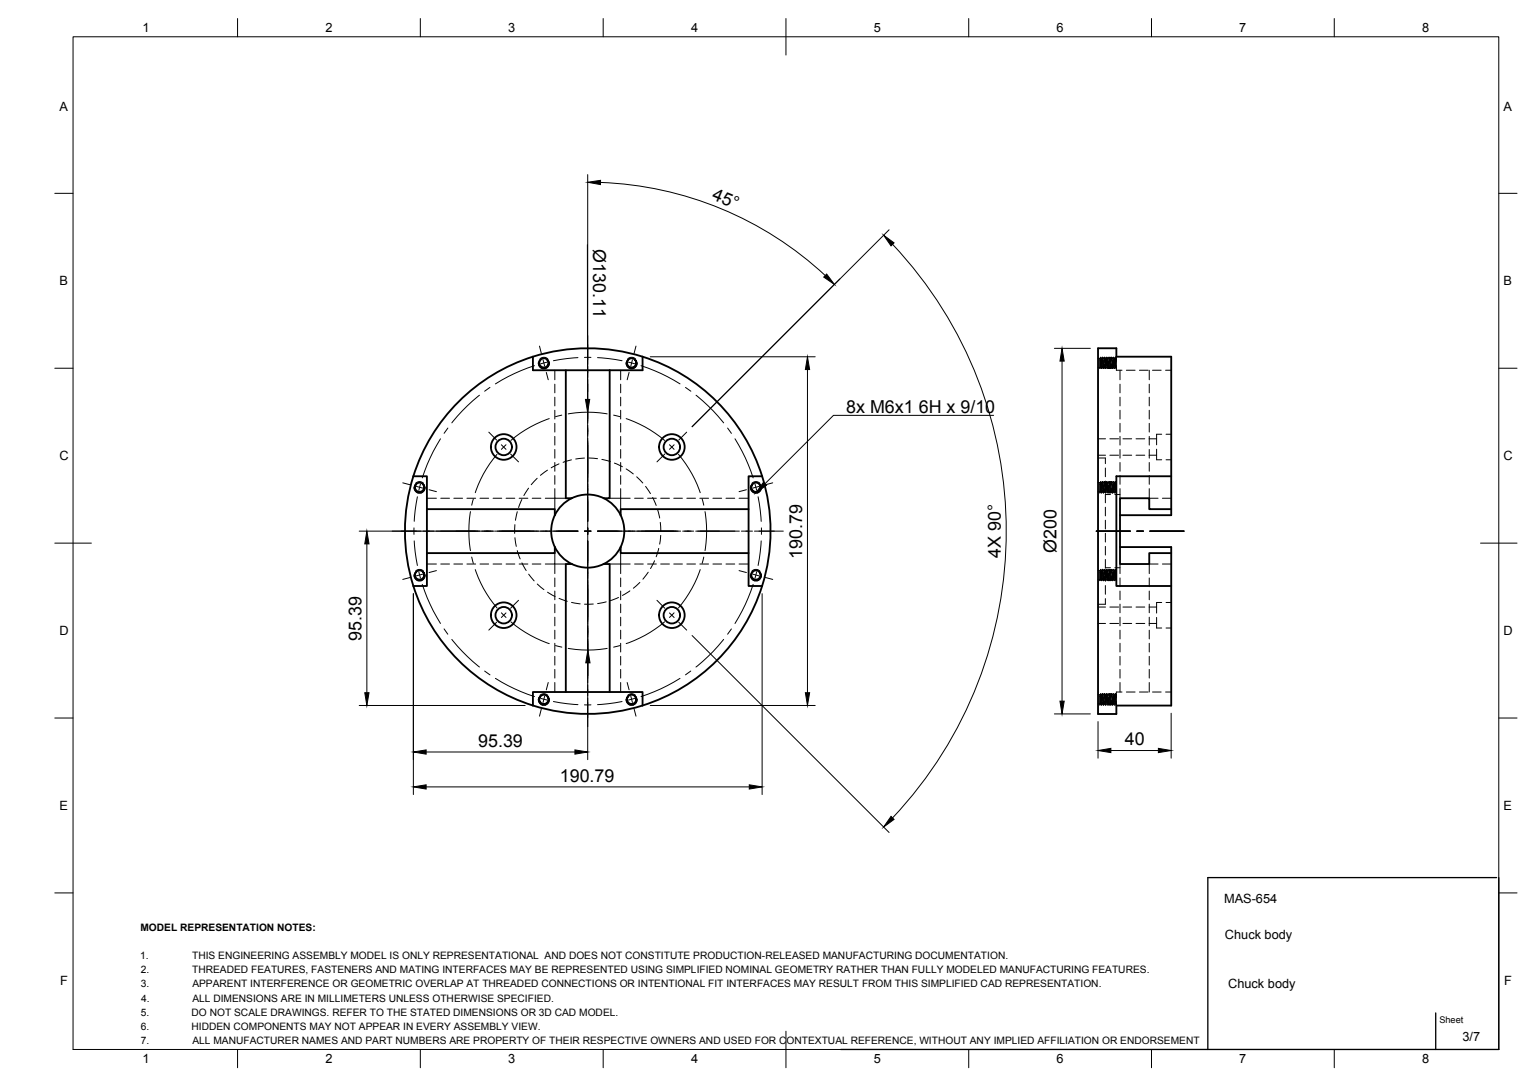
ISO-10303-21;
HEADER;
/* Generated by software containing ST-Developer
 * from STEP Tools, Inc. (www.steptools.com) 
 */

FILE_DESCRIPTION(
/* description */ ('Independent four-jaw lathe chuck,200mm body,40mm bore,36\X2\2013\X0\7
6mm nominal opposed jaw opening. Four shared machined T-jaws and model
ed partial M12x1.75 feed screws, native independent screw/slider links
, removable bolted bronze-bearing cartridges, fully captured ring/wash
er/head thrust stacks and registered bolted backplate. Custom spindle 
interface; no compatibility, speed, grip force or safety rating assign
ed.'),
/* implementation_level */ '2;1');

FILE_NAME(
/* name */ 'Chuck body.step',
/* time_stamp */ '2026-11-09T20:24:54-08:00',
/* author */ (''),
/* organization */ (''),
/* preprocessor_version */ 'ST-DEVELOPER v20.2',
/* originating_system */ 'Autodesk Translation Framework v15.17.0.0',
/* authorisation */ '');

FILE_SCHEMA (('AUTOMOTIVE_DESIGN { 1 0 10303 214 3 1 1 }'));
ENDSEC;

DATA;
#10=MECHANICAL_DESIGN_GEOMETRIC_PRESENTATION_REPRESENTATION('',(#236),#69491);
#214=SHAPE_REPRESENTATION_RELATIONSHIP('SRR','None',#69571,#225);
#225=ADVANCED_BREP_SHAPE_REPRESENTATION('',(#247),#69480);
#236=STYLED_ITEM('',(#69635),#247);
#247=MANIFOLD_SOLID_BREP('Body1',#14731);
#258=B_SPLINE_SURFACE_WITH_KNOTS('',3,3,((#24006,#24007,#24008,#24009,#24010,
#24011,#24012,#24013,#24014,#24015,#24016,#24017,#24018,#24019,#24020,#24021,
#24022,#24023,#24024,#24025,#24026,#24027,#24028,#24029,#24030,#24031,#24032,
#24033,#24034,#24035,#24036,#24037,#24038,#24039,#24040,#24041,#24042,#24043,
#24044,#24045,#24046,#24047,#24048,#24049,#24050,#24051,#24052,#24053,#24054,
#24055,#24056,#24057,#24058,#24059,#24060,#24061,#24062,#24063,#24064,#24065,
#24066,#24067),(#24068,#24069,#24070,#24071,#24072,#24073,#24074,#24075,
#24076,#24077,#24078,#24079,#24080,#24081,#24082,#24083,#24084,#24085,#24086,
#24087,#24088,#24089,#24090,#24091,#24092,#24093,#24094,#24095,#24096,#24097,
#24098,#24099,#24100,#24101,#24102,#24103,#24104,#24105,#24106,#24107,#24108,
#24109,#24110,#24111,#24112,#24113,#24114,#24115,#24116,#24117,#24118,#24119,
#24120,#24121,#24122,#24123,#24124,#24125,#24126,#24127,#24128,#24129),
(#24130,#24131,#24132,#24133,#24134,#24135,#24136,#24137,#24138,#24139,
#24140,#24141,#24142,#24143,#24144,#24145,#24146,#24147,#24148,#24149,#24150,
#24151,#24152,#24153,#24154,#24155,#24156,#24157,#24158,#24159,#24160,#24161,
#24162,#24163,#24164,#24165,#24166,#24167,#24168,#24169,#24170,#24171,#24172,
#24173,#24174,#24175,#24176,#24177,#24178,#24179,#24180,#24181,#24182,#24183,
#24184,#24185,#24186,#24187,#24188,#24189,#24190,#24191),(#24192,#24193,
#24194,#24195,#24196,#24197,#24198,#24199,#24200,#24201,#24202,#24203,#24204,
#24205,#24206,#24207,#24208,#24209,#24210,#24211,#24212,#24213,#24214,#24215,
#24216,#24217,#24218,#24219,#24220,#24221,#24222,#24223,#24224,#24225,#24226,
#24227,#24228,#24229,#24230,#24231,#24232,#24233,#24234,#24235,#24236,#24237,
#24238,#24239,#24240,#24241,#24242,#24243,#24244,#24245,#24246,#24247,#24248,
#24249,#24250,#24251,#24252,#24253)),.UNSPECIFIED.,.F.,.F.,.F.,(4,4),(4,
1,1,1,1,1,1,1,1,1,1,1,1,1,1,1,1,1,1,1,1,1,1,1,1,1,1,1,1,1,1,1,1,1,1,1,1,
1,1,1,1,1,1,1,1,1,1,1,1,1,1,1,1,1,1,1,1,1,1,4),(0.,0.0642013499338865),
(11.8589888623078,12.8516263649797,13.8442638676517,14.8369013703236,15.8295388729956,
16.8221763756675,17.8148138783395,18.8074513810114,19.8000888836834,20.7927263863553,
21.7853638890272,22.7780013916992,23.7706388943711,24.7632763970431,25.755913899715,
26.748551402387,27.7411889050589,28.7338264077309,29.7264639104028,30.7191014130747,
31.7117389157467,32.7043764184186,33.6970139210906,34.6896514237625,35.6822889264345,
36.6749264291064,37.6675639317784,38.6602014344503,39.6528389371222,40.6454764397942,
41.6381139424661,42.6307514451381,43.62338894781,44.616026450482,45.6086639531539,
46.6013014558259,47.5939389584978,48.5865764611697,49.5792139638417,50.5718514665136,
51.5644889691856,52.5571264718575,53.5497639745295,54.5424014772014,55.5350389798734,
56.5276764825453,57.5203139852172,58.5129514878892,59.5055889905611,60.4982264932331,
61.490863995905,62.483501498577,63.4761390012489,64.4687765039209,65.4614140065928,
66.4540515092648,67.4466890119367,68.4393265146086,69.4319640172806,70.4246015199525),
 .UNSPECIFIED.);
#259=B_SPLINE_SURFACE_WITH_KNOTS('',3,3,((#24370,#24371,#24372,#24373,#24374,
#24375,#24376,#24377,#24378,#24379,#24380,#24381,#24382,#24383,#24384,#24385,
#24386,#24387,#24388,#24389,#24390,#24391,#24392,#24393,#24394,#24395,#24396,
#24397,#24398,#24399,#24400,#24401,#24402,#24403,#24404,#24405,#24406,#24407,
#24408,#24409,#24410,#24411,#24412,#24413,#24414,#24415,#24416,#24417,#24418,
#24419,#24420,#24421,#24422,#24423,#24424,#24425,#24426,#24427,#24428,#24429,
#24430,#24431),(#24432,#24433,#24434,#24435,#24436,#24437,#24438,#24439,
#24440,#24441,#24442,#24443,#24444,#24445,#24446,#24447,#24448,#24449,#24450,
#24451,#24452,#24453,#24454,#24455,#24456,#24457,#24458,#24459,#24460,#24461,
#24462,#24463,#24464,#24465,#24466,#24467,#24468,#24469,#24470,#24471,#24472,
#24473,#24474,#24475,#24476,#24477,#24478,#24479,#24480,#24481,#24482,#24483,
#24484,#24485,#24486,#24487,#24488,#24489,#24490,#24491,#24492,#24493),
(#24494,#24495,#24496,#24497,#24498,#24499,#24500,#24501,#24502,#24503,
#24504,#24505,#24506,#24507,#24508,#24509,#24510,#24511,#24512,#24513,#24514,
#24515,#24516,#24517,#24518,#24519,#24520,#24521,#24522,#24523,#24524,#24525,
#24526,#24527,#24528,#24529,#24530,#24531,#24532,#24533,#24534,#24535,#24536,
#24537,#24538,#24539,#24540,#24541,#24542,#24543,#24544,#24545,#24546,#24547,
#24548,#24549,#24550,#24551,#24552,#24553,#24554,#24555),(#24556,#24557,
#24558,#24559,#24560,#24561,#24562,#24563,#24564,#24565,#24566,#24567,#24568,
#24569,#24570,#24571,#24572,#24573,#24574,#24575,#24576,#24577,#24578,#24579,
#24580,#24581,#24582,#24583,#24584,#24585,#24586,#24587,#24588,#24589,#24590,
#24591,#24592,#24593,#24594,#24595,#24596,#24597,#24598,#24599,#24600,#24601,
#24602,#24603,#24604,#24605,#24606,#24607,#24608,#24609,#24610,#24611,#24612,
#24613,#24614,#24615,#24616,#24617)),.UNSPECIFIED.,.F.,.F.,.F.,(4,4),(4,
1,1,1,1,1,1,1,1,1,1,1,1,1,1,1,1,1,1,1,1,1,1,1,1,1,1,1,1,1,1,1,1,1,1,1,1,
1,1,1,1,1,1,1,1,1,1,1,1,1,1,1,1,1,1,1,1,1,1,4),(0.,0.0642013499338865),
(14.3984001269718,15.3910376296438,16.3836751323157,17.3763126349877,18.3689501376596,
19.3615876403316,20.3542251430035,21.3468626456754,22.3395001483474,23.3321376510193,
24.3247751536913,25.3174126563632,26.3100501590352,27.3026876617071,28.2953251643791,
29.287962667051,30.2806001697229,31.2732376723949,32.2658751750668,33.2585126777388,
34.2511501804107,35.2437876830827,36.2364251857546,37.2290626884266,38.2217001910985,
39.2143376937704,40.2069751964424,41.1996126991143,42.1922502017863,43.1848877044582,
44.1775252071302,45.1701627098021,46.1628002124741,47.155437715146,48.1480752178179,
49.1407127204899,50.1333502231618,51.1259877258338,52.1186252285057,53.1112627311777,
54.1039002338496,55.0965377365216,56.0891752391935,57.0818127418655,58.0744502445374,
59.0670877472093,60.0597252498813,61.0523627525532,62.0450002552252,63.0376377578971,
64.0302752605691,65.022912763241,66.015550265913,67.0081877685849,68.0008252712568,
68.9934627739288,69.9861002766007,70.9787377792727,71.9713752819446,72.9640127846166),
 .UNSPECIFIED.);
#260=B_SPLINE_SURFACE_WITH_KNOTS('',3,3,((#24943,#24944,#24945,#24946,#24947,
#24948,#24949,#24950,#24951,#24952,#24953,#24954,#24955,#24956,#24957,#24958,
#24959,#24960,#24961,#24962,#24963,#24964,#24965,#24966,#24967,#24968,#24969,
#24970,#24971,#24972,#24973,#24974,#24975,#24976,#24977,#24978,#24979,#24980,
#24981,#24982,#24983,#24984,#24985,#24986,#24987,#24988,#24989,#24990,#24991,
#24992,#24993,#24994,#24995,#24996,#24997,#24998,#24999,#25000,#25001,#25002,
#25003,#25004),(#25005,#25006,#25007,#25008,#25009,#25010,#25011,#25012,
#25013,#25014,#25015,#25016,#25017,#25018,#25019,#25020,#25021,#25022,#25023,
#25024,#25025,#25026,#25027,#25028,#25029,#25030,#25031,#25032,#25033,#25034,
#25035,#25036,#25037,#25038,#25039,#25040,#25041,#25042,#25043,#25044,#25045,
#25046,#25047,#25048,#25049,#25050,#25051,#25052,#25053,#25054,#25055,#25056,
#25057,#25058,#25059,#25060,#25061,#25062,#25063,#25064,#25065,#25066),
(#25067,#25068,#25069,#25070,#25071,#25072,#25073,#25074,#25075,#25076,
#25077,#25078,#25079,#25080,#25081,#25082,#25083,#25084,#25085,#25086,#25087,
#25088,#25089,#25090,#25091,#25092,#25093,#25094,#25095,#25096,#25097,#25098,
#25099,#25100,#25101,#25102,#25103,#25104,#25105,#25106,#25107,#25108,#25109,
#25110,#25111,#25112,#25113,#25114,#25115,#25116,#25117,#25118,#25119,#25120,
#25121,#25122,#25123,#25124,#25125,#25126,#25127,#25128),(#25129,#25130,
#25131,#25132,#25133,#25134,#25135,#25136,#25137,#25138,#25139,#25140,#25141,
#25142,#25143,#25144,#25145,#25146,#25147,#25148,#25149,#25150,#25151,#25152,
#25153,#25154,#25155,#25156,#25157,#25158,#25159,#25160,#25161,#25162,#25163,
#25164,#25165,#25166,#25167,#25168,#25169,#25170,#25171,#25172,#25173,#25174,
#25175,#25176,#25177,#25178,#25179,#25180,#25181,#25182,#25183,#25184,#25185,
#25186,#25187,#25188,#25189,#25190)),.UNSPECIFIED.,.F.,.F.,.F.,(4,4),(4,
1,1,1,1,1,1,1,1,1,1,1,1,1,1,1,1,1,1,1,1,1,1,1,1,1,1,1,1,1,1,1,1,1,1,1,1,
1,1,1,1,1,1,1,1,1,1,1,1,1,1,1,1,1,1,1,1,1,1,4),(0.,0.0642013499338865),
(11.8589888623078,12.8516263649797,13.8442638676517,14.8369013703236,15.8295388729956,
16.8221763756675,17.8148138783395,18.8074513810114,19.8000888836834,20.7927263863553,
21.7853638890272,22.7780013916992,23.7706388943711,24.7632763970431,25.755913899715,
26.748551402387,27.7411889050589,28.7338264077309,29.7264639104028,30.7191014130747,
31.7117389157467,32.7043764184186,33.6970139210906,34.6896514237625,35.6822889264345,
36.6749264291064,37.6675639317784,38.6602014344503,39.6528389371222,40.6454764397942,
41.6381139424661,42.6307514451381,43.62338894781,44.616026450482,45.6086639531539,
46.6013014558259,47.5939389584978,48.5865764611697,49.5792139638417,50.5718514665136,
51.5644889691856,52.5571264718575,53.5497639745295,54.5424014772014,55.5350389798734,
56.5276764825453,57.5203139852172,58.5129514878892,59.5055889905611,60.4982264932331,
61.490863995905,62.483501498577,63.4761390012489,64.4687765039209,65.4614140065928,
66.4540515092647,67.4466890119367,68.4393265146086,69.4319640172806,70.4246015199525),
 .UNSPECIFIED.);
#261=B_SPLINE_SURFACE_WITH_KNOTS('',3,3,((#25307,#25308,#25309,#25310,#25311,
#25312,#25313,#25314,#25315,#25316,#25317,#25318,#25319,#25320,#25321,#25322,
#25323,#25324,#25325,#25326,#25327,#25328,#25329,#25330,#25331,#25332,#25333,
#25334,#25335,#25336,#25337,#25338,#25339,#25340,#25341,#25342,#25343,#25344,
#25345,#25346,#25347,#25348,#25349,#25350,#25351,#25352,#25353,#25354,#25355,
#25356,#25357,#25358,#25359,#25360,#25361,#25362,#25363,#25364,#25365,#25366,
#25367,#25368),(#25369,#25370,#25371,#25372,#25373,#25374,#25375,#25376,
#25377,#25378,#25379,#25380,#25381,#25382,#25383,#25384,#25385,#25386,#25387,
#25388,#25389,#25390,#25391,#25392,#25393,#25394,#25395,#25396,#25397,#25398,
#25399,#25400,#25401,#25402,#25403,#25404,#25405,#25406,#25407,#25408,#25409,
#25410,#25411,#25412,#25413,#25414,#25415,#25416,#25417,#25418,#25419,#25420,
#25421,#25422,#25423,#25424,#25425,#25426,#25427,#25428,#25429,#25430),
(#25431,#25432,#25433,#25434,#25435,#25436,#25437,#25438,#25439,#25440,
#25441,#25442,#25443,#25444,#25445,#25446,#25447,#25448,#25449,#25450,#25451,
#25452,#25453,#25454,#25455,#25456,#25457,#25458,#25459,#25460,#25461,#25462,
#25463,#25464,#25465,#25466,#25467,#25468,#25469,#25470,#25471,#25472,#25473,
#25474,#25475,#25476,#25477,#25478,#25479,#25480,#25481,#25482,#25483,#25484,
#25485,#25486,#25487,#25488,#25489,#25490,#25491,#25492),(#25493,#25494,
#25495,#25496,#25497,#25498,#25499,#25500,#25501,#25502,#25503,#25504,#25505,
#25506,#25507,#25508,#25509,#25510,#25511,#25512,#25513,#25514,#25515,#25516,
#25517,#25518,#25519,#25520,#25521,#25522,#25523,#25524,#25525,#25526,#25527,
#25528,#25529,#25530,#25531,#25532,#25533,#25534,#25535,#25536,#25537,#25538,
#25539,#25540,#25541,#25542,#25543,#25544,#25545,#25546,#25547,#25548,#25549,
#25550,#25551,#25552,#25553,#25554)),.UNSPECIFIED.,.F.,.F.,.F.,(4,4),(4,
1,1,1,1,1,1,1,1,1,1,1,1,1,1,1,1,1,1,1,1,1,1,1,1,1,1,1,1,1,1,1,1,1,1,1,1,
1,1,1,1,1,1,1,1,1,1,1,1,1,1,1,1,1,1,1,1,1,1,4),(0.,0.0642013499338865),
(14.3984001269718,15.3910376296438,16.3836751323157,17.3763126349877,18.3689501376596,
19.3615876403316,20.3542251430035,21.3468626456754,22.3395001483474,23.3321376510193,
24.3247751536913,25.3174126563632,26.3100501590352,27.3026876617071,28.2953251643791,
29.287962667051,30.280600169723,31.2732376723949,32.2658751750668,33.2585126777388,
34.2511501804107,35.2437876830827,36.2364251857546,37.2290626884266,38.2217001910985,
39.2143376937705,40.2069751964424,41.1996126991143,42.1922502017863,43.1848877044582,
44.1775252071302,45.1701627098021,46.1628002124741,47.155437715146,48.148075217818,
49.1407127204899,50.1333502231619,51.1259877258338,52.1186252285057,53.1112627311777,
54.1039002338496,55.0965377365216,56.0891752391935,57.0818127418655,58.0744502445374,
59.0670877472094,60.0597252498813,61.0523627525533,62.0450002552252,63.0376377578971,
64.0302752605691,65.022912763241,66.015550265913,67.0081877685849,68.0008252712569,
68.9934627739288,69.9861002766008,70.9787377792727,71.9713752819446,72.9640127846166),
 .UNSPECIFIED.);
#262=B_SPLINE_SURFACE_WITH_KNOTS('',3,3,((#25880,#25881,#25882,#25883,#25884,
#25885,#25886,#25887,#25888,#25889,#25890,#25891,#25892,#25893,#25894,#25895,
#25896,#25897,#25898,#25899,#25900,#25901,#25902,#25903,#25904,#25905,#25906,
#25907,#25908,#25909,#25910,#25911,#25912,#25913,#25914,#25915,#25916,#25917,
#25918,#25919,#25920,#25921,#25922,#25923,#25924,#25925,#25926,#25927,#25928,
#25929,#25930,#25931,#25932,#25933,#25934,#25935,#25936,#25937,#25938,#25939,
#25940,#25941),(#25942,#25943,#25944,#25945,#25946,#25947,#25948,#25949,
#25950,#25951,#25952,#25953,#25954,#25955,#25956,#25957,#25958,#25959,#25960,
#25961,#25962,#25963,#25964,#25965,#25966,#25967,#25968,#25969,#25970,#25971,
#25972,#25973,#25974,#25975,#25976,#25977,#25978,#25979,#25980,#25981,#25982,
#25983,#25984,#25985,#25986,#25987,#25988,#25989,#25990,#25991,#25992,#25993,
#25994,#25995,#25996,#25997,#25998,#25999,#26000,#26001,#26002,#26003),
(#26004,#26005,#26006,#26007,#26008,#26009,#26010,#26011,#26012,#26013,
#26014,#26015,#26016,#26017,#26018,#26019,#26020,#26021,#26022,#26023,#26024,
#26025,#26026,#26027,#26028,#26029,#26030,#26031,#26032,#26033,#26034,#26035,
#26036,#26037,#26038,#26039,#26040,#26041,#26042,#26043,#26044,#26045,#26046,
#26047,#26048,#26049,#26050,#26051,#26052,#26053,#26054,#26055,#26056,#26057,
#26058,#26059,#26060,#26061,#26062,#26063,#26064,#26065),(#26066,#26067,
#26068,#26069,#26070,#26071,#26072,#26073,#26074,#26075,#26076,#26077,#26078,
#26079,#26080,#26081,#26082,#26083,#26084,#26085,#26086,#26087,#26088,#26089,
#26090,#26091,#26092,#26093,#26094,#26095,#26096,#26097,#26098,#26099,#26100,
#26101,#26102,#26103,#26104,#26105,#26106,#26107,#26108,#26109,#26110,#26111,
#26112,#26113,#26114,#26115,#26116,#26117,#26118,#26119,#26120,#26121,#26122,
#26123,#26124,#26125,#26126,#26127)),.UNSPECIFIED.,.F.,.F.,.F.,(4,4),(4,
1,1,1,1,1,1,1,1,1,1,1,1,1,1,1,1,1,1,1,1,1,1,1,1,1,1,1,1,1,1,1,1,1,1,1,1,
1,1,1,1,1,1,1,1,1,1,1,1,1,1,1,1,1,1,1,1,1,1,4),(0.,0.0642013499338865),
(11.8589888623078,12.8516263649797,13.8442638676517,14.8369013703236,15.8295388729956,
16.8221763756675,17.8148138783395,18.8074513810114,19.8000888836834,20.7927263863553,
21.7853638890272,22.7780013916992,23.7706388943711,24.7632763970431,25.755913899715,
26.748551402387,27.7411889050589,28.7338264077309,29.7264639104028,30.7191014130747,
31.7117389157467,32.7043764184186,33.6970139210906,34.6896514237625,35.6822889264345,
36.6749264291064,37.6675639317784,38.6602014344503,39.6528389371222,40.6454764397942,
41.6381139424661,42.6307514451381,43.62338894781,44.616026450482,45.6086639531539,
46.6013014558259,47.5939389584978,48.5865764611697,49.5792139638417,50.5718514665136,
51.5644889691856,52.5571264718575,53.5497639745295,54.5424014772014,55.5350389798734,
56.5276764825453,57.5203139852172,58.5129514878892,59.5055889905611,60.4982264932331,
61.490863995905,62.483501498577,63.4761390012489,64.4687765039209,65.4614140065928,
66.4540515092647,67.4466890119367,68.4393265146086,69.4319640172806,70.4246015199525),
 .UNSPECIFIED.);
#263=B_SPLINE_SURFACE_WITH_KNOTS('',3,3,((#26244,#26245,#26246,#26247,#26248,
#26249,#26250,#26251,#26252,#26253,#26254,#26255,#26256,#26257,#26258,#26259,
#26260,#26261,#26262,#26263,#26264,#26265,#26266,#26267,#26268,#26269,#26270,
#26271,#26272,#26273,#26274,#26275,#26276,#26277,#26278,#26279,#26280,#26281,
#26282,#26283,#26284,#26285,#26286,#26287,#26288,#26289,#26290,#26291,#26292,
#26293,#26294,#26295,#26296,#26297,#26298,#26299,#26300,#26301,#26302,#26303,
#26304,#26305),(#26306,#26307,#26308,#26309,#26310,#26311,#26312,#26313,
#26314,#26315,#26316,#26317,#26318,#26319,#26320,#26321,#26322,#26323,#26324,
#26325,#26326,#26327,#26328,#26329,#26330,#26331,#26332,#26333,#26334,#26335,
#26336,#26337,#26338,#26339,#26340,#26341,#26342,#26343,#26344,#26345,#26346,
#26347,#26348,#26349,#26350,#26351,#26352,#26353,#26354,#26355,#26356,#26357,
#26358,#26359,#26360,#26361,#26362,#26363,#26364,#26365,#26366,#26367),
(#26368,#26369,#26370,#26371,#26372,#26373,#26374,#26375,#26376,#26377,
#26378,#26379,#26380,#26381,#26382,#26383,#26384,#26385,#26386,#26387,#26388,
#26389,#26390,#26391,#26392,#26393,#26394,#26395,#26396,#26397,#26398,#26399,
#26400,#26401,#26402,#26403,#26404,#26405,#26406,#26407,#26408,#26409,#26410,
#26411,#26412,#26413,#26414,#26415,#26416,#26417,#26418,#26419,#26420,#26421,
#26422,#26423,#26424,#26425,#26426,#26427,#26428,#26429),(#26430,#26431,
#26432,#26433,#26434,#26435,#26436,#26437,#26438,#26439,#26440,#26441,#26442,
#26443,#26444,#26445,#26446,#26447,#26448,#26449,#26450,#26451,#26452,#26453,
#26454,#26455,#26456,#26457,#26458,#26459,#26460,#26461,#26462,#26463,#26464,
#26465,#26466,#26467,#26468,#26469,#26470,#26471,#26472,#26473,#26474,#26475,
#26476,#26477,#26478,#26479,#26480,#26481,#26482,#26483,#26484,#26485,#26486,
#26487,#26488,#26489,#26490,#26491)),.UNSPECIFIED.,.F.,.F.,.F.,(4,4),(4,
1,1,1,1,1,1,1,1,1,1,1,1,1,1,1,1,1,1,1,1,1,1,1,1,1,1,1,1,1,1,1,1,1,1,1,1,
1,1,1,1,1,1,1,1,1,1,1,1,1,1,1,1,1,1,1,1,1,1,4),(0.,0.0642013499338865),
(14.3984001269718,15.3910376296438,16.3836751323157,17.3763126349877,18.3689501376596,
19.3615876403316,20.3542251430035,21.3468626456755,22.3395001483474,23.3321376510193,
24.3247751536913,25.3174126563632,26.3100501590352,27.3026876617071,28.2953251643791,
29.287962667051,30.280600169723,31.2732376723949,32.2658751750668,33.2585126777388,
34.2511501804107,35.2437876830827,36.2364251857546,37.2290626884266,38.2217001910985,
39.2143376937705,40.2069751964424,41.1996126991143,42.1922502017863,43.1848877044582,
44.1775252071302,45.1701627098021,46.1628002124741,47.155437715146,48.148075217818,
49.1407127204899,50.1333502231619,51.1259877258338,52.1186252285057,53.1112627311777,
54.1039002338496,55.0965377365216,56.0891752391935,57.0818127418655,58.0744502445374,
59.0670877472094,60.0597252498813,61.0523627525533,62.0450002552252,63.0376377578971,
64.0302752605691,65.022912763241,66.015550265913,67.0081877685849,68.0008252712569,
68.9934627739288,69.9861002766008,70.9787377792727,71.9713752819446,72.9640127846166),
 .UNSPECIFIED.);
#264=B_SPLINE_SURFACE_WITH_KNOTS('',3,3,((#26817,#26818,#26819,#26820,#26821,
#26822,#26823,#26824,#26825,#26826,#26827,#26828,#26829,#26830,#26831,#26832,
#26833,#26834,#26835,#26836,#26837,#26838,#26839,#26840,#26841,#26842,#26843,
#26844,#26845,#26846,#26847,#26848,#26849,#26850,#26851,#26852,#26853,#26854,
#26855,#26856,#26857,#26858,#26859,#26860,#26861,#26862,#26863,#26864,#26865,
#26866,#26867,#26868,#26869,#26870,#26871,#26872,#26873,#26874,#26875,#26876,
#26877,#26878),(#26879,#26880,#26881,#26882,#26883,#26884,#26885,#26886,
#26887,#26888,#26889,#26890,#26891,#26892,#26893,#26894,#26895,#26896,#26897,
#26898,#26899,#26900,#26901,#26902,#26903,#26904,#26905,#26906,#26907,#26908,
#26909,#26910,#26911,#26912,#26913,#26914,#26915,#26916,#26917,#26918,#26919,
#26920,#26921,#26922,#26923,#26924,#26925,#26926,#26927,#26928,#26929,#26930,
#26931,#26932,#26933,#26934,#26935,#26936,#26937,#26938,#26939,#26940),
(#26941,#26942,#26943,#26944,#26945,#26946,#26947,#26948,#26949,#26950,
#26951,#26952,#26953,#26954,#26955,#26956,#26957,#26958,#26959,#26960,#26961,
#26962,#26963,#26964,#26965,#26966,#26967,#26968,#26969,#26970,#26971,#26972,
#26973,#26974,#26975,#26976,#26977,#26978,#26979,#26980,#26981,#26982,#26983,
#26984,#26985,#26986,#26987,#26988,#26989,#26990,#26991,#26992,#26993,#26994,
#26995,#26996,#26997,#26998,#26999,#27000,#27001,#27002),(#27003,#27004,
#27005,#27006,#27007,#27008,#27009,#27010,#27011,#27012,#27013,#27014,#27015,
#27016,#27017,#27018,#27019,#27020,#27021,#27022,#27023,#27024,#27025,#27026,
#27027,#27028,#27029,#27030,#27031,#27032,#27033,#27034,#27035,#27036,#27037,
#27038,#27039,#27040,#27041,#27042,#27043,#27044,#27045,#27046,#27047,#27048,
#27049,#27050,#27051,#27052,#27053,#27054,#27055,#27056,#27057,#27058,#27059,
#27060,#27061,#27062,#27063,#27064)),.UNSPECIFIED.,.F.,.F.,.F.,(4,4),(4,
1,1,1,1,1,1,1,1,1,1,1,1,1,1,1,1,1,1,1,1,1,1,1,1,1,1,1,1,1,1,1,1,1,1,1,1,
1,1,1,1,1,1,1,1,1,1,1,1,1,1,1,1,1,1,1,1,1,1,4),(0.,0.0642013499338865),
(11.8589888623078,12.8516263649797,13.8442638676517,14.8369013703236,15.8295388729956,
16.8221763756675,17.8148138783395,18.8074513810114,19.8000888836834,20.7927263863553,
21.7853638890272,22.7780013916992,23.7706388943711,24.7632763970431,25.755913899715,
26.748551402387,27.7411889050589,28.7338264077309,29.7264639104028,30.7191014130747,
31.7117389157467,32.7043764184186,33.6970139210906,34.6896514237625,35.6822889264345,
36.6749264291064,37.6675639317784,38.6602014344503,39.6528389371222,40.6454764397942,
41.6381139424661,42.6307514451381,43.62338894781,44.616026450482,45.6086639531539,
46.6013014558259,47.5939389584978,48.5865764611697,49.5792139638417,50.5718514665136,
51.5644889691856,52.5571264718575,53.5497639745295,54.5424014772014,55.5350389798734,
56.5276764825453,57.5203139852172,58.5129514878892,59.5055889905611,60.4982264932331,
61.490863995905,62.483501498577,63.4761390012489,64.4687765039209,65.4614140065928,
66.4540515092647,67.4466890119367,68.4393265146086,69.4319640172806,70.4246015199525),
 .UNSPECIFIED.);
#265=B_SPLINE_SURFACE_WITH_KNOTS('',3,3,((#27181,#27182,#27183,#27184,#27185,
#27186,#27187,#27188,#27189,#27190,#27191,#27192,#27193,#27194,#27195,#27196,
#27197,#27198,#27199,#27200,#27201,#27202,#27203,#27204,#27205,#27206,#27207,
#27208,#27209,#27210,#27211,#27212,#27213,#27214,#27215,#27216,#27217,#27218,
#27219,#27220,#27221,#27222,#27223,#27224,#27225,#27226,#27227,#27228,#27229,
#27230,#27231,#27232,#27233,#27234,#27235,#27236,#27237,#27238,#27239,#27240,
#27241,#27242),(#27243,#27244,#27245,#27246,#27247,#27248,#27249,#27250,
#27251,#27252,#27253,#27254,#27255,#27256,#27257,#27258,#27259,#27260,#27261,
#27262,#27263,#27264,#27265,#27266,#27267,#27268,#27269,#27270,#27271,#27272,
#27273,#27274,#27275,#27276,#27277,#27278,#27279,#27280,#27281,#27282,#27283,
#27284,#27285,#27286,#27287,#27288,#27289,#27290,#27291,#27292,#27293,#27294,
#27295,#27296,#27297,#27298,#27299,#27300,#27301,#27302,#27303,#27304),
(#27305,#27306,#27307,#27308,#27309,#27310,#27311,#27312,#27313,#27314,
#27315,#27316,#27317,#27318,#27319,#27320,#27321,#27322,#27323,#27324,#27325,
#27326,#27327,#27328,#27329,#27330,#27331,#27332,#27333,#27334,#27335,#27336,
#27337,#27338,#27339,#27340,#27341,#27342,#27343,#27344,#27345,#27346,#27347,
#27348,#27349,#27350,#27351,#27352,#27353,#27354,#27355,#27356,#27357,#27358,
#27359,#27360,#27361,#27362,#27363,#27364,#27365,#27366),(#27367,#27368,
#27369,#27370,#27371,#27372,#27373,#27374,#27375,#27376,#27377,#27378,#27379,
#27380,#27381,#27382,#27383,#27384,#27385,#27386,#27387,#27388,#27389,#27390,
#27391,#27392,#27393,#27394,#27395,#27396,#27397,#27398,#27399,#27400,#27401,
#27402,#27403,#27404,#27405,#27406,#27407,#27408,#27409,#27410,#27411,#27412,
#27413,#27414,#27415,#27416,#27417,#27418,#27419,#27420,#27421,#27422,#27423,
#27424,#27425,#27426,#27427,#27428)),.UNSPECIFIED.,.F.,.F.,.F.,(4,4),(4,
1,1,1,1,1,1,1,1,1,1,1,1,1,1,1,1,1,1,1,1,1,1,1,1,1,1,1,1,1,1,1,1,1,1,1,1,
1,1,1,1,1,1,1,1,1,1,1,1,1,1,1,1,1,1,1,1,1,1,4),(0.,0.0642013499338865),
(14.3984001269718,15.3910376296438,16.3836751323157,17.3763126349877,18.3689501376596,
19.3615876403316,20.3542251430035,21.3468626456754,22.3395001483474,23.3321376510193,
24.3247751536913,25.3174126563632,26.3100501590352,27.3026876617071,28.2953251643791,
29.287962667051,30.2806001697229,31.2732376723949,32.2658751750668,33.2585126777388,
34.2511501804107,35.2437876830827,36.2364251857546,37.2290626884266,38.2217001910985,
39.2143376937704,40.2069751964424,41.1996126991143,42.1922502017863,43.1848877044582,
44.1775252071302,45.1701627098021,46.1628002124741,47.155437715146,48.1480752178179,
49.1407127204899,50.1333502231618,51.1259877258338,52.1186252285057,53.1112627311777,
54.1039002338496,55.0965377365216,56.0891752391935,57.0818127418654,58.0744502445374,
59.0670877472093,60.0597252498813,61.0523627525532,62.0450002552252,63.0376377578971,
64.0302752605691,65.022912763241,66.0155502659129,67.0081877685849,68.0008252712568,
68.9934627739288,69.9861002766007,70.9787377792727,71.9713752819446,72.9640127846166),
 .UNSPECIFIED.);
#266=B_SPLINE_SURFACE_WITH_KNOTS('',3,3,((#27754,#27755,#27756,#27757,#27758,
#27759,#27760,#27761,#27762,#27763,#27764,#27765,#27766,#27767,#27768,#27769,
#27770,#27771,#27772,#27773,#27774,#27775,#27776,#27777,#27778,#27779,#27780,
#27781,#27782,#27783,#27784,#27785,#27786,#27787,#27788,#27789,#27790,#27791,
#27792,#27793,#27794,#27795,#27796,#27797,#27798,#27799,#27800,#27801,#27802,
#27803,#27804,#27805,#27806,#27807,#27808,#27809,#27810,#27811,#27812,#27813,
#27814,#27815),(#27816,#27817,#27818,#27819,#27820,#27821,#27822,#27823,
#27824,#27825,#27826,#27827,#27828,#27829,#27830,#27831,#27832,#27833,#27834,
#27835,#27836,#27837,#27838,#27839,#27840,#27841,#27842,#27843,#27844,#27845,
#27846,#27847,#27848,#27849,#27850,#27851,#27852,#27853,#27854,#27855,#27856,
#27857,#27858,#27859,#27860,#27861,#27862,#27863,#27864,#27865,#27866,#27867,
#27868,#27869,#27870,#27871,#27872,#27873,#27874,#27875,#27876,#27877),
(#27878,#27879,#27880,#27881,#27882,#27883,#27884,#27885,#27886,#27887,
#27888,#27889,#27890,#27891,#27892,#27893,#27894,#27895,#27896,#27897,#27898,
#27899,#27900,#27901,#27902,#27903,#27904,#27905,#27906,#27907,#27908,#27909,
#27910,#27911,#27912,#27913,#27914,#27915,#27916,#27917,#27918,#27919,#27920,
#27921,#27922,#27923,#27924,#27925,#27926,#27927,#27928,#27929,#27930,#27931,
#27932,#27933,#27934,#27935,#27936,#27937,#27938,#27939),(#27940,#27941,
#27942,#27943,#27944,#27945,#27946,#27947,#27948,#27949,#27950,#27951,#27952,
#27953,#27954,#27955,#27956,#27957,#27958,#27959,#27960,#27961,#27962,#27963,
#27964,#27965,#27966,#27967,#27968,#27969,#27970,#27971,#27972,#27973,#27974,
#27975,#27976,#27977,#27978,#27979,#27980,#27981,#27982,#27983,#27984,#27985,
#27986,#27987,#27988,#27989,#27990,#27991,#27992,#27993,#27994,#27995,#27996,
#27997,#27998,#27999,#28000,#28001)),.UNSPECIFIED.,.F.,.F.,.F.,(4,4),(4,
1,1,1,1,1,1,1,1,1,1,1,1,1,1,1,1,1,1,1,1,1,1,1,1,1,1,1,1,1,1,1,1,1,1,1,1,
1,1,1,1,1,1,1,1,1,1,1,1,1,1,1,1,1,1,1,1,1,1,4),(0.,0.0642013499338865),
(11.8589888623078,12.8516263649797,13.8442638676517,14.8369013703236,15.8295388729956,
16.8221763756675,17.8148138783395,18.8074513810114,19.8000888836834,20.7927263863553,
21.7853638890272,22.7780013916992,23.7706388943711,24.7632763970431,25.755913899715,
26.748551402387,27.7411889050589,28.7338264077309,29.7264639104028,30.7191014130747,
31.7117389157467,32.7043764184186,33.6970139210906,34.6896514237625,35.6822889264345,
36.6749264291064,37.6675639317784,38.6602014344503,39.6528389371222,40.6454764397942,
41.6381139424661,42.6307514451381,43.62338894781,44.616026450482,45.6086639531539,
46.6013014558259,47.5939389584978,48.5865764611697,49.5792139638417,50.5718514665136,
51.5644889691856,52.5571264718575,53.5497639745295,54.5424014772014,55.5350389798734,
56.5276764825453,57.5203139852172,58.5129514878892,59.5055889905611,60.4982264932331,
61.490863995905,62.483501498577,63.4761390012489,64.4687765039209,65.4614140065928,
66.4540515092647,67.4466890119367,68.4393265146086,69.4319640172806,70.4246015199525),
 .UNSPECIFIED.);
#267=B_SPLINE_SURFACE_WITH_KNOTS('',3,3,((#28118,#28119,#28120,#28121,#28122,
#28123,#28124,#28125,#28126,#28127,#28128,#28129,#28130,#28131,#28132,#28133,
#28134,#28135,#28136,#28137,#28138,#28139,#28140,#28141,#28142,#28143,#28144,
#28145,#28146,#28147,#28148,#28149,#28150,#28151,#28152,#28153,#28154,#28155,
#28156,#28157,#28158,#28159,#28160,#28161,#28162,#28163,#28164,#28165,#28166,
#28167,#28168,#28169,#28170,#28171,#28172,#28173,#28174,#28175,#28176,#28177,
#28178,#28179),(#28180,#28181,#28182,#28183,#28184,#28185,#28186,#28187,
#28188,#28189,#28190,#28191,#28192,#28193,#28194,#28195,#28196,#28197,#28198,
#28199,#28200,#28201,#28202,#28203,#28204,#28205,#28206,#28207,#28208,#28209,
#28210,#28211,#28212,#28213,#28214,#28215,#28216,#28217,#28218,#28219,#28220,
#28221,#28222,#28223,#28224,#28225,#28226,#28227,#28228,#28229,#28230,#28231,
#28232,#28233,#28234,#28235,#28236,#28237,#28238,#28239,#28240,#28241),
(#28242,#28243,#28244,#28245,#28246,#28247,#28248,#28249,#28250,#28251,
#28252,#28253,#28254,#28255,#28256,#28257,#28258,#28259,#28260,#28261,#28262,
#28263,#28264,#28265,#28266,#28267,#28268,#28269,#28270,#28271,#28272,#28273,
#28274,#28275,#28276,#28277,#28278,#28279,#28280,#28281,#28282,#28283,#28284,
#28285,#28286,#28287,#28288,#28289,#28290,#28291,#28292,#28293,#28294,#28295,
#28296,#28297,#28298,#28299,#28300,#28301,#28302,#28303),(#28304,#28305,
#28306,#28307,#28308,#28309,#28310,#28311,#28312,#28313,#28314,#28315,#28316,
#28317,#28318,#28319,#28320,#28321,#28322,#28323,#28324,#28325,#28326,#28327,
#28328,#28329,#28330,#28331,#28332,#28333,#28334,#28335,#28336,#28337,#28338,
#28339,#28340,#28341,#28342,#28343,#28344,#28345,#28346,#28347,#28348,#28349,
#28350,#28351,#28352,#28353,#28354,#28355,#28356,#28357,#28358,#28359,#28360,
#28361,#28362,#28363,#28364,#28365)),.UNSPECIFIED.,.F.,.F.,.F.,(4,4),(4,
1,1,1,1,1,1,1,1,1,1,1,1,1,1,1,1,1,1,1,1,1,1,1,1,1,1,1,1,1,1,1,1,1,1,1,1,
1,1,1,1,1,1,1,1,1,1,1,1,1,1,1,1,1,1,1,1,1,1,4),(0.,0.0642013499338865),
(14.3984001269718,15.3910376296438,16.3836751323157,17.3763126349877,18.3689501376596,
19.3615876403316,20.3542251430035,21.3468626456754,22.3395001483474,23.3321376510193,
24.3247751536913,25.3174126563632,26.3100501590352,27.3026876617071,28.2953251643791,
29.287962667051,30.280600169723,31.2732376723949,32.2658751750668,33.2585126777388,
34.2511501804107,35.2437876830827,36.2364251857546,37.2290626884266,38.2217001910985,
39.2143376937705,40.2069751964424,41.1996126991143,42.1922502017863,43.1848877044582,
44.1775252071302,45.1701627098021,46.1628002124741,47.155437715146,48.148075217818,
49.1407127204899,50.1333502231619,51.1259877258338,52.1186252285057,53.1112627311777,
54.1039002338496,55.0965377365216,56.0891752391935,57.0818127418655,58.0744502445374,
59.0670877472094,60.0597252498813,61.0523627525533,62.0450002552252,63.0376377578971,
64.0302752605691,65.022912763241,66.015550265913,67.0081877685849,68.0008252712569,
68.9934627739288,69.9861002766008,70.9787377792727,71.9713752819446,72.9640127846166),
 .UNSPECIFIED.);
#268=B_SPLINE_SURFACE_WITH_KNOTS('',3,3,((#28691,#28692,#28693,#28694,#28695,
#28696,#28697,#28698,#28699,#28700,#28701,#28702,#28703,#28704,#28705,#28706,
#28707,#28708,#28709,#28710,#28711,#28712,#28713,#28714,#28715,#28716,#28717,
#28718,#28719,#28720,#28721,#28722,#28723,#28724,#28725,#28726,#28727,#28728,
#28729,#28730,#28731,#28732,#28733,#28734,#28735,#28736,#28737,#28738,#28739,
#28740,#28741,#28742,#28743,#28744,#28745,#28746,#28747,#28748,#28749,#28750,
#28751,#28752),(#28753,#28754,#28755,#28756,#28757,#28758,#28759,#28760,
#28761,#28762,#28763,#28764,#28765,#28766,#28767,#28768,#28769,#28770,#28771,
#28772,#28773,#28774,#28775,#28776,#28777,#28778,#28779,#28780,#28781,#28782,
#28783,#28784,#28785,#28786,#28787,#28788,#28789,#28790,#28791,#28792,#28793,
#28794,#28795,#28796,#28797,#28798,#28799,#28800,#28801,#28802,#28803,#28804,
#28805,#28806,#28807,#28808,#28809,#28810,#28811,#28812,#28813,#28814),
(#28815,#28816,#28817,#28818,#28819,#28820,#28821,#28822,#28823,#28824,
#28825,#28826,#28827,#28828,#28829,#28830,#28831,#28832,#28833,#28834,#28835,
#28836,#28837,#28838,#28839,#28840,#28841,#28842,#28843,#28844,#28845,#28846,
#28847,#28848,#28849,#28850,#28851,#28852,#28853,#28854,#28855,#28856,#28857,
#28858,#28859,#28860,#28861,#28862,#28863,#28864,#28865,#28866,#28867,#28868,
#28869,#28870,#28871,#28872,#28873,#28874,#28875,#28876),(#28877,#28878,
#28879,#28880,#28881,#28882,#28883,#28884,#28885,#28886,#28887,#28888,#28889,
#28890,#28891,#28892,#28893,#28894,#28895,#28896,#28897,#28898,#28899,#28900,
#28901,#28902,#28903,#28904,#28905,#28906,#28907,#28908,#28909,#28910,#28911,
#28912,#28913,#28914,#28915,#28916,#28917,#28918,#28919,#28920,#28921,#28922,
#28923,#28924,#28925,#28926,#28927,#28928,#28929,#28930,#28931,#28932,#28933,
#28934,#28935,#28936,#28937,#28938)),.UNSPECIFIED.,.F.,.F.,.F.,(4,4),(4,
1,1,1,1,1,1,1,1,1,1,1,1,1,1,1,1,1,1,1,1,1,1,1,1,1,1,1,1,1,1,1,1,1,1,1,1,
1,1,1,1,1,1,1,1,1,1,1,1,1,1,1,1,1,1,1,1,1,1,4),(0.,0.0642013499338865),
(11.8589888623078,12.8516263649797,13.8442638676517,14.8369013703236,15.8295388729956,
16.8221763756675,17.8148138783395,18.8074513810114,19.8000888836834,20.7927263863553,
21.7853638890272,22.7780013916992,23.7706388943711,24.7632763970431,25.755913899715,
26.748551402387,27.7411889050589,28.7338264077309,29.7264639104028,30.7191014130747,
31.7117389157467,32.7043764184186,33.6970139210906,34.6896514237625,35.6822889264345,
36.6749264291064,37.6675639317784,38.6602014344503,39.6528389371222,40.6454764397942,
41.6381139424661,42.6307514451381,43.62338894781,44.616026450482,45.6086639531539,
46.6013014558259,47.5939389584978,48.5865764611697,49.5792139638417,50.5718514665136,
51.5644889691856,52.5571264718575,53.5497639745295,54.5424014772014,55.5350389798734,
56.5276764825453,57.5203139852172,58.5129514878892,59.5055889905611,60.4982264932331,
61.490863995905,62.483501498577,63.4761390012489,64.4687765039209,65.4614140065928,
66.4540515092647,67.4466890119367,68.4393265146086,69.4319640172806,70.4246015199525),
 .UNSPECIFIED.);
#269=B_SPLINE_SURFACE_WITH_KNOTS('',3,3,((#29055,#29056,#29057,#29058,#29059,
#29060,#29061,#29062,#29063,#29064,#29065,#29066,#29067,#29068,#29069,#29070,
#29071,#29072,#29073,#29074,#29075,#29076,#29077,#29078,#29079,#29080,#29081,
#29082,#29083,#29084,#29085,#29086,#29087,#29088,#29089,#29090,#29091,#29092,
#29093,#29094,#29095,#29096,#29097,#29098,#29099,#29100,#29101,#29102,#29103,
#29104,#29105,#29106,#29107,#29108,#29109,#29110,#29111,#29112,#29113,#29114,
#29115,#29116),(#29117,#29118,#29119,#29120,#29121,#29122,#29123,#29124,
#29125,#29126,#29127,#29128,#29129,#29130,#29131,#29132,#29133,#29134,#29135,
#29136,#29137,#29138,#29139,#29140,#29141,#29142,#29143,#29144,#29145,#29146,
#29147,#29148,#29149,#29150,#29151,#29152,#29153,#29154,#29155,#29156,#29157,
#29158,#29159,#29160,#29161,#29162,#29163,#29164,#29165,#29166,#29167,#29168,
#29169,#29170,#29171,#29172,#29173,#29174,#29175,#29176,#29177,#29178),
(#29179,#29180,#29181,#29182,#29183,#29184,#29185,#29186,#29187,#29188,
#29189,#29190,#29191,#29192,#29193,#29194,#29195,#29196,#29197,#29198,#29199,
#29200,#29201,#29202,#29203,#29204,#29205,#29206,#29207,#29208,#29209,#29210,
#29211,#29212,#29213,#29214,#29215,#29216,#29217,#29218,#29219,#29220,#29221,
#29222,#29223,#29224,#29225,#29226,#29227,#29228,#29229,#29230,#29231,#29232,
#29233,#29234,#29235,#29236,#29237,#29238,#29239,#29240),(#29241,#29242,
#29243,#29244,#29245,#29246,#29247,#29248,#29249,#29250,#29251,#29252,#29253,
#29254,#29255,#29256,#29257,#29258,#29259,#29260,#29261,#29262,#29263,#29264,
#29265,#29266,#29267,#29268,#29269,#29270,#29271,#29272,#29273,#29274,#29275,
#29276,#29277,#29278,#29279,#29280,#29281,#29282,#29283,#29284,#29285,#29286,
#29287,#29288,#29289,#29290,#29291,#29292,#29293,#29294,#29295,#29296,#29297,
#29298,#29299,#29300,#29301,#29302)),.UNSPECIFIED.,.F.,.F.,.F.,(4,4),(4,
1,1,1,1,1,1,1,1,1,1,1,1,1,1,1,1,1,1,1,1,1,1,1,1,1,1,1,1,1,1,1,1,1,1,1,1,
1,1,1,1,1,1,1,1,1,1,1,1,1,1,1,1,1,1,1,1,1,1,4),(0.,0.0642013499338865),
(14.3984001269718,15.3910376296438,16.3836751323157,17.3763126349877,18.3689501376596,
19.3615876403316,20.3542251430035,21.3468626456754,22.3395001483474,23.3321376510193,
24.3247751536913,25.3174126563632,26.3100501590352,27.3026876617071,28.2953251643791,
29.287962667051,30.280600169723,31.2732376723949,32.2658751750668,33.2585126777388,
34.2511501804107,35.2437876830827,36.2364251857546,37.2290626884266,38.2217001910985,
39.2143376937705,40.2069751964424,41.1996126991143,42.1922502017863,43.1848877044582,
44.1775252071302,45.1701627098021,46.1628002124741,47.155437715146,48.148075217818,
49.1407127204899,50.1333502231619,51.1259877258338,52.1186252285057,53.1112627311777,
54.1039002338496,55.0965377365216,56.0891752391935,57.0818127418655,58.0744502445374,
59.0670877472094,60.0597252498813,61.0523627525533,62.0450002552252,63.0376377578971,
64.0302752605691,65.022912763241,66.015550265913,67.0081877685849,68.0008252712569,
68.9934627739288,69.9861002766008,70.9787377792727,71.9713752819446,72.9640127846166),
 .UNSPECIFIED.);
#270=B_SPLINE_SURFACE_WITH_KNOTS('',3,3,((#29628,#29629,#29630,#29631,#29632,
#29633,#29634,#29635,#29636,#29637,#29638,#29639,#29640,#29641,#29642,#29643,
#29644,#29645,#29646,#29647,#29648,#29649,#29650,#29651,#29652,#29653,#29654,
#29655,#29656,#29657,#29658,#29659,#29660,#29661,#29662,#29663,#29664,#29665,
#29666,#29667,#29668,#29669,#29670,#29671,#29672,#29673,#29674,#29675,#29676,
#29677,#29678,#29679,#29680,#29681,#29682,#29683,#29684,#29685,#29686,#29687,
#29688,#29689),(#29690,#29691,#29692,#29693,#29694,#29695,#29696,#29697,
#29698,#29699,#29700,#29701,#29702,#29703,#29704,#29705,#29706,#29707,#29708,
#29709,#29710,#29711,#29712,#29713,#29714,#29715,#29716,#29717,#29718,#29719,
#29720,#29721,#29722,#29723,#29724,#29725,#29726,#29727,#29728,#29729,#29730,
#29731,#29732,#29733,#29734,#29735,#29736,#29737,#29738,#29739,#29740,#29741,
#29742,#29743,#29744,#29745,#29746,#29747,#29748,#29749,#29750,#29751),
(#29752,#29753,#29754,#29755,#29756,#29757,#29758,#29759,#29760,#29761,
#29762,#29763,#29764,#29765,#29766,#29767,#29768,#29769,#29770,#29771,#29772,
#29773,#29774,#29775,#29776,#29777,#29778,#29779,#29780,#29781,#29782,#29783,
#29784,#29785,#29786,#29787,#29788,#29789,#29790,#29791,#29792,#29793,#29794,
#29795,#29796,#29797,#29798,#29799,#29800,#29801,#29802,#29803,#29804,#29805,
#29806,#29807,#29808,#29809,#29810,#29811,#29812,#29813),(#29814,#29815,
#29816,#29817,#29818,#29819,#29820,#29821,#29822,#29823,#29824,#29825,#29826,
#29827,#29828,#29829,#29830,#29831,#29832,#29833,#29834,#29835,#29836,#29837,
#29838,#29839,#29840,#29841,#29842,#29843,#29844,#29845,#29846,#29847,#29848,
#29849,#29850,#29851,#29852,#29853,#29854,#29855,#29856,#29857,#29858,#29859,
#29860,#29861,#29862,#29863,#29864,#29865,#29866,#29867,#29868,#29869,#29870,
#29871,#29872,#29873,#29874,#29875)),.UNSPECIFIED.,.F.,.F.,.F.,(4,4),(4,
1,1,1,1,1,1,1,1,1,1,1,1,1,1,1,1,1,1,1,1,1,1,1,1,1,1,1,1,1,1,1,1,1,1,1,1,
1,1,1,1,1,1,1,1,1,1,1,1,1,1,1,1,1,1,1,1,1,1,4),(0.,0.0642013499338865),
(11.8589888623078,12.8516263649797,13.8442638676517,14.8369013703236,15.8295388729956,
16.8221763756675,17.8148138783395,18.8074513810114,19.8000888836834,20.7927263863553,
21.7853638890272,22.7780013916992,23.7706388943711,24.7632763970431,25.755913899715,
26.748551402387,27.7411889050589,28.7338264077309,29.7264639104028,30.7191014130747,
31.7117389157467,32.7043764184186,33.6970139210906,34.6896514237625,35.6822889264345,
36.6749264291064,37.6675639317784,38.6602014344503,39.6528389371222,40.6454764397942,
41.6381139424661,42.6307514451381,43.62338894781,44.616026450482,45.6086639531539,
46.6013014558259,47.5939389584978,48.5865764611697,49.5792139638417,50.5718514665136,
51.5644889691856,52.5571264718575,53.5497639745295,54.5424014772014,55.5350389798734,
56.5276764825453,57.5203139852172,58.5129514878892,59.5055889905611,60.4982264932331,
61.490863995905,62.483501498577,63.4761390012489,64.4687765039209,65.4614140065928,
66.4540515092647,67.4466890119367,68.4393265146086,69.4319640172806,70.4246015199525),
 .UNSPECIFIED.);
#271=B_SPLINE_SURFACE_WITH_KNOTS('',3,3,((#29992,#29993,#29994,#29995,#29996,
#29997,#29998,#29999,#30000,#30001,#30002,#30003,#30004,#30005,#30006,#30007,
#30008,#30009,#30010,#30011,#30012,#30013,#30014,#30015,#30016,#30017,#30018,
#30019,#30020,#30021,#30022,#30023,#30024,#30025,#30026,#30027,#30028,#30029,
#30030,#30031,#30032,#30033,#30034,#30035,#30036,#30037,#30038,#30039,#30040,
#30041,#30042,#30043,#30044,#30045,#30046,#30047,#30048,#30049,#30050,#30051,
#30052,#30053),(#30054,#30055,#30056,#30057,#30058,#30059,#30060,#30061,
#30062,#30063,#30064,#30065,#30066,#30067,#30068,#30069,#30070,#30071,#30072,
#30073,#30074,#30075,#30076,#30077,#30078,#30079,#30080,#30081,#30082,#30083,
#30084,#30085,#30086,#30087,#30088,#30089,#30090,#30091,#30092,#30093,#30094,
#30095,#30096,#30097,#30098,#30099,#30100,#30101,#30102,#30103,#30104,#30105,
#30106,#30107,#30108,#30109,#30110,#30111,#30112,#30113,#30114,#30115),
(#30116,#30117,#30118,#30119,#30120,#30121,#30122,#30123,#30124,#30125,
#30126,#30127,#30128,#30129,#30130,#30131,#30132,#30133,#30134,#30135,#30136,
#30137,#30138,#30139,#30140,#30141,#30142,#30143,#30144,#30145,#30146,#30147,
#30148,#30149,#30150,#30151,#30152,#30153,#30154,#30155,#30156,#30157,#30158,
#30159,#30160,#30161,#30162,#30163,#30164,#30165,#30166,#30167,#30168,#30169,
#30170,#30171,#30172,#30173,#30174,#30175,#30176,#30177),(#30178,#30179,
#30180,#30181,#30182,#30183,#30184,#30185,#30186,#30187,#30188,#30189,#30190,
#30191,#30192,#30193,#30194,#30195,#30196,#30197,#30198,#30199,#30200,#30201,
#30202,#30203,#30204,#30205,#30206,#30207,#30208,#30209,#30210,#30211,#30212,
#30213,#30214,#30215,#30216,#30217,#30218,#30219,#30220,#30221,#30222,#30223,
#30224,#30225,#30226,#30227,#30228,#30229,#30230,#30231,#30232,#30233,#30234,
#30235,#30236,#30237,#30238,#30239)),.UNSPECIFIED.,.F.,.F.,.F.,(4,4),(4,
1,1,1,1,1,1,1,1,1,1,1,1,1,1,1,1,1,1,1,1,1,1,1,1,1,1,1,1,1,1,1,1,1,1,1,1,
1,1,1,1,1,1,1,1,1,1,1,1,1,1,1,1,1,1,1,1,1,1,4),(0.,0.0642013499338865),
(14.3984001269718,15.3910376296438,16.3836751323157,17.3763126349877,18.3689501376596,
19.3615876403316,20.3542251430035,21.3468626456754,22.3395001483474,23.3321376510193,
24.3247751536913,25.3174126563632,26.3100501590352,27.3026876617071,28.2953251643791,
29.287962667051,30.2806001697229,31.2732376723949,32.2658751750668,33.2585126777388,
34.2511501804107,35.2437876830827,36.2364251857546,37.2290626884266,38.2217001910985,
39.2143376937704,40.2069751964424,41.1996126991143,42.1922502017863,43.1848877044582,
44.1775252071302,45.1701627098021,46.1628002124741,47.155437715146,48.1480752178179,
49.1407127204899,50.1333502231618,51.1259877258338,52.1186252285057,53.1112627311777,
54.1039002338496,55.0965377365216,56.0891752391935,57.0818127418654,58.0744502445374,
59.0670877472093,60.0597252498813,61.0523627525532,62.0450002552252,63.0376377578971,
64.0302752605691,65.022912763241,66.0155502659129,67.0081877685849,68.0008252712568,
68.9934627739288,69.9861002766007,70.9787377792727,71.9713752819446,72.9640127846166),
 .UNSPECIFIED.);
#272=B_SPLINE_SURFACE_WITH_KNOTS('',3,3,((#30565,#30566,#30567,#30568,#30569,
#30570,#30571,#30572,#30573,#30574,#30575,#30576,#30577,#30578,#30579,#30580,
#30581,#30582,#30583,#30584,#30585,#30586,#30587,#30588,#30589,#30590,#30591,
#30592,#30593,#30594,#30595,#30596,#30597,#30598,#30599,#30600,#30601,#30602,
#30603,#30604,#30605,#30606,#30607,#30608,#30609,#30610,#30611,#30612,#30613,
#30614,#30615,#30616,#30617,#30618,#30619,#30620,#30621,#30622,#30623,#30624,
#30625,#30626),(#30627,#30628,#30629,#30630,#30631,#30632,#30633,#30634,
#30635,#30636,#30637,#30638,#30639,#30640,#30641,#30642,#30643,#30644,#30645,
#30646,#30647,#30648,#30649,#30650,#30651,#30652,#30653,#30654,#30655,#30656,
#30657,#30658,#30659,#30660,#30661,#30662,#30663,#30664,#30665,#30666,#30667,
#30668,#30669,#30670,#30671,#30672,#30673,#30674,#30675,#30676,#30677,#30678,
#30679,#30680,#30681,#30682,#30683,#30684,#30685,#30686,#30687,#30688),
(#30689,#30690,#30691,#30692,#30693,#30694,#30695,#30696,#30697,#30698,
#30699,#30700,#30701,#30702,#30703,#30704,#30705,#30706,#30707,#30708,#30709,
#30710,#30711,#30712,#30713,#30714,#30715,#30716,#30717,#30718,#30719,#30720,
#30721,#30722,#30723,#30724,#30725,#30726,#30727,#30728,#30729,#30730,#30731,
#30732,#30733,#30734,#30735,#30736,#30737,#30738,#30739,#30740,#30741,#30742,
#30743,#30744,#30745,#30746,#30747,#30748,#30749,#30750),(#30751,#30752,
#30753,#30754,#30755,#30756,#30757,#30758,#30759,#30760,#30761,#30762,#30763,
#30764,#30765,#30766,#30767,#30768,#30769,#30770,#30771,#30772,#30773,#30774,
#30775,#30776,#30777,#30778,#30779,#30780,#30781,#30782,#30783,#30784,#30785,
#30786,#30787,#30788,#30789,#30790,#30791,#30792,#30793,#30794,#30795,#30796,
#30797,#30798,#30799,#30800,#30801,#30802,#30803,#30804,#30805,#30806,#30807,
#30808,#30809,#30810,#30811,#30812)),.UNSPECIFIED.,.F.,.F.,.F.,(4,4),(4,
1,1,1,1,1,1,1,1,1,1,1,1,1,1,1,1,1,1,1,1,1,1,1,1,1,1,1,1,1,1,1,1,1,1,1,1,
1,1,1,1,1,1,1,1,1,1,1,1,1,1,1,1,1,1,1,1,1,1,4),(0.,0.0642013499338865),
(11.8589888623078,12.8516263649797,13.8442638676517,14.8369013703236,15.8295388729956,
16.8221763756675,17.8148138783395,18.8074513810114,19.8000888836834,20.7927263863553,
21.7853638890272,22.7780013916992,23.7706388943711,24.7632763970431,25.755913899715,
26.748551402387,27.7411889050589,28.7338264077309,29.7264639104028,30.7191014130747,
31.7117389157467,32.7043764184186,33.6970139210906,34.6896514237625,35.6822889264345,
36.6749264291064,37.6675639317784,38.6602014344503,39.6528389371222,40.6454764397942,
41.6381139424661,42.6307514451381,43.62338894781,44.616026450482,45.6086639531539,
46.6013014558259,47.5939389584978,48.5865764611697,49.5792139638417,50.5718514665136,
51.5644889691856,52.5571264718575,53.5497639745295,54.5424014772014,55.5350389798734,
56.5276764825453,57.5203139852172,58.5129514878892,59.5055889905611,60.4982264932331,
61.490863995905,62.483501498577,63.4761390012489,64.4687765039209,65.4614140065928,
66.4540515092647,67.4466890119367,68.4393265146086,69.4319640172806,70.4246015199525),
 .UNSPECIFIED.);
#273=B_SPLINE_SURFACE_WITH_KNOTS('',3,3,((#30929,#30930,#30931,#30932,#30933,
#30934,#30935,#30936,#30937,#30938,#30939,#30940,#30941,#30942,#30943,#30944,
#30945,#30946,#30947,#30948,#30949,#30950,#30951,#30952,#30953,#30954,#30955,
#30956,#30957,#30958,#30959,#30960,#30961,#30962,#30963,#30964,#30965,#30966,
#30967,#30968,#30969,#30970,#30971,#30972,#30973,#30974,#30975,#30976,#30977,
#30978,#30979,#30980,#30981,#30982,#30983,#30984,#30985,#30986,#30987,#30988,
#30989,#30990),(#30991,#30992,#30993,#30994,#30995,#30996,#30997,#30998,
#30999,#31000,#31001,#31002,#31003,#31004,#31005,#31006,#31007,#31008,#31009,
#31010,#31011,#31012,#31013,#31014,#31015,#31016,#31017,#31018,#31019,#31020,
#31021,#31022,#31023,#31024,#31025,#31026,#31027,#31028,#31029,#31030,#31031,
#31032,#31033,#31034,#31035,#31036,#31037,#31038,#31039,#31040,#31041,#31042,
#31043,#31044,#31045,#31046,#31047,#31048,#31049,#31050,#31051,#31052),
(#31053,#31054,#31055,#31056,#31057,#31058,#31059,#31060,#31061,#31062,
#31063,#31064,#31065,#31066,#31067,#31068,#31069,#31070,#31071,#31072,#31073,
#31074,#31075,#31076,#31077,#31078,#31079,#31080,#31081,#31082,#31083,#31084,
#31085,#31086,#31087,#31088,#31089,#31090,#31091,#31092,#31093,#31094,#31095,
#31096,#31097,#31098,#31099,#31100,#31101,#31102,#31103,#31104,#31105,#31106,
#31107,#31108,#31109,#31110,#31111,#31112,#31113,#31114),(#31115,#31116,
#31117,#31118,#31119,#31120,#31121,#31122,#31123,#31124,#31125,#31126,#31127,
#31128,#31129,#31130,#31131,#31132,#31133,#31134,#31135,#31136,#31137,#31138,
#31139,#31140,#31141,#31142,#31143,#31144,#31145,#31146,#31147,#31148,#31149,
#31150,#31151,#31152,#31153,#31154,#31155,#31156,#31157,#31158,#31159,#31160,
#31161,#31162,#31163,#31164,#31165,#31166,#31167,#31168,#31169,#31170,#31171,
#31172,#31173,#31174,#31175,#31176)),.UNSPECIFIED.,.F.,.F.,.F.,(4,4),(4,
1,1,1,1,1,1,1,1,1,1,1,1,1,1,1,1,1,1,1,1,1,1,1,1,1,1,1,1,1,1,1,1,1,1,1,1,
1,1,1,1,1,1,1,1,1,1,1,1,1,1,1,1,1,1,1,1,1,1,4),(0.,0.0642013499338865),
(14.3984001269718,15.3910376296438,16.3836751323157,17.3763126349877,18.3689501376596,
19.3615876403316,20.3542251430035,21.3468626456754,22.3395001483474,23.3321376510193,
24.3247751536913,25.3174126563632,26.3100501590352,27.3026876617071,28.2953251643791,
29.287962667051,30.2806001697229,31.2732376723949,32.2658751750668,33.2585126777388,
34.2511501804107,35.2437876830827,36.2364251857546,37.2290626884266,38.2217001910985,
39.2143376937704,40.2069751964424,41.1996126991143,42.1922502017863,43.1848877044582,
44.1775252071302,45.1701627098021,46.1628002124741,47.155437715146,48.1480752178179,
49.1407127204899,50.1333502231618,51.1259877258338,52.1186252285057,53.1112627311777,
54.1039002338496,55.0965377365216,56.0891752391935,57.0818127418655,58.0744502445374,
59.0670877472093,60.0597252498813,61.0523627525532,62.0450002552252,63.0376377578971,
64.0302752605691,65.022912763241,66.015550265913,67.0081877685849,68.0008252712568,
68.9934627739288,69.9861002766007,70.9787377792727,71.9713752819446,72.9640127846166),
 .UNSPECIFIED.);
#298=FACE_BOUND('',#1449,.T.);
#299=FACE_BOUND('',#1452,.T.);
#300=FACE_BOUND('',#1455,.T.);
#301=FACE_BOUND('',#1458,.T.);
#302=FACE_BOUND('',#1507,.T.);
#303=FACE_BOUND('',#1508,.T.);
#304=FACE_BOUND('',#1513,.T.);
#305=FACE_BOUND('',#1514,.T.);
#306=FACE_BOUND('',#1518,.T.);
#307=FACE_BOUND('',#1520,.T.);
#308=FACE_BOUND('',#1528,.T.);
#309=FACE_BOUND('',#1542,.T.);
#310=FACE_BOUND('',#1543,.T.);
#311=FACE_BOUND('',#1550,.T.);
#312=FACE_BOUND('',#1551,.T.);
#313=FACE_BOUND('',#1559,.T.);
#314=FACE_BOUND('',#1575,.T.);
#315=FACE_BOUND('',#1577,.T.);
#316=FACE_BOUND('',#1578,.T.);
#317=FACE_BOUND('',#1579,.T.);
#318=FACE_BOUND('',#1580,.T.);
#319=FACE_BOUND('',#1581,.T.);
#320=FACE_BOUND('',#1582,.T.);
#321=FACE_BOUND('',#1583,.T.);
#322=FACE_BOUND('',#1584,.T.);
#323=FACE_BOUND('',#1585,.T.);
#324=FACE_BOUND('',#1586,.T.);
#325=FACE_BOUND('',#1587,.T.);
#326=FACE_BOUND('',#1588,.T.);
#327=FACE_BOUND('',#1589,.T.);
#365=PLANE('',#15061);
#366=PLANE('',#15066);
#367=PLANE('',#15071);
#368=PLANE('',#15076);
#369=PLANE('',#15086);
#370=PLANE('',#15089);
#371=PLANE('',#15092);
#372=PLANE('',#15095);
#373=PLANE('',#15098);
#374=PLANE('',#15101);
#375=PLANE('',#15104);
#376=PLANE('',#15107);
#377=PLANE('',#15110);
#378=PLANE('',#15111);
#379=PLANE('',#15112);
#380=PLANE('',#15113);
#381=PLANE('',#15115);
#382=PLANE('',#15116);
#383=PLANE('',#15117);
#384=PLANE('',#15118);
#385=PLANE('',#15120);
#386=PLANE('',#15122);
#387=PLANE('',#15123);
#388=PLANE('',#15126);
#389=PLANE('',#15129);
#390=PLANE('',#15130);
#391=PLANE('',#15131);
#392=PLANE('',#15133);
#393=PLANE('',#15134);
#394=PLANE('',#15135);
#395=PLANE('',#15136);
#396=PLANE('',#15139);
#397=PLANE('',#15140);
#398=PLANE('',#15141);
#399=PLANE('',#15142);
#400=PLANE('',#15149);
#401=PLANE('',#15150);
#402=PLANE('',#15151);
#403=PLANE('',#15152);
#404=PLANE('',#15153);
#405=PLANE('',#15154);
#406=PLANE('',#15155);
#407=PLANE('',#15156);
#408=PLANE('',#15159);
#409=PLANE('',#15160);
#410=PLANE('',#15161);
#411=PLANE('',#15162);
#412=PLANE('',#15163);
#413=PLANE('',#15164);
#414=PLANE('',#15166);
#415=PLANE('',#15167);
#416=PLANE('',#15168);
#417=PLANE('',#15172);
#418=PLANE('',#15173);
#419=PLANE('',#15174);
#420=PLANE('',#15175);
#421=PLANE('',#15176);
#422=PLANE('',#15177);
#423=PLANE('',#15178);
#424=PLANE('',#15179);
#425=PLANE('',#15180);
#426=PLANE('',#15181);
#427=PLANE('',#15182);
#428=PLANE('',#15183);
#429=PLANE('',#15184);
#430=PLANE('',#15185);
#431=PLANE('',#15186);
#432=PLANE('',#15187);
#433=PLANE('',#15191);
#434=PLANE('',#15192);
#522=FACE_OUTER_BOUND('',#1303,.T.);
#523=FACE_OUTER_BOUND('',#1304,.T.);
#524=FACE_OUTER_BOUND('',#1305,.T.);
#525=FACE_OUTER_BOUND('',#1306,.T.);
#526=FACE_OUTER_BOUND('',#1307,.T.);
#527=FACE_OUTER_BOUND('',#1308,.T.);
#528=FACE_OUTER_BOUND('',#1309,.T.);
#529=FACE_OUTER_BOUND('',#1310,.T.);
#530=FACE_OUTER_BOUND('',#1311,.T.);
#531=FACE_OUTER_BOUND('',#1312,.T.);
#532=FACE_OUTER_BOUND('',#1313,.T.);
#533=FACE_OUTER_BOUND('',#1314,.T.);
#534=FACE_OUTER_BOUND('',#1315,.T.);
#535=FACE_OUTER_BOUND('',#1316,.T.);
#536=FACE_OUTER_BOUND('',#1317,.T.);
#537=FACE_OUTER_BOUND('',#1318,.T.);
#538=FACE_OUTER_BOUND('',#1319,.T.);
#539=FACE_OUTER_BOUND('',#1320,.T.);
#540=FACE_OUTER_BOUND('',#1321,.T.);
#541=FACE_OUTER_BOUND('',#1322,.T.);
#542=FACE_OUTER_BOUND('',#1323,.T.);
#543=FACE_OUTER_BOUND('',#1324,.T.);
#544=FACE_OUTER_BOUND('',#1325,.T.);
#545=FACE_OUTER_BOUND('',#1326,.T.);
#546=FACE_OUTER_BOUND('',#1327,.T.);
#547=FACE_OUTER_BOUND('',#1328,.T.);
#548=FACE_OUTER_BOUND('',#1329,.T.);
#549=FACE_OUTER_BOUND('',#1330,.T.);
#550=FACE_OUTER_BOUND('',#1331,.T.);
#551=FACE_OUTER_BOUND('',#1332,.T.);
#552=FACE_OUTER_BOUND('',#1333,.T.);
#553=FACE_OUTER_BOUND('',#1334,.T.);
#554=FACE_OUTER_BOUND('',#1335,.T.);
#555=FACE_OUTER_BOUND('',#1336,.T.);
#556=FACE_OUTER_BOUND('',#1337,.T.);
#557=FACE_OUTER_BOUND('',#1338,.T.);
#558=FACE_OUTER_BOUND('',#1339,.T.);
#559=FACE_OUTER_BOUND('',#1340,.T.);
#560=FACE_OUTER_BOUND('',#1341,.T.);
#561=FACE_OUTER_BOUND('',#1342,.T.);
#562=FACE_OUTER_BOUND('',#1343,.T.);
#563=FACE_OUTER_BOUND('',#1344,.T.);
#564=FACE_OUTER_BOUND('',#1345,.T.);
#565=FACE_OUTER_BOUND('',#1346,.T.);
#566=FACE_OUTER_BOUND('',#1347,.T.);
#567=FACE_OUTER_BOUND('',#1348,.T.);
#568=FACE_OUTER_BOUND('',#1349,.T.);
#569=FACE_OUTER_BOUND('',#1350,.T.);
#570=FACE_OUTER_BOUND('',#1351,.T.);
#571=FACE_OUTER_BOUND('',#1352,.T.);
#572=FACE_OUTER_BOUND('',#1353,.T.);
#573=FACE_OUTER_BOUND('',#1354,.T.);
#574=FACE_OUTER_BOUND('',#1355,.T.);
#575=FACE_OUTER_BOUND('',#1356,.T.);
#576=FACE_OUTER_BOUND('',#1357,.T.);
#577=FACE_OUTER_BOUND('',#1358,.T.);
#578=FACE_OUTER_BOUND('',#1359,.T.);
#579=FACE_OUTER_BOUND('',#1360,.T.);
#580=FACE_OUTER_BOUND('',#1361,.T.);
#581=FACE_OUTER_BOUND('',#1362,.T.);
#582=FACE_OUTER_BOUND('',#1363,.T.);
#583=FACE_OUTER_BOUND('',#1364,.T.);
#584=FACE_OUTER_BOUND('',#1365,.T.);
#585=FACE_OUTER_BOUND('',#1366,.T.);
#586=FACE_OUTER_BOUND('',#1367,.T.);
#587=FACE_OUTER_BOUND('',#1368,.T.);
#588=FACE_OUTER_BOUND('',#1369,.T.);
#589=FACE_OUTER_BOUND('',#1370,.T.);
#590=FACE_OUTER_BOUND('',#1371,.T.);
#591=FACE_OUTER_BOUND('',#1372,.T.);
#592=FACE_OUTER_BOUND('',#1373,.T.);
#593=FACE_OUTER_BOUND('',#1374,.T.);
#594=FACE_OUTER_BOUND('',#1375,.T.);
#595=FACE_OUTER_BOUND('',#1376,.T.);
#596=FACE_OUTER_BOUND('',#1377,.T.);
#597=FACE_OUTER_BOUND('',#1378,.T.);
#598=FACE_OUTER_BOUND('',#1379,.T.);
#599=FACE_OUTER_BOUND('',#1380,.T.);
#600=FACE_OUTER_BOUND('',#1381,.T.);
#601=FACE_OUTER_BOUND('',#1382,.T.);
#602=FACE_OUTER_BOUND('',#1383,.T.);
#603=FACE_OUTER_BOUND('',#1384,.T.);
#604=FACE_OUTER_BOUND('',#1385,.T.);
#605=FACE_OUTER_BOUND('',#1386,.T.);
#606=FACE_OUTER_BOUND('',#1387,.T.);
#607=FACE_OUTER_BOUND('',#1388,.T.);
#608=FACE_OUTER_BOUND('',#1389,.T.);
#609=FACE_OUTER_BOUND('',#1390,.T.);
#610=FACE_OUTER_BOUND('',#1391,.T.);
#611=FACE_OUTER_BOUND('',#1392,.T.);
#612=FACE_OUTER_BOUND('',#1393,.T.);
#613=FACE_OUTER_BOUND('',#1394,.T.);
#614=FACE_OUTER_BOUND('',#1395,.T.);
#615=FACE_OUTER_BOUND('',#1396,.T.);
#616=FACE_OUTER_BOUND('',#1397,.T.);
#617=FACE_OUTER_BOUND('',#1398,.T.);
#618=FACE_OUTER_BOUND('',#1399,.T.);
#619=FACE_OUTER_BOUND('',#1400,.T.);
#620=FACE_OUTER_BOUND('',#1401,.T.);
#621=FACE_OUTER_BOUND('',#1402,.T.);
#622=FACE_OUTER_BOUND('',#1403,.T.);
#623=FACE_OUTER_BOUND('',#1404,.T.);
#624=FACE_OUTER_BOUND('',#1405,.T.);
#625=FACE_OUTER_BOUND('',#1406,.T.);
#626=FACE_OUTER_BOUND('',#1407,.T.);
#627=FACE_OUTER_BOUND('',#1408,.T.);
#628=FACE_OUTER_BOUND('',#1409,.T.);
#629=FACE_OUTER_BOUND('',#1410,.T.);
#630=FACE_OUTER_BOUND('',#1411,.T.);
#631=FACE_OUTER_BOUND('',#1412,.T.);
#632=FACE_OUTER_BOUND('',#1413,.T.);
#633=FACE_OUTER_BOUND('',#1414,.T.);
#634=FACE_OUTER_BOUND('',#1415,.T.);
#635=FACE_OUTER_BOUND('',#1416,.T.);
#636=FACE_OUTER_BOUND('',#1417,.T.);
#637=FACE_OUTER_BOUND('',#1418,.T.);
#638=FACE_OUTER_BOUND('',#1419,.T.);
#639=FACE_OUTER_BOUND('',#1420,.T.);
#640=FACE_OUTER_BOUND('',#1421,.T.);
#641=FACE_OUTER_BOUND('',#1422,.T.);
#642=FACE_OUTER_BOUND('',#1423,.T.);
#643=FACE_OUTER_BOUND('',#1424,.T.);
#644=FACE_OUTER_BOUND('',#1425,.T.);
#645=FACE_OUTER_BOUND('',#1426,.T.);
#646=FACE_OUTER_BOUND('',#1427,.T.);
#647=FACE_OUTER_BOUND('',#1428,.T.);
#648=FACE_OUTER_BOUND('',#1429,.T.);
#649=FACE_OUTER_BOUND('',#1430,.T.);
#650=FACE_OUTER_BOUND('',#1431,.T.);
#651=FACE_OUTER_BOUND('',#1432,.T.);
#652=FACE_OUTER_BOUND('',#1433,.T.);
#653=FACE_OUTER_BOUND('',#1434,.T.);
#654=FACE_OUTER_BOUND('',#1435,.T.);
#655=FACE_OUTER_BOUND('',#1436,.T.);
#656=FACE_OUTER_BOUND('',#1437,.T.);
#657=FACE_OUTER_BOUND('',#1438,.T.);
#658=FACE_OUTER_BOUND('',#1439,.T.);
#659=FACE_OUTER_BOUND('',#1440,.T.);
#660=FACE_OUTER_BOUND('',#1441,.T.);
#661=FACE_OUTER_BOUND('',#1442,.T.);
#662=FACE_OUTER_BOUND('',#1443,.T.);
#663=FACE_OUTER_BOUND('',#1444,.T.);
#664=FACE_OUTER_BOUND('',#1445,.T.);
#665=FACE_OUTER_BOUND('',#1446,.T.);
#666=FACE_OUTER_BOUND('',#1447,.T.);
#667=FACE_OUTER_BOUND('',#1448,.T.);
#668=FACE_OUTER_BOUND('',#1450,.T.);
#669=FACE_OUTER_BOUND('',#1451,.T.);
#670=FACE_OUTER_BOUND('',#1453,.T.);
#671=FACE_OUTER_BOUND('',#1454,.T.);
#672=FACE_OUTER_BOUND('',#1456,.T.);
#673=FACE_OUTER_BOUND('',#1457,.T.);
#674=FACE_OUTER_BOUND('',#1459,.T.);
#675=FACE_OUTER_BOUND('',#1460,.T.);
#676=FACE_OUTER_BOUND('',#1461,.T.);
#677=FACE_OUTER_BOUND('',#1462,.T.);
#678=FACE_OUTER_BOUND('',#1463,.T.);
#679=FACE_OUTER_BOUND('',#1464,.T.);
#680=FACE_OUTER_BOUND('',#1465,.T.);
#681=FACE_OUTER_BOUND('',#1466,.T.);
#682=FACE_OUTER_BOUND('',#1467,.T.);
#683=FACE_OUTER_BOUND('',#1468,.T.);
#684=FACE_OUTER_BOUND('',#1469,.T.);
#685=FACE_OUTER_BOUND('',#1470,.T.);
#686=FACE_OUTER_BOUND('',#1471,.T.);
#687=FACE_OUTER_BOUND('',#1472,.T.);
#688=FACE_OUTER_BOUND('',#1473,.T.);
#689=FACE_OUTER_BOUND('',#1474,.T.);
#690=FACE_OUTER_BOUND('',#1475,.T.);
#691=FACE_OUTER_BOUND('',#1476,.T.);
#692=FACE_OUTER_BOUND('',#1477,.T.);
#693=FACE_OUTER_BOUND('',#1478,.T.);
#694=FACE_OUTER_BOUND('',#1479,.T.);
#695=FACE_OUTER_BOUND('',#1480,.T.);
#696=FACE_OUTER_BOUND('',#1481,.T.);
#697=FACE_OUTER_BOUND('',#1482,.T.);
#698=FACE_OUTER_BOUND('',#1483,.T.);
#699=FACE_OUTER_BOUND('',#1484,.T.);
#700=FACE_OUTER_BOUND('',#1485,.T.);
#701=FACE_OUTER_BOUND('',#1486,.T.);
#702=FACE_OUTER_BOUND('',#1487,.T.);
#703=FACE_OUTER_BOUND('',#1488,.T.);
#704=FACE_OUTER_BOUND('',#1489,.T.);
#705=FACE_OUTER_BOUND('',#1490,.T.);
#706=FACE_OUTER_BOUND('',#1491,.T.);
#707=FACE_OUTER_BOUND('',#1492,.T.);
#708=FACE_OUTER_BOUND('',#1493,.T.);
#709=FACE_OUTER_BOUND('',#1494,.T.);
#710=FACE_OUTER_BOUND('',#1495,.T.);
#711=FACE_OUTER_BOUND('',#1496,.T.);
#712=FACE_OUTER_BOUND('',#1497,.T.);
#713=FACE_OUTER_BOUND('',#1498,.T.);
#714=FACE_OUTER_BOUND('',#1499,.T.);
#715=FACE_OUTER_BOUND('',#1500,.T.);
#716=FACE_OUTER_BOUND('',#1501,.T.);
#717=FACE_OUTER_BOUND('',#1502,.T.);
#718=FACE_OUTER_BOUND('',#1503,.T.);
#719=FACE_OUTER_BOUND('',#1504,.T.);
#720=FACE_OUTER_BOUND('',#1505,.T.);
#721=FACE_OUTER_BOUND('',#1506,.T.);
#722=FACE_OUTER_BOUND('',#1509,.T.);
#723=FACE_OUTER_BOUND('',#1510,.T.);
#724=FACE_OUTER_BOUND('',#1511,.T.);
#725=FACE_OUTER_BOUND('',#1512,.T.);
#726=FACE_OUTER_BOUND('',#1515,.T.);
#727=FACE_OUTER_BOUND('',#1516,.T.);
#728=FACE_OUTER_BOUND('',#1517,.T.);
#729=FACE_OUTER_BOUND('',#1519,.T.);
#730=FACE_OUTER_BOUND('',#1521,.T.);
#731=FACE_OUTER_BOUND('',#1522,.T.);
#732=FACE_OUTER_BOUND('',#1523,.T.);
#733=FACE_OUTER_BOUND('',#1524,.T.);
#734=FACE_OUTER_BOUND('',#1525,.T.);
#735=FACE_OUTER_BOUND('',#1526,.T.);
#736=FACE_OUTER_BOUND('',#1527,.T.);
#737=FACE_OUTER_BOUND('',#1529,.T.);
#738=FACE_OUTER_BOUND('',#1530,.T.);
#739=FACE_OUTER_BOUND('',#1531,.T.);
#740=FACE_OUTER_BOUND('',#1532,.T.);
#741=FACE_OUTER_BOUND('',#1533,.T.);
#742=FACE_OUTER_BOUND('',#1534,.T.);
#743=FACE_OUTER_BOUND('',#1535,.T.);
#744=FACE_OUTER_BOUND('',#1536,.T.);
#745=FACE_OUTER_BOUND('',#1537,.T.);
#746=FACE_OUTER_BOUND('',#1538,.T.);
#747=FACE_OUTER_BOUND('',#1539,.T.);
#748=FACE_OUTER_BOUND('',#1540,.T.);
#749=FACE_OUTER_BOUND('',#1541,.T.);
#750=FACE_OUTER_BOUND('',#1544,.T.);
#751=FACE_OUTER_BOUND('',#1545,.T.);
#752=FACE_OUTER_BOUND('',#1546,.T.);
#753=FACE_OUTER_BOUND('',#1547,.T.);
#754=FACE_OUTER_BOUND('',#1548,.T.);
#755=FACE_OUTER_BOUND('',#1549,.T.);
#756=FACE_OUTER_BOUND('',#1552,.T.);
#757=FACE_OUTER_BOUND('',#1553,.T.);
#758=FACE_OUTER_BOUND('',#1554,.T.);
#759=FACE_OUTER_BOUND('',#1555,.T.);
#760=FACE_OUTER_BOUND('',#1556,.T.);
#761=FACE_OUTER_BOUND('',#1557,.T.);
#762=FACE_OUTER_BOUND('',#1558,.T.);
#763=FACE_OUTER_BOUND('',#1560,.T.);
#764=FACE_OUTER_BOUND('',#1561,.T.);
#765=FACE_OUTER_BOUND('',#1562,.T.);
#766=FACE_OUTER_BOUND('',#1563,.T.);
#767=FACE_OUTER_BOUND('',#1564,.T.);
#768=FACE_OUTER_BOUND('',#1565,.T.);
#769=FACE_OUTER_BOUND('',#1566,.T.);
#770=FACE_OUTER_BOUND('',#1567,.T.);
#771=FACE_OUTER_BOUND('',#1568,.T.);
#772=FACE_OUTER_BOUND('',#1569,.T.);
#773=FACE_OUTER_BOUND('',#1570,.T.);
#774=FACE_OUTER_BOUND('',#1571,.T.);
#775=FACE_OUTER_BOUND('',#1572,.T.);
#776=FACE_OUTER_BOUND('',#1573,.T.);
#777=FACE_OUTER_BOUND('',#1574,.T.);
#778=FACE_OUTER_BOUND('',#1576,.T.);
#1303=EDGE_LOOP('',(#8921,#8922,#8923,#8924,#8925,#8926,#8927,#8928));
#1304=EDGE_LOOP('',(#8929,#8930,#8931,#8932));
#1305=EDGE_LOOP('',(#8933,#8934,#8935,#8936));
#1306=EDGE_LOOP('',(#8937,#8938,#8939,#8940));
#1307=EDGE_LOOP('',(#8941,#8942,#8943,#8944));
#1308=EDGE_LOOP('',(#8945,#8946,#8947,#8948));
#1309=EDGE_LOOP('',(#8949,#8950,#8951,#8952));
#1310=EDGE_LOOP('',(#8953,#8954,#8955,#8956));
#1311=EDGE_LOOP('',(#8957,#8958,#8959,#8960));
#1312=EDGE_LOOP('',(#8961,#8962,#8963,#8964));
#1313=EDGE_LOOP('',(#8965,#8966,#8967,#8968));
#1314=EDGE_LOOP('',(#8969,#8970,#8971,#8972));
#1315=EDGE_LOOP('',(#8973,#8974,#8975,#8976));
#1316=EDGE_LOOP('',(#8977,#8978,#8979,#8980));
#1317=EDGE_LOOP('',(#8981,#8982,#8983,#8984));
#1318=EDGE_LOOP('',(#8985,#8986,#8987,#8988));
#1319=EDGE_LOOP('',(#8989,#8990,#8991,#8992));
#1320=EDGE_LOOP('',(#8993,#8994,#8995,#8996));
#1321=EDGE_LOOP('',(#8997,#8998,#8999,#9000,#9001,#9002,#9003,#9004));
#1322=EDGE_LOOP('',(#9005,#9006,#9007,#9008));
#1323=EDGE_LOOP('',(#9009,#9010,#9011,#9012));
#1324=EDGE_LOOP('',(#9013,#9014,#9015,#9016));
#1325=EDGE_LOOP('',(#9017,#9018,#9019,#9020));
#1326=EDGE_LOOP('',(#9021,#9022,#9023,#9024));
#1327=EDGE_LOOP('',(#9025,#9026,#9027,#9028));
#1328=EDGE_LOOP('',(#9029,#9030,#9031,#9032));
#1329=EDGE_LOOP('',(#9033,#9034,#9035,#9036));
#1330=EDGE_LOOP('',(#9037,#9038,#9039,#9040));
#1331=EDGE_LOOP('',(#9041,#9042,#9043,#9044));
#1332=EDGE_LOOP('',(#9045,#9046,#9047,#9048));
#1333=EDGE_LOOP('',(#9049,#9050,#9051,#9052));
#1334=EDGE_LOOP('',(#9053,#9054,#9055,#9056));
#1335=EDGE_LOOP('',(#9057,#9058,#9059,#9060));
#1336=EDGE_LOOP('',(#9061,#9062,#9063,#9064));
#1337=EDGE_LOOP('',(#9065,#9066,#9067,#9068));
#1338=EDGE_LOOP('',(#9069,#9070,#9071,#9072));
#1339=EDGE_LOOP('',(#9073,#9074,#9075,#9076,#9077,#9078,#9079,#9080));
#1340=EDGE_LOOP('',(#9081,#9082,#9083,#9084));
#1341=EDGE_LOOP('',(#9085,#9086,#9087,#9088));
#1342=EDGE_LOOP('',(#9089,#9090,#9091,#9092));
#1343=EDGE_LOOP('',(#9093,#9094,#9095,#9096));
#1344=EDGE_LOOP('',(#9097,#9098,#9099,#9100));
#1345=EDGE_LOOP('',(#9101,#9102,#9103,#9104));
#1346=EDGE_LOOP('',(#9105,#9106,#9107,#9108));
#1347=EDGE_LOOP('',(#9109,#9110,#9111,#9112));
#1348=EDGE_LOOP('',(#9113,#9114,#9115,#9116));
#1349=EDGE_LOOP('',(#9117,#9118,#9119,#9120));
#1350=EDGE_LOOP('',(#9121,#9122,#9123,#9124));
#1351=EDGE_LOOP('',(#9125,#9126,#9127,#9128));
#1352=EDGE_LOOP('',(#9129,#9130,#9131,#9132));
#1353=EDGE_LOOP('',(#9133,#9134,#9135,#9136));
#1354=EDGE_LOOP('',(#9137,#9138,#9139,#9140));
#1355=EDGE_LOOP('',(#9141,#9142,#9143,#9144));
#1356=EDGE_LOOP('',(#9145,#9146,#9147,#9148));
#1357=EDGE_LOOP('',(#9149,#9150,#9151,#9152,#9153,#9154,#9155,#9156));
#1358=EDGE_LOOP('',(#9157,#9158,#9159,#9160));
#1359=EDGE_LOOP('',(#9161,#9162,#9163,#9164));
#1360=EDGE_LOOP('',(#9165,#9166,#9167,#9168));
#1361=EDGE_LOOP('',(#9169,#9170,#9171,#9172));
#1362=EDGE_LOOP('',(#9173,#9174,#9175,#9176));
#1363=EDGE_LOOP('',(#9177,#9178,#9179,#9180));
#1364=EDGE_LOOP('',(#9181,#9182,#9183,#9184));
#1365=EDGE_LOOP('',(#9185,#9186,#9187,#9188));
#1366=EDGE_LOOP('',(#9189,#9190,#9191,#9192));
#1367=EDGE_LOOP('',(#9193,#9194,#9195,#9196));
#1368=EDGE_LOOP('',(#9197,#9198,#9199,#9200));
#1369=EDGE_LOOP('',(#9201,#9202,#9203,#9204));
#1370=EDGE_LOOP('',(#9205,#9206,#9207,#9208));
#1371=EDGE_LOOP('',(#9209,#9210,#9211,#9212));
#1372=EDGE_LOOP('',(#9213,#9214,#9215,#9216));
#1373=EDGE_LOOP('',(#9217,#9218,#9219,#9220));
#1374=EDGE_LOOP('',(#9221,#9222,#9223,#9224));
#1375=EDGE_LOOP('',(#9225,#9226,#9227,#9228,#9229,#9230,#9231,#9232));
#1376=EDGE_LOOP('',(#9233,#9234,#9235,#9236));
#1377=EDGE_LOOP('',(#9237,#9238,#9239,#9240));
#1378=EDGE_LOOP('',(#9241,#9242,#9243,#9244));
#1379=EDGE_LOOP('',(#9245,#9246,#9247,#9248));
#1380=EDGE_LOOP('',(#9249,#9250,#9251,#9252));
#1381=EDGE_LOOP('',(#9253,#9254,#9255,#9256));
#1382=EDGE_LOOP('',(#9257,#9258,#9259,#9260));
#1383=EDGE_LOOP('',(#9261,#9262,#9263,#9264));
#1384=EDGE_LOOP('',(#9265,#9266,#9267,#9268));
#1385=EDGE_LOOP('',(#9269,#9270,#9271,#9272));
#1386=EDGE_LOOP('',(#9273,#9274,#9275,#9276));
#1387=EDGE_LOOP('',(#9277,#9278,#9279,#9280));
#1388=EDGE_LOOP('',(#9281,#9282,#9283,#9284));
#1389=EDGE_LOOP('',(#9285,#9286,#9287,#9288));
#1390=EDGE_LOOP('',(#9289,#9290,#9291,#9292));
#1391=EDGE_LOOP('',(#9293,#9294,#9295,#9296));
#1392=EDGE_LOOP('',(#9297,#9298,#9299,#9300));
#1393=EDGE_LOOP('',(#9301,#9302,#9303,#9304,#9305,#9306,#9307,#9308));
#1394=EDGE_LOOP('',(#9309,#9310,#9311,#9312));
#1395=EDGE_LOOP('',(#9313,#9314,#9315,#9316));
#1396=EDGE_LOOP('',(#9317,#9318,#9319,#9320));
#1397=EDGE_LOOP('',(#9321,#9322,#9323,#9324));
#1398=EDGE_LOOP('',(#9325,#9326,#9327,#9328));
#1399=EDGE_LOOP('',(#9329,#9330,#9331,#9332));
#1400=EDGE_LOOP('',(#9333,#9334,#9335,#9336));
#1401=EDGE_LOOP('',(#9337,#9338,#9339,#9340));
#1402=EDGE_LOOP('',(#9341,#9342,#9343,#9344));
#1403=EDGE_LOOP('',(#9345,#9346,#9347,#9348));
#1404=EDGE_LOOP('',(#9349,#9350,#9351,#9352));
#1405=EDGE_LOOP('',(#9353,#9354,#9355,#9356));
#1406=EDGE_LOOP('',(#9357,#9358,#9359,#9360));
#1407=EDGE_LOOP('',(#9361,#9362,#9363,#9364));
#1408=EDGE_LOOP('',(#9365,#9366,#9367,#9368));
#1409=EDGE_LOOP('',(#9369,#9370,#9371,#9372));
#1410=EDGE_LOOP('',(#9373,#9374,#9375,#9376));
#1411=EDGE_LOOP('',(#9377,#9378,#9379,#9380,#9381,#9382,#9383,#9384));
#1412=EDGE_LOOP('',(#9385,#9386,#9387,#9388));
#1413=EDGE_LOOP('',(#9389,#9390,#9391,#9392));
#1414=EDGE_LOOP('',(#9393,#9394,#9395,#9396));
#1415=EDGE_LOOP('',(#9397,#9398,#9399,#9400));
#1416=EDGE_LOOP('',(#9401,#9402,#9403,#9404));
#1417=EDGE_LOOP('',(#9405,#9406,#9407,#9408));
#1418=EDGE_LOOP('',(#9409,#9410,#9411,#9412));
#1419=EDGE_LOOP('',(#9413,#9414,#9415,#9416));
#1420=EDGE_LOOP('',(#9417,#9418,#9419,#9420));
#1421=EDGE_LOOP('',(#9421,#9422,#9423,#9424));
#1422=EDGE_LOOP('',(#9425,#9426,#9427,#9428));
#1423=EDGE_LOOP('',(#9429,#9430,#9431,#9432));
#1424=EDGE_LOOP('',(#9433,#9434,#9435,#9436));
#1425=EDGE_LOOP('',(#9437,#9438,#9439,#9440));
#1426=EDGE_LOOP('',(#9441,#9442,#9443,#9444));
#1427=EDGE_LOOP('',(#9445,#9446,#9447,#9448));
#1428=EDGE_LOOP('',(#9449,#9450,#9451,#9452));
#1429=EDGE_LOOP('',(#9453,#9454,#9455,#9456,#9457,#9458,#9459,#9460));
#1430=EDGE_LOOP('',(#9461,#9462,#9463,#9464));
#1431=EDGE_LOOP('',(#9465,#9466,#9467,#9468));
#1432=EDGE_LOOP('',(#9469,#9470,#9471,#9472));
#1433=EDGE_LOOP('',(#9473,#9474,#9475,#9476));
#1434=EDGE_LOOP('',(#9477,#9478,#9479,#9480));
#1435=EDGE_LOOP('',(#9481,#9482,#9483,#9484));
#1436=EDGE_LOOP('',(#9485,#9486,#9487,#9488));
#1437=EDGE_LOOP('',(#9489,#9490,#9491,#9492));
#1438=EDGE_LOOP('',(#9493,#9494,#9495,#9496));
#1439=EDGE_LOOP('',(#9497,#9498,#9499,#9500));
#1440=EDGE_LOOP('',(#9501,#9502,#9503,#9504));
#1441=EDGE_LOOP('',(#9505,#9506,#9507,#9508));
#1442=EDGE_LOOP('',(#9509,#9510,#9511,#9512));
#1443=EDGE_LOOP('',(#9513,#9514,#9515,#9516));
#1444=EDGE_LOOP('',(#9517,#9518,#9519,#9520));
#1445=EDGE_LOOP('',(#9521,#9522,#9523,#9524));
#1446=EDGE_LOOP('',(#9525,#9526,#9527,#9528));
#1447=EDGE_LOOP('',(#9529,#9530,#9531,#9532));
#1448=EDGE_LOOP('',(#9533));
#1449=EDGE_LOOP('',(#9534));
#1450=EDGE_LOOP('',(#9535,#9536,#9537,#9538));
#1451=EDGE_LOOP('',(#9539));
#1452=EDGE_LOOP('',(#9540));
#1453=EDGE_LOOP('',(#9541,#9542,#9543,#9544));
#1454=EDGE_LOOP('',(#9545));
#1455=EDGE_LOOP('',(#9546));
#1456=EDGE_LOOP('',(#9547,#9548,#9549,#9550));
#1457=EDGE_LOOP('',(#9551));
#1458=EDGE_LOOP('',(#9552));
#1459=EDGE_LOOP('',(#9553,#9554,#9555,#9556));
#1460=EDGE_LOOP('',(#9557,#9558,#9559,#9560));
#1461=EDGE_LOOP('',(#9561,#9562,#9563,#9564));
#1462=EDGE_LOOP('',(#9565,#9566,#9567,#9568));
#1463=EDGE_LOOP('',(#9569,#9570,#9571,#9572,#9573));
#1464=EDGE_LOOP('',(#9574,#9575,#9576,#9577));
#1465=EDGE_LOOP('',(#9578,#9579,#9580,#9581,#9582,#9583,#9584,#9585,#9586,
#9587,#9588,#9589,#9590,#9591,#9592,#9593,#9594,#9595,#9596,#9597,#9598,
#9599));
#1466=EDGE_LOOP('',(#9600,#9601,#9602,#9603,#9604,#9605,#9606,#9607,#9608,
#9609,#9610,#9611,#9612,#9613,#9614,#9615,#9616,#9617,#9618,#9619,#9620,
#9621));
#1467=EDGE_LOOP('',(#9622,#9623,#9624,#9625));
#1468=EDGE_LOOP('',(#9626,#9627,#9628,#9629,#9630));
#1469=EDGE_LOOP('',(#9631,#9632,#9633,#9634));
#1470=EDGE_LOOP('',(#9635,#9636,#9637,#9638,#9639,#9640,#9641,#9642,#9643,
#9644,#9645,#9646,#9647,#9648,#9649,#9650,#9651,#9652,#9653,#9654,#9655,
#9656));
#1471=EDGE_LOOP('',(#9657,#9658,#9659,#9660,#9661,#9662,#9663,#9664,#9665,
#9666,#9667,#9668,#9669,#9670,#9671,#9672,#9673,#9674,#9675,#9676,#9677,
#9678));
#1472=EDGE_LOOP('',(#9679,#9680,#9681,#9682));
#1473=EDGE_LOOP('',(#9683,#9684,#9685,#9686,#9687));
#1474=EDGE_LOOP('',(#9688,#9689,#9690,#9691));
#1475=EDGE_LOOP('',(#9692,#9693,#9694,#9695,#9696,#9697,#9698,#9699,#9700,
#9701,#9702,#9703,#9704,#9705,#9706,#9707,#9708,#9709,#9710,#9711,#9712,
#9713));
#1476=EDGE_LOOP('',(#9714,#9715,#9716,#9717,#9718,#9719,#9720,#9721,#9722,
#9723,#9724,#9725,#9726,#9727,#9728,#9729,#9730,#9731,#9732,#9733,#9734,
#9735));
#1477=EDGE_LOOP('',(#9736,#9737,#9738,#9739));
#1478=EDGE_LOOP('',(#9740,#9741,#9742,#9743,#9744));
#1479=EDGE_LOOP('',(#9745,#9746,#9747,#9748));
#1480=EDGE_LOOP('',(#9749,#9750,#9751,#9752,#9753,#9754,#9755,#9756,#9757,
#9758,#9759,#9760,#9761,#9762,#9763,#9764,#9765,#9766,#9767,#9768,#9769,
#9770));
#1481=EDGE_LOOP('',(#9771,#9772,#9773,#9774,#9775,#9776,#9777,#9778,#9779,
#9780,#9781,#9782,#9783,#9784,#9785,#9786,#9787,#9788,#9789,#9790,#9791,
#9792));
#1482=EDGE_LOOP('',(#9793,#9794,#9795,#9796));
#1483=EDGE_LOOP('',(#9797,#9798,#9799,#9800,#9801));
#1484=EDGE_LOOP('',(#9802,#9803,#9804,#9805));
#1485=EDGE_LOOP('',(#9806,#9807,#9808,#9809,#9810,#9811,#9812,#9813,#9814,
#9815,#9816,#9817,#9818,#9819,#9820,#9821,#9822,#9823,#9824,#9825,#9826,
#9827));
#1486=EDGE_LOOP('',(#9828,#9829,#9830,#9831,#9832,#9833,#9834,#9835,#9836,
#9837,#9838,#9839,#9840,#9841,#9842,#9843,#9844,#9845,#9846,#9847,#9848,
#9849));
#1487=EDGE_LOOP('',(#9850,#9851,#9852,#9853));
#1488=EDGE_LOOP('',(#9854,#9855,#9856,#9857,#9858));
#1489=EDGE_LOOP('',(#9859,#9860,#9861,#9862));
#1490=EDGE_LOOP('',(#9863,#9864,#9865,#9866,#9867,#9868,#9869,#9870,#9871,
#9872,#9873,#9874,#9875,#9876,#9877,#9878,#9879,#9880,#9881,#9882,#9883,
#9884));
#1491=EDGE_LOOP('',(#9885,#9886,#9887,#9888,#9889,#9890,#9891,#9892,#9893,
#9894,#9895,#9896,#9897,#9898,#9899,#9900,#9901,#9902,#9903,#9904,#9905,
#9906));
#1492=EDGE_LOOP('',(#9907,#9908,#9909,#9910));
#1493=EDGE_LOOP('',(#9911,#9912,#9913,#9914,#9915));
#1494=EDGE_LOOP('',(#9916,#9917,#9918,#9919));
#1495=EDGE_LOOP('',(#9920,#9921,#9922,#9923,#9924,#9925,#9926,#9927,#9928,
#9929,#9930,#9931,#9932,#9933,#9934,#9935,#9936,#9937,#9938,#9939,#9940,
#9941));
#1496=EDGE_LOOP('',(#9942,#9943,#9944,#9945,#9946,#9947,#9948,#9949,#9950,
#9951,#9952,#9953,#9954,#9955,#9956,#9957,#9958,#9959,#9960,#9961,#9962,
#9963));
#1497=EDGE_LOOP('',(#9964,#9965,#9966,#9967));
#1498=EDGE_LOOP('',(#9968,#9969,#9970,#9971,#9972));
#1499=EDGE_LOOP('',(#9973,#9974,#9975,#9976));
#1500=EDGE_LOOP('',(#9977,#9978,#9979,#9980,#9981,#9982,#9983,#9984,#9985,
#9986,#9987,#9988,#9989,#9990,#9991,#9992,#9993,#9994,#9995,#9996,#9997,
#9998));
#1501=EDGE_LOOP('',(#9999,#10000,#10001,#10002,#10003,#10004,#10005,#10006,
#10007,#10008,#10009,#10010,#10011,#10012,#10013,#10014,#10015,#10016,#10017,
#10018,#10019,#10020));
#1502=EDGE_LOOP('',(#10021,#10022,#10023,#10024));
#1503=EDGE_LOOP('',(#10025,#10026,#10027,#10028));
#1504=EDGE_LOOP('',(#10029,#10030,#10031,#10032,#10033,#10034,#10035,#10036,
#10037,#10038,#10039,#10040));
#1505=EDGE_LOOP('',(#10041,#10042,#10043,#10044));
#1506=EDGE_LOOP('',(#10045,#10046,#10047,#10048));
#1507=EDGE_LOOP('',(#10049,#10050,#10051,#10052));
#1508=EDGE_LOOP('',(#10053,#10054,#10055,#10056));
#1509=EDGE_LOOP('',(#10057,#10058,#10059,#10060,#10061,#10062,#10063,#10064,
#10065,#10066,#10067,#10068));
#1510=EDGE_LOOP('',(#10069,#10070,#10071,#10072));
#1511=EDGE_LOOP('',(#10073,#10074,#10075,#10076));
#1512=EDGE_LOOP('',(#10077,#10078,#10079,#10080));
#1513=EDGE_LOOP('',(#10081,#10082,#10083,#10084));
#1514=EDGE_LOOP('',(#10085,#10086,#10087,#10088));
#1515=EDGE_LOOP('',(#10089,#10090,#10091,#10092,#10093,#10094));
#1516=EDGE_LOOP('',(#10095,#10096,#10097,#10098));
#1517=EDGE_LOOP('',(#10099,#10100,#10101,#10102,#10103,#10104,#10105,#10106,
#10107,#10108));
#1518=EDGE_LOOP('',(#10109));
#1519=EDGE_LOOP('',(#10110,#10111,#10112,#10113,#10114,#10115,#10116,#10117,
#10118,#10119));
#1520=EDGE_LOOP('',(#10120));
#1521=EDGE_LOOP('',(#10121,#10122,#10123,#10124));
#1522=EDGE_LOOP('',(#10125,#10126,#10127,#10128));
#1523=EDGE_LOOP('',(#10129,#10130,#10131,#10132,#10133,#10134));
#1524=EDGE_LOOP('',(#10135,#10136,#10137,#10138));
#1525=EDGE_LOOP('',(#10139,#10140,#10141,#10142));
#1526=EDGE_LOOP('',(#10143,#10144,#10145,#10146));
#1527=EDGE_LOOP('',(#10147,#10148,#10149,#10150,#10151,#10152,#10153,#10154,
#10155,#10156));
#1528=EDGE_LOOP('',(#10157));
#1529=EDGE_LOOP('',(#10158,#10159,#10160,#10161));
#1530=EDGE_LOOP('',(#10162,#10163,#10164,#10165));
#1531=EDGE_LOOP('',(#10166,#10167,#10168,#10169));
#1532=EDGE_LOOP('',(#10170,#10171,#10172,#10173));
#1533=EDGE_LOOP('',(#10174,#10175,#10176,#10177,#10178,#10179,#10180,#10181,
#10182,#10183,#10184,#10185,#10186,#10187,#10188,#10189,#10190,#10191,#10192,
#10193));
#1534=EDGE_LOOP('',(#10194,#10195,#10196,#10197,#10198,#10199));
#1535=EDGE_LOOP('',(#10200,#10201,#10202,#10203,#10204,#10205));
#1536=EDGE_LOOP('',(#10206,#10207,#10208,#10209));
#1537=EDGE_LOOP('',(#10210,#10211,#10212,#10213,#10214,#10215));
#1538=EDGE_LOOP('',(#10216,#10217,#10218,#10219,#10220,#10221));
#1539=EDGE_LOOP('',(#10222,#10223,#10224,#10225));
#1540=EDGE_LOOP('',(#10226,#10227,#10228,#10229));
#1541=EDGE_LOOP('',(#10230,#10231,#10232,#10233,#10234));
#1542=EDGE_LOOP('',(#10235,#10236,#10237,#10238));
#1543=EDGE_LOOP('',(#10239,#10240,#10241,#10242));
#1544=EDGE_LOOP('',(#10243,#10244,#10245,#10246,#10247,#10248,#10249,#10250,
#10251,#10252,#10253,#10254));
#1545=EDGE_LOOP('',(#10255,#10256,#10257,#10258));
#1546=EDGE_LOOP('',(#10259,#10260,#10261,#10262));
#1547=EDGE_LOOP('',(#10263,#10264,#10265,#10266,#10267,#10268,#10269,#10270,
#10271,#10272,#10273,#10274));
#1548=EDGE_LOOP('',(#10275,#10276,#10277,#10278));
#1549=EDGE_LOOP('',(#10279,#10280,#10281,#10282));
#1550=EDGE_LOOP('',(#10283,#10284,#10285,#10286));
#1551=EDGE_LOOP('',(#10287,#10288,#10289,#10290));
#1552=EDGE_LOOP('',(#10291,#10292,#10293,#10294));
#1553=EDGE_LOOP('',(#10295,#10296,#10297,#10298));
#1554=EDGE_LOOP('',(#10299,#10300,#10301,#10302));
#1555=EDGE_LOOP('',(#10303,#10304,#10305,#10306,#10307,#10308,#10309,#10310,
#10311,#10312,#10313,#10314,#10315,#10316,#10317,#10318,#10319,#10320,#10321,
#10322));
#1556=EDGE_LOOP('',(#10323,#10324,#10325,#10326));
#1557=EDGE_LOOP('',(#10327,#10328,#10329,#10330));
#1558=EDGE_LOOP('',(#10331,#10332,#10333,#10334,#10335,#10336,#10337,#10338,
#10339,#10340));
#1559=EDGE_LOOP('',(#10341));
#1560=EDGE_LOOP('',(#10342,#10343,#10344,#10345));
#1561=EDGE_LOOP('',(#10346,#10347,#10348,#10349,#10350,#10351));
#1562=EDGE_LOOP('',(#10352,#10353,#10354,#10355));
#1563=EDGE_LOOP('',(#10356,#10357,#10358,#10359,#10360,#10361,#10362));
#1564=EDGE_LOOP('',(#10363,#10364,#10365,#10366));
#1565=EDGE_LOOP('',(#10367,#10368,#10369,#10370));
#1566=EDGE_LOOP('',(#10371,#10372,#10373,#10374));
#1567=EDGE_LOOP('',(#10375,#10376,#10377,#10378,#10379,#10380));
#1568=EDGE_LOOP('',(#10381,#10382,#10383,#10384,#10385,#10386));
#1569=EDGE_LOOP('',(#10387,#10388,#10389,#10390));
#1570=EDGE_LOOP('',(#10391,#10392,#10393,#10394,#10395,#10396));
#1571=EDGE_LOOP('',(#10397,#10398,#10399,#10400));
#1572=EDGE_LOOP('',(#10401,#10402,#10403,#10404,#10405,#10406));
#1573=EDGE_LOOP('',(#10407,#10408,#10409,#10410));
#1574=EDGE_LOOP('',(#10411));
#1575=EDGE_LOOP('',(#10412));
#1576=EDGE_LOOP('',(#10413));
#1577=EDGE_LOOP('',(#10414));
#1578=EDGE_LOOP('',(#10415));
#1579=EDGE_LOOP('',(#10416));
#1580=EDGE_LOOP('',(#10417));
#1581=EDGE_LOOP('',(#10418));
#1582=EDGE_LOOP('',(#10419));
#1583=EDGE_LOOP('',(#10420));
#1584=EDGE_LOOP('',(#10421));
#1585=EDGE_LOOP('',(#10422));
#1586=EDGE_LOOP('',(#10423));
#1587=EDGE_LOOP('',(#10424));
#1588=EDGE_LOOP('',(#10425));
#1589=EDGE_LOOP('',(#10426));
#2151=CIRCLE('',#14867,2.5175);
#2152=CIRCLE('',#14868,2.5175);
#2153=CIRCLE('',#14869,2.5175);
#2154=CIRCLE('',#14878,2.5175);
#2155=CIRCLE('',#14880,3.07349999999999);
#2156=CIRCLE('',#14889,3.0735);
#2157=CIRCLE('',#14891,2.5175);
#2158=CIRCLE('',#14892,2.5175);
#2159=CIRCLE('',#14893,2.5175);
#2160=CIRCLE('',#14902,2.5175);
#2161=CIRCLE('',#14904,3.07349999999999);
#2162=CIRCLE('',#14913,3.0735);
#2163=CIRCLE('',#14915,2.5175);
#2164=CIRCLE('',#14916,2.5175);
#2165=CIRCLE('',#14917,2.5175);
#2166=CIRCLE('',#14926,2.5175);
#2167=CIRCLE('',#14928,3.0735);
#2168=CIRCLE('',#14937,3.0735);
#2169=CIRCLE('',#14939,2.5175);
#2170=CIRCLE('',#14940,2.5175);
#2171=CIRCLE('',#14941,2.5175);
#2172=CIRCLE('',#14950,2.5175);
#2173=CIRCLE('',#14952,3.0735);
#2174=CIRCLE('',#14961,3.0735);
#2175=CIRCLE('',#14963,2.5175);
#2176=CIRCLE('',#14964,2.5175);
#2177=CIRCLE('',#14965,2.5175);
#2178=CIRCLE('',#14974,2.5175);
#2179=CIRCLE('',#14976,3.07349999999999);
#2180=CIRCLE('',#14985,3.0735);
#2181=CIRCLE('',#14987,2.5175);
#2182=CIRCLE('',#14988,2.5175);
#2183=CIRCLE('',#14989,2.5175);
#2184=CIRCLE('',#14998,2.5175);
#2185=CIRCLE('',#15000,3.0735);
#2186=CIRCLE('',#15009,3.0735);
#2187=CIRCLE('',#15011,2.5175);
#2188=CIRCLE('',#15012,2.5175);
#2189=CIRCLE('',#15013,2.5175);
#2190=CIRCLE('',#15022,2.5175);
#2191=CIRCLE('',#15024,3.0735);
#2192=CIRCLE('',#15033,3.0735);
#2193=CIRCLE('',#15035,2.5175);
#2194=CIRCLE('',#15036,2.5175);
#2195=CIRCLE('',#15037,2.5175);
#2196=CIRCLE('',#15046,2.5175);
#2197=CIRCLE('',#15048,3.07349999999999);
#2198=CIRCLE('',#15057,3.0735);
#2199=CIRCLE('',#15059,7.);
#2200=CIRCLE('',#15060,7.);
#2201=CIRCLE('',#15062,4.5);
#2202=CIRCLE('',#15064,7.);
#2203=CIRCLE('',#15065,7.);
#2204=CIRCLE('',#15067,4.5);
#2205=CIRCLE('',#15069,7.);
#2206=CIRCLE('',#15070,7.);
#2207=CIRCLE('',#15072,4.5);
#2208=CIRCLE('',#15074,7.);
#2209=CIRCLE('',#15075,7.);
#2210=CIRCLE('',#15077,4.5);
#2211=CIRCLE('',#15079,4.5);
#2212=CIRCLE('',#15081,4.5);
#2213=CIRCLE('',#15083,4.5);
#2214=CIRCLE('',#15085,4.5);
#2215=CIRCLE('',#15114,100.);
#2216=CIRCLE('',#15119,100.);
#2217=CIRCLE('',#15121,20.);
#2218=CIRCLE('',#15124,100.);
#2219=CIRCLE('',#15125,20.);
#2220=CIRCLE('',#15127,20.);
#2221=CIRCLE('',#15128,100.);
#2222=CIRCLE('',#15132,20.);
#2223=CIRCLE('',#15137,100.);
#2224=CIRCLE('',#15138,20.);
#2225=CIRCLE('',#15144,20.);
#2226=CIRCLE('',#15145,20.);
#2227=CIRCLE('',#15146,20.);
#2228=CIRCLE('',#15147,20.);
#2229=CIRCLE('',#15148,20.);
#2230=CIRCLE('',#15157,100.);
#2231=CIRCLE('',#15158,100.);
#2232=CIRCLE('',#15165,100.);
#2233=CIRCLE('',#15170,100.);
#2234=CIRCLE('',#15171,100.);
#2235=CIRCLE('',#15189,40.);
#2236=CIRCLE('',#15190,40.);
#2347=B_SPLINE_CURVE_WITH_KNOTS('',3,(#18716,#18717,#18718,#18719),
 .UNSPECIFIED.,.F.,.F.,(4,4),(57.8582309055934,58.5656126576447),
 .UNSPECIFIED.);
#2348=B_SPLINE_CURVE_WITH_KNOTS('',3,(#18727,#18728,#18729,#18730,#18731,
#18732,#18733,#18734,#18735,#18736),.UNSPECIFIED.,.F.,.F.,(4,3,3,4),(-56.5486677646163,
-55.5877001496289,-54.595062646957,-54.1144568630778),.UNSPECIFIED.);
#2349=B_SPLINE_CURVE_WITH_KNOTS('',3,(#18741,#18742,#18743,#18744,#18745,
#18746,#18747,#18748,#18749,#18750,#18751,#18752,#18753,#18754,#18755,#18756,
#18757,#18758,#18759,#18760,#18761,#18762,#18763,#18764,#18765),
 .UNSPECIFIED.,.F.,.F.,(4,3,3,3,3,3,3,3,4),(51.5750455984138,51.6171501389411,
52.6097876416131,53.602425144285,54.595062646957,55.5877001496289,56.5803376523009,
57.5729751549728,57.8582309055934),.UNSPECIFIED.);
#2350=B_SPLINE_CURVE_WITH_KNOTS('',3,(#18766,#18767,#18768,#18769,#18770,
#18771,#18772,#18773,#18774,#18775,#18776,#18777,#18778,#18779,#18780,#18781,
#18782,#18783,#18784,#18785,#18786,#18787),.UNSPECIFIED.,.F.,.F.,(4,3,3,
3,3,3,3,4),(-54.1144568630778,-53.602425144285,-52.6097876416131,-51.6171501389411,
-50.6245126362692,-49.6318751335972,-48.6392376309253,-47.8312715558982),
 .UNSPECIFIED.);
#2351=B_SPLINE_CURVE_WITH_KNOTS('',3,(#18792,#18793,#18794,#18795,#18796,
#18797,#18798,#18799,#18800,#18801,#18802,#18803,#18804,#18805,#18806,#18807,
#18808,#18809,#18810,#18811,#18812,#18813),.UNSPECIFIED.,.F.,.F.,(4,3,3,
3,3,3,3,4),(45.2918602912342,45.6613251229095,46.6539626255814,47.6466001282533,
48.6392376309253,49.6318751335972,50.6245126362692,51.5750455984138),
 .UNSPECIFIED.);
#2352=B_SPLINE_CURVE_WITH_KNOTS('',3,(#18814,#18815,#18816,#18817,#18818,
#18819,#18820,#18821,#18822,#18823,#18824,#18825,#18826,#18827,#18828,#18829,
#18830,#18831,#18832,#18833,#18834,#18835,#18836,#18837,#18838),
 .UNSPECIFIED.,.F.,.F.,(4,3,3,3,3,3,3,3,4),(-47.8312715558982,-47.6466001282533,
-46.6539626255814,-45.6613251229095,-44.6686876202375,-43.6760501175656,
-42.6834126148936,-41.6907751122217,-41.5480862487187),.UNSPECIFIED.);
#2353=B_SPLINE_CURVE_WITH_KNOTS('',3,(#18843,#18844,#18845,#18846,#18847,
#18848,#18849,#18850,#18851,#18852,#18853,#18854,#18855,#18856,#18857,#18858,
#18859,#18860,#18861,#18862,#18863,#18864),.UNSPECIFIED.,.F.,.F.,(4,3,3,
3,3,3,3,4),(39.0086749840546,39.7055001068778,40.6981376095497,41.6907751122217,
42.6834126148936,43.6760501175656,44.6686876202375,45.2918602912342),
 .UNSPECIFIED.);
#2354=B_SPLINE_CURVE_WITH_KNOTS('',3,(#18865,#18866,#18867,#18868,#18869,
#18870,#18871,#18872,#18873,#18874,#18875,#18876,#18877,#18878,#18879,#18880,
#18881,#18882,#18883,#18884,#18885,#18886),.UNSPECIFIED.,.F.,.F.,(4,3,3,
3,3,3,3,4),(-41.5480862487187,-40.6981376095497,-39.7055001068778,-38.7128626042058,
-37.7202251015339,-36.727587598862,-35.73495009619,-35.2649009415391),
 .UNSPECIFIED.);
#2355=B_SPLINE_CURVE_WITH_KNOTS('',3,(#18891,#18892,#18893,#18894,#18895,
#18896,#18897,#18898,#18899,#18900,#18901,#18902,#18903,#18904,#18905,#18906,
#18907,#18908,#18909,#18910,#18911,#18912,#18913,#18914,#18915),
 .UNSPECIFIED.,.F.,.F.,(4,3,3,3,3,3,3,3,4),(32.725489676875,32.7570375881742,
33.7496750908461,34.7423125935181,35.73495009619,36.727587598862,37.7202251015339,
38.7128626042058,39.0086749840546),.UNSPECIFIED.);
#2356=B_SPLINE_CURVE_WITH_KNOTS('',3,(#18916,#18917,#18918,#18919,#18920,
#18921,#18922,#18923,#18924,#18925,#18926,#18927,#18928,#18929,#18930,#18931,
#18932,#18933,#18934,#18935,#18936,#18937),.UNSPECIFIED.,.F.,.F.,(4,3,3,
3,3,3,3,4),(-35.2649009415391,-34.7423125935181,-33.7496750908461,-32.7570375881742,
-31.7644000855022,-30.7717625828303,-29.7791250801584,-28.9817156343595),
 .UNSPECIFIED.);
#2357=B_SPLINE_CURVE_WITH_KNOTS('',3,(#18942,#18943,#18944,#18945,#18946,
#18947,#18948,#18949,#18950,#18951,#18952,#18953,#18954,#18955,#18956,#18957,
#18958,#18959,#18960,#18961,#18962,#18963),.UNSPECIFIED.,.F.,.F.,(4,3,3,
3,3,3,3,4),(26.4423043696954,26.8012125721425,27.7938500748145,28.7864875774864,
29.7791250801583,30.7717625828303,31.7644000855022,32.725489676875),
 .UNSPECIFIED.);
#2358=B_SPLINE_CURVE_WITH_KNOTS('',3,(#18964,#18965,#18966,#18967,#18968,
#18969,#18970,#18971,#18972,#18973,#18974,#18975,#18976,#18977,#18978,#18979,
#18980,#18981,#18982,#18983,#18984,#18985,#18986,#18987,#18988),
 .UNSPECIFIED.,.F.,.F.,(4,3,3,3,3,3,3,3,4),(-28.9817156343595,-28.7864875774864,
-27.7938500748145,-26.8012125721425,-25.8085750694706,-24.8159375667986,
-23.8233000641267,-22.8306625614547,-22.6985303271799),.UNSPECIFIED.);
#2359=B_SPLINE_CURVE_WITH_KNOTS('',3,(#18993,#18994,#18995,#18996,#18997,
#18998,#18999,#19000,#19001,#19002,#19003,#19004,#19005,#19006,#19007,#19008,
#19009,#19010,#19011,#19012,#19013,#19014),.UNSPECIFIED.,.F.,.F.,(4,3,3,
3,3,3,3,4),(20.1591190625158,20.8453875561108,21.8380250587828,22.8306625614547,
23.8233000641267,24.8159375667986,25.8085750694706,26.4423043696954),
 .UNSPECIFIED.);
#2360=B_SPLINE_CURVE_WITH_KNOTS('',3,(#19015,#19016,#19017,#19018,#19019,
#19020,#19021,#19022,#19023,#19024,#19025,#19026,#19027,#19028,#19029,#19030,
#19031,#19032,#19033,#19034,#19035,#19036),.UNSPECIFIED.,.F.,.F.,(4,3,3,
3,3,3,3,4),(-22.6985303271799,-21.8380250587828,-20.8453875561108,-19.8527500534389,
-18.8601125507669,-17.867475048095,-16.8748375454231,-16.4153450200003),
 .UNSPECIFIED.);
#2361=B_SPLINE_CURVE_WITH_KNOTS('',3,(#19041,#19042,#19043,#19044,#19045,
#19046,#19047,#19048,#19049,#19050,#19051,#19052,#19053,#19054,#19055,#19056,
#19057,#19058,#19059,#19060,#19061,#19062,#19063,#19064,#19065),
 .UNSPECIFIED.,.F.,.F.,(4,3,3,3,3,3,3,3,4),(13.8759337553362,13.8969250374072,
14.8895625400792,15.8822000427511,16.8748375454231,17.867475048095,18.860112550767,
19.8527500534389,20.1591190625158),.UNSPECIFIED.);
#2362=B_SPLINE_CURVE_WITH_KNOTS('',3,(#19066,#19067,#19068,#19069,#19070,
#19071,#19072,#19073,#19074,#19075,#19076,#19077,#19078,#19079,#19080,#19081,
#19082,#19083,#19084,#19085,#19086,#19087),.UNSPECIFIED.,.F.,.F.,(4,3,3,
3,3,3,3,4),(-16.4153450200003,-15.8822000427511,-14.8895625400792,-13.8969250374072,
-12.9042875347353,-11.9116500320633,-10.9190125293914,-10.1321597128207),
 .UNSPECIFIED.);
#2363=B_SPLINE_CURVE_WITH_KNOTS('',3,(#19093,#19094,#19095,#19096,#19097,
#19098,#19099,#19100,#19101,#19102,#19103,#19104,#19105),.UNSPECIFIED.,
 .F.,.F.,(4,3,3,3,4),(-3.84897440564114,-2.97791250801584,-1.98527500534389,
-0.992637502671947,0.),.UNSPECIFIED.);
#2364=B_SPLINE_CURVE_WITH_KNOTS('',3,(#19108,#19109,#19110,#19111,#19112,
#19113,#19114,#19115,#19116,#19117,#19118,#19119,#19120,#19121,#19122,#19123,
#19124,#19125,#19126),.UNSPECIFIED.,.F.,.F.,(4,3,3,3,3,3,4),(2.01694489302841,
2.97791250801583,3.97055001068778,4.96318751335972,5.95582501603167,6.94846251870361,
7.59274844815666),.UNSPECIFIED.);
#2365=B_SPLINE_CURVE_WITH_KNOTS('',3,(#19132,#19133,#19134,#19135,#19136,
#19137,#19138,#19139),.UNSPECIFIED.,.F.,.F.,(4,1,1,1,1,4),(65.9734457253856,
66.4540515092647,67.4466890119367,68.4393265146086,69.4319640172806,70.4246015199525),
 .UNSPECIFIED.);
#2366=B_SPLINE_CURVE_WITH_KNOTS('',3,(#19142,#19143,#19144,#19145,#19146,
#19147,#19148,#19149,#19150),.UNSPECIFIED.,.F.,.F.,(4,1,1,1,1,1,4),(65.9734457253856,
66.015550265913,67.0081877685849,68.0008252712568,68.9934627739288,69.9861002766007,
70.9470678915881),.UNSPECIFIED.);
#2367=B_SPLINE_CURVE_WITH_KNOTS('',3,(#19155,#19156,#19157,#19158,#19159,
#19160,#19161,#19162,#19163,#19164),.UNSPECIFIED.,.F.,.F.,(4,1,1,1,1,1,
1,4),(59.6902604182061,60.4982264932331,61.490863995905,62.483501498577,
63.4761390012489,64.4687765039209,65.4614140065928,65.9734457253856),
 .UNSPECIFIED.);
#2368=B_SPLINE_CURVE_WITH_KNOTS('',3,(#19165,#19166,#19167,#19168,#19169,
#19170,#19171,#19172,#19173,#19174),.UNSPECIFIED.,.F.,.F.,(4,1,1,1,1,1,
1,4),(59.6902604182061,60.0597252498813,61.0523627525532,62.0450002552252,
63.0376377578971,64.0302752605691,65.022912763241,65.9734457253856),
 .UNSPECIFIED.);
#2369=B_SPLINE_CURVE_WITH_KNOTS('',3,(#19179,#19180,#19181,#19182,#19183,
#19184,#19185,#19186,#19187,#19188,#19189),.UNSPECIFIED.,.F.,.F.,(4,1,1,
1,1,1,1,1,4),(53.4070751110265,53.5497639745295,54.5424014772014,55.5350389798734,
56.5276764825453,57.5203139852172,58.5129514878892,59.5055889905611,59.6902604182061),
 .UNSPECIFIED.);
#2370=B_SPLINE_CURVE_WITH_KNOTS('',3,(#19190,#19191,#19192,#19193,#19194,
#19195,#19196,#19197,#19198,#19199),.UNSPECIFIED.,.F.,.F.,(4,1,1,1,1,1,
1,4),(53.4070751110265,54.1039002338496,55.0965377365216,56.0891752391935,
57.0818127418655,58.0744502445374,59.0670877472093,59.6902604182061),
 .UNSPECIFIED.);
#2371=B_SPLINE_CURVE_WITH_KNOTS('',3,(#19204,#19205,#19206,#19207,#19208,
#19209,#19210,#19211,#19212,#19213),.UNSPECIFIED.,.F.,.F.,(4,1,1,1,1,1,
1,4),(47.1238898038469,47.5939389584978,48.5865764611697,49.5792139638417,
50.5718514665136,51.5644889691856,52.5571264718575,53.4070751110265),
 .UNSPECIFIED.);
#2372=B_SPLINE_CURVE_WITH_KNOTS('',3,(#19214,#19215,#19216,#19217,#19218,
#19219,#19220,#19221,#19222,#19223,#19224),.UNSPECIFIED.,.F.,.F.,(4,1,1,
1,1,1,1,1,4),(47.1238898038469,47.155437715146,48.1480752178179,49.1407127204899,
50.1333502231618,51.1259877258338,52.1186252285057,53.1112627311777,53.4070751110265),
 .UNSPECIFIED.);
#2373=B_SPLINE_CURVE_WITH_KNOTS('',3,(#19229,#19230,#19231,#19232,#19233,
#19234,#19235,#19236,#19237,#19238),.UNSPECIFIED.,.F.,.F.,(4,1,1,1,1,1,
1,4),(40.8407044966673,41.6381139424661,42.6307514451381,43.62338894781,
44.616026450482,45.6086639531539,46.6013014558259,47.1238898038469),
 .UNSPECIFIED.);
#2374=B_SPLINE_CURVE_WITH_KNOTS('',3,(#19239,#19240,#19241,#19242,#19243,
#19244,#19245,#19246,#19247,#19248),.UNSPECIFIED.,.F.,.F.,(4,1,1,1,1,1,
1,4),(40.8407044966673,41.1996126991143,42.1922502017863,43.1848877044582,
44.1775252071302,45.1701627098021,46.1628002124741,47.1238898038469),
 .UNSPECIFIED.);
#2375=B_SPLINE_CURVE_WITH_KNOTS('',3,(#19253,#19254,#19255,#19256,#19257,
#19258,#19259,#19260,#19261,#19262,#19263),.UNSPECIFIED.,.F.,.F.,(4,1,1,
1,1,1,1,1,4),(34.5575191894877,34.6896514237625,35.6822889264345,36.6749264291064,
37.6675639317784,38.6602014344503,39.6528389371222,40.6454764397942,40.8407044966673),
 .UNSPECIFIED.);
#2376=B_SPLINE_CURVE_WITH_KNOTS('',3,(#19264,#19265,#19266,#19267,#19268,
#19269,#19270,#19271,#19272,#19273),.UNSPECIFIED.,.F.,.F.,(4,1,1,1,1,1,
1,4),(34.5575191894877,35.2437876830827,36.2364251857546,37.2290626884266,
38.2217001910985,39.2143376937704,40.2069751964424,40.8407044966673),
 .UNSPECIFIED.);
#2377=B_SPLINE_CURVE_WITH_KNOTS('',3,(#19278,#19279,#19280,#19281,#19282,
#19283,#19284,#19285,#19286,#19287),.UNSPECIFIED.,.F.,.F.,(4,1,1,1,1,1,
1,4),(28.2743338823081,28.7338264077309,29.7264639104028,30.7191014130747,
31.7117389157467,32.7043764184186,33.6970139210906,34.5575191894877),
 .UNSPECIFIED.);
#2378=B_SPLINE_CURVE_WITH_KNOTS('',3,(#19288,#19289,#19290,#19291,#19292,
#19293,#19294,#19295,#19296,#19297,#19298),.UNSPECIFIED.,.F.,.F.,(4,1,1,
1,1,1,1,1,4),(28.2743338823081,28.2953251643791,29.287962667051,30.2806001697229,
31.2732376723949,32.2658751750668,33.2585126777388,34.2511501804107,34.5575191894877),
 .UNSPECIFIED.);
#2379=B_SPLINE_CURVE_WITH_KNOTS('',3,(#19303,#19304,#19305,#19306,#19307,
#19308,#19309,#19310,#19311,#19312),.UNSPECIFIED.,.F.,.F.,(4,1,1,1,1,1,
1,4),(21.9911485751285,22.7780013916992,23.7706388943711,24.7632763970431,
25.755913899715,26.748551402387,27.7411889050589,28.2743338823081),
 .UNSPECIFIED.);
#2380=B_SPLINE_CURVE_WITH_KNOTS('',3,(#19313,#19314,#19315,#19316,#19317,
#19318,#19319,#19320,#19321,#19322),.UNSPECIFIED.,.F.,.F.,(4,1,1,1,1,1,
1,4),(21.9911485751285,22.3395001483474,23.3321376510193,24.3247751536913,
25.3174126563632,26.3100501590352,27.3026876617071,28.2743338823081),
 .UNSPECIFIED.);
#2381=B_SPLINE_CURVE_WITH_KNOTS('',3,(#19328,#19329,#19330,#19331,#19332),
 .UNSPECIFIED.,.F.,.F.,(4,1,4),(14.3984001269718,15.3910376296438,15.7079632679489),
 .UNSPECIFIED.);
#2382=B_SPLINE_CURVE_WITH_KNOTS('',3,(#19335,#19336,#19337,#19338,#19339),
 .UNSPECIFIED.,.F.,.F.,(4,1,4),(13.8759337553362,14.8369013703236,15.7079632679489),
 .UNSPECIFIED.);
#2383=B_SPLINE_CURVE_WITH_KNOTS('',3,(#19345,#19346,#19347,#19348),
 .UNSPECIFIED.,.F.,.F.,(4,4),(57.8582309055934,58.5656126576447),
 .UNSPECIFIED.);
#2384=B_SPLINE_CURVE_WITH_KNOTS('',3,(#19356,#19357,#19358,#19359,#19360,
#19361,#19362,#19363,#19364,#19365),.UNSPECIFIED.,.F.,.F.,(4,3,3,4),(-56.5486677646163,
-55.5877001496289,-54.595062646957,-54.1144568630778),.UNSPECIFIED.);
#2385=B_SPLINE_CURVE_WITH_KNOTS('',3,(#19370,#19371,#19372,#19373,#19374,
#19375,#19376,#19377,#19378,#19379,#19380,#19381,#19382,#19383,#19384,#19385,
#19386,#19387,#19388,#19389,#19390,#19391,#19392,#19393,#19394),
 .UNSPECIFIED.,.F.,.F.,(4,3,3,3,3,3,3,3,4),(51.5750455984138,51.6171501389411,
52.6097876416131,53.602425144285,54.5950626469569,55.5877001496289,56.5803376523008,
57.5729751549728,57.8582309055934),.UNSPECIFIED.);
#2386=B_SPLINE_CURVE_WITH_KNOTS('',3,(#19395,#19396,#19397,#19398,#19399,
#19400,#19401,#19402,#19403,#19404,#19405,#19406,#19407,#19408,#19409,#19410,
#19411,#19412,#19413,#19414,#19415,#19416),.UNSPECIFIED.,.F.,.F.,(4,3,3,
3,3,3,3,4),(-54.1144568630778,-53.602425144285,-52.6097876416131,-51.6171501389411,
-50.6245126362692,-49.6318751335972,-48.6392376309253,-47.8312715558982),
 .UNSPECIFIED.);
#2387=B_SPLINE_CURVE_WITH_KNOTS('',3,(#19421,#19422,#19423,#19424,#19425,
#19426,#19427,#19428,#19429,#19430,#19431,#19432,#19433,#19434,#19435,#19436,
#19437,#19438,#19439,#19440,#19441,#19442),.UNSPECIFIED.,.F.,.F.,(4,3,3,
3,3,3,3,4),(45.2918602912342,45.6613251229094,46.6539626255814,47.6466001282533,
48.6392376309253,49.6318751335972,50.6245126362692,51.5750455984138),
 .UNSPECIFIED.);
#2388=B_SPLINE_CURVE_WITH_KNOTS('',3,(#19443,#19444,#19445,#19446,#19447,
#19448,#19449,#19450,#19451,#19452,#19453,#19454,#19455,#19456,#19457,#19458,
#19459,#19460,#19461,#19462,#19463,#19464,#19465,#19466,#19467),
 .UNSPECIFIED.,.F.,.F.,(4,3,3,3,3,3,3,3,4),(-47.8312715558982,-47.6466001282533,
-46.6539626255814,-45.6613251229095,-44.6686876202375,-43.6760501175656,
-42.6834126148936,-41.6907751122217,-41.5480862487187),.UNSPECIFIED.);
#2389=B_SPLINE_CURVE_WITH_KNOTS('',3,(#19472,#19473,#19474,#19475,#19476,
#19477,#19478,#19479,#19480,#19481,#19482,#19483,#19484,#19485,#19486,#19487,
#19488,#19489,#19490,#19491,#19492,#19493),.UNSPECIFIED.,.F.,.F.,(4,3,3,
3,3,3,3,4),(39.0086749840546,39.7055001068778,40.6981376095497,41.6907751122217,
42.6834126148936,43.6760501175656,44.6686876202375,45.2918602912342),
 .UNSPECIFIED.);
#2390=B_SPLINE_CURVE_WITH_KNOTS('',3,(#19494,#19495,#19496,#19497,#19498,
#19499,#19500,#19501,#19502,#19503,#19504,#19505,#19506,#19507,#19508,#19509,
#19510,#19511,#19512,#19513,#19514,#19515),.UNSPECIFIED.,.F.,.F.,(4,3,3,
3,3,3,3,4),(-41.5480862487187,-40.6981376095497,-39.7055001068778,-38.7128626042058,
-37.7202251015339,-36.727587598862,-35.73495009619,-35.2649009415391),
 .UNSPECIFIED.);
#2391=B_SPLINE_CURVE_WITH_KNOTS('',3,(#19520,#19521,#19522,#19523,#19524,
#19525,#19526,#19527,#19528,#19529,#19530,#19531,#19532,#19533,#19534,#19535,
#19536,#19537,#19538,#19539,#19540,#19541,#19542,#19543,#19544),
 .UNSPECIFIED.,.F.,.F.,(4,3,3,3,3,3,3,3,4),(32.725489676875,32.7570375881742,
33.7496750908461,34.7423125935181,35.73495009619,36.727587598862,37.7202251015339,
38.7128626042058,39.0086749840546),.UNSPECIFIED.);
#2392=B_SPLINE_CURVE_WITH_KNOTS('',3,(#19545,#19546,#19547,#19548,#19549,
#19550,#19551,#19552,#19553,#19554,#19555,#19556,#19557,#19558,#19559,#19560,
#19561,#19562,#19563,#19564,#19565,#19566),.UNSPECIFIED.,.F.,.F.,(4,3,3,
3,3,3,3,4),(-35.2649009415391,-34.7423125935181,-33.7496750908461,-32.7570375881742,
-31.7644000855022,-30.7717625828303,-29.7791250801584,-28.9817156343595),
 .UNSPECIFIED.);
#2393=B_SPLINE_CURVE_WITH_KNOTS('',3,(#19571,#19572,#19573,#19574,#19575,
#19576,#19577,#19578,#19579,#19580,#19581,#19582,#19583,#19584,#19585,#19586,
#19587,#19588,#19589,#19590,#19591,#19592),.UNSPECIFIED.,.F.,.F.,(4,3,3,
3,3,3,3,4),(26.4423043696954,26.8012125721425,27.7938500748145,28.7864875774864,
29.7791250801583,30.7717625828303,31.7644000855022,32.725489676875),
 .UNSPECIFIED.);
#2394=B_SPLINE_CURVE_WITH_KNOTS('',3,(#19593,#19594,#19595,#19596,#19597,
#19598,#19599,#19600,#19601,#19602,#19603,#19604,#19605,#19606,#19607,#19608,
#19609,#19610,#19611,#19612,#19613,#19614,#19615,#19616,#19617),
 .UNSPECIFIED.,.F.,.F.,(4,3,3,3,3,3,3,3,4),(-28.9817156343595,-28.7864875774864,
-27.7938500748145,-26.8012125721425,-25.8085750694706,-24.8159375667986,
-23.8233000641267,-22.8306625614547,-22.6985303271799),.UNSPECIFIED.);
#2395=B_SPLINE_CURVE_WITH_KNOTS('',3,(#19622,#19623,#19624,#19625,#19626,
#19627,#19628,#19629,#19630,#19631,#19632,#19633,#19634,#19635,#19636,#19637,
#19638,#19639,#19640,#19641,#19642,#19643),.UNSPECIFIED.,.F.,.F.,(4,3,3,
3,3,3,3,4),(20.1591190625158,20.8453875561108,21.8380250587828,22.8306625614547,
23.8233000641267,24.8159375667986,25.8085750694706,26.4423043696954),
 .UNSPECIFIED.);
#2396=B_SPLINE_CURVE_WITH_KNOTS('',3,(#19644,#19645,#19646,#19647,#19648,
#19649,#19650,#19651,#19652,#19653,#19654,#19655,#19656,#19657,#19658,#19659,
#19660,#19661,#19662,#19663,#19664,#19665),.UNSPECIFIED.,.F.,.F.,(4,3,3,
3,3,3,3,4),(-22.6985303271799,-21.8380250587828,-20.8453875561108,-19.8527500534389,
-18.8601125507669,-17.867475048095,-16.8748375454231,-16.4153450200003),
 .UNSPECIFIED.);
#2397=B_SPLINE_CURVE_WITH_KNOTS('',3,(#19670,#19671,#19672,#19673,#19674,
#19675,#19676,#19677,#19678,#19679,#19680,#19681,#19682,#19683,#19684,#19685,
#19686,#19687,#19688,#19689,#19690,#19691,#19692,#19693,#19694),
 .UNSPECIFIED.,.F.,.F.,(4,3,3,3,3,3,3,3,4),(13.8759337553362,13.8969250374072,
14.8895625400792,15.8822000427511,16.8748375454231,17.867475048095,18.8601125507669,
19.8527500534389,20.1591190625158),.UNSPECIFIED.);
#2398=B_SPLINE_CURVE_WITH_KNOTS('',3,(#19695,#19696,#19697,#19698,#19699,
#19700,#19701,#19702,#19703,#19704,#19705,#19706,#19707,#19708,#19709,#19710,
#19711,#19712,#19713,#19714,#19715,#19716),.UNSPECIFIED.,.F.,.F.,(4,3,3,
3,3,3,3,4),(-16.4153450200003,-15.8822000427511,-14.8895625400792,-13.8969250374072,
-12.9042875347353,-11.9116500320633,-10.9190125293914,-10.1321597128207),
 .UNSPECIFIED.);
#2399=B_SPLINE_CURVE_WITH_KNOTS('',3,(#19722,#19723,#19724,#19725,#19726,
#19727,#19728,#19729,#19730,#19731,#19732,#19733,#19734),.UNSPECIFIED.,
 .F.,.F.,(4,3,3,3,4),(-3.84897440564114,-2.97791250801584,-1.98527500534389,
-0.992637502671947,0.),.UNSPECIFIED.);
#2400=B_SPLINE_CURVE_WITH_KNOTS('',3,(#19737,#19738,#19739,#19740,#19741,
#19742,#19743,#19744,#19745,#19746,#19747,#19748,#19749,#19750,#19751,#19752,
#19753,#19754,#19755),.UNSPECIFIED.,.F.,.F.,(4,3,3,3,3,3,4),(2.01694489302844,
2.97791250801583,3.97055001068778,4.96318751335972,5.95582501603167,6.94846251870362,
7.59274844815666),.UNSPECIFIED.);
#2401=B_SPLINE_CURVE_WITH_KNOTS('',3,(#19761,#19762,#19763,#19764,#19765,
#19766,#19767,#19768),.UNSPECIFIED.,.F.,.F.,(4,1,1,1,1,4),(65.9734457253856,
66.4540515092647,67.4466890119367,68.4393265146086,69.4319640172806,70.4246015199525),
 .UNSPECIFIED.);
#2402=B_SPLINE_CURVE_WITH_KNOTS('',3,(#19771,#19772,#19773,#19774,#19775,
#19776,#19777,#19778,#19779),.UNSPECIFIED.,.F.,.F.,(4,1,1,1,1,1,4),(65.9734457253856,
66.0155502659129,67.0081877685849,68.0008252712568,68.9934627739288,69.9861002766007,
70.9470678915881),.UNSPECIFIED.);
#2403=B_SPLINE_CURVE_WITH_KNOTS('',3,(#19784,#19785,#19786,#19787,#19788,
#19789,#19790,#19791,#19792,#19793),.UNSPECIFIED.,.F.,.F.,(4,1,1,1,1,1,
1,4),(59.6902604182061,60.4982264932331,61.490863995905,62.483501498577,
63.4761390012489,64.4687765039209,65.4614140065928,65.9734457253856),
 .UNSPECIFIED.);
#2404=B_SPLINE_CURVE_WITH_KNOTS('',3,(#19794,#19795,#19796,#19797,#19798,
#19799,#19800,#19801,#19802,#19803),.UNSPECIFIED.,.F.,.F.,(4,1,1,1,1,1,
1,4),(59.6902604182061,60.0597252498813,61.0523627525532,62.0450002552252,
63.0376377578971,64.0302752605691,65.022912763241,65.9734457253856),
 .UNSPECIFIED.);
#2405=B_SPLINE_CURVE_WITH_KNOTS('',3,(#19808,#19809,#19810,#19811,#19812,
#19813,#19814,#19815,#19816,#19817,#19818),.UNSPECIFIED.,.F.,.F.,(4,1,1,
1,1,1,1,1,4),(53.4070751110265,53.5497639745295,54.5424014772014,55.5350389798734,
56.5276764825453,57.5203139852172,58.5129514878892,59.5055889905611,59.6902604182061),
 .UNSPECIFIED.);
#2406=B_SPLINE_CURVE_WITH_KNOTS('',3,(#19819,#19820,#19821,#19822,#19823,
#19824,#19825,#19826,#19827,#19828),.UNSPECIFIED.,.F.,.F.,(4,1,1,1,1,1,
1,4),(53.4070751110265,54.1039002338496,55.0965377365216,56.0891752391935,
57.0818127418654,58.0744502445374,59.0670877472093,59.6902604182061),
 .UNSPECIFIED.);
#2407=B_SPLINE_CURVE_WITH_KNOTS('',3,(#19833,#19834,#19835,#19836,#19837,
#19838,#19839,#19840,#19841,#19842),.UNSPECIFIED.,.F.,.F.,(4,1,1,1,1,1,
1,4),(47.1238898038469,47.5939389584978,48.5865764611697,49.5792139638417,
50.5718514665136,51.5644889691856,52.5571264718575,53.4070751110265),
 .UNSPECIFIED.);
#2408=B_SPLINE_CURVE_WITH_KNOTS('',3,(#19843,#19844,#19845,#19846,#19847,
#19848,#19849,#19850,#19851,#19852,#19853),.UNSPECIFIED.,.F.,.F.,(4,1,1,
1,1,1,1,1,4),(47.1238898038469,47.155437715146,48.1480752178179,49.1407127204899,
50.1333502231618,51.1259877258338,52.1186252285057,53.1112627311777,53.4070751110265),
 .UNSPECIFIED.);
#2409=B_SPLINE_CURVE_WITH_KNOTS('',3,(#19858,#19859,#19860,#19861,#19862,
#19863,#19864,#19865,#19866,#19867),.UNSPECIFIED.,.F.,.F.,(4,1,1,1,1,1,
1,4),(40.8407044966673,41.6381139424661,42.6307514451381,43.62338894781,
44.616026450482,45.6086639531539,46.6013014558259,47.1238898038469),
 .UNSPECIFIED.);
#2410=B_SPLINE_CURVE_WITH_KNOTS('',3,(#19868,#19869,#19870,#19871,#19872,
#19873,#19874,#19875,#19876,#19877),.UNSPECIFIED.,.F.,.F.,(4,1,1,1,1,1,
1,4),(40.8407044966673,41.1996126991143,42.1922502017863,43.1848877044582,
44.1775252071302,45.1701627098021,46.1628002124741,47.1238898038469),
 .UNSPECIFIED.);
#2411=B_SPLINE_CURVE_WITH_KNOTS('',3,(#19882,#19883,#19884,#19885,#19886,
#19887,#19888,#19889,#19890,#19891,#19892),.UNSPECIFIED.,.F.,.F.,(4,1,1,
1,1,1,1,1,4),(34.5575191894877,34.6896514237625,35.6822889264345,36.6749264291064,
37.6675639317784,38.6602014344503,39.6528389371222,40.6454764397942,40.8407044966673),
 .UNSPECIFIED.);
#2412=B_SPLINE_CURVE_WITH_KNOTS('',3,(#19893,#19894,#19895,#19896,#19897,
#19898,#19899,#19900,#19901,#19902),.UNSPECIFIED.,.F.,.F.,(4,1,1,1,1,1,
1,4),(34.5575191894877,35.2437876830827,36.2364251857546,37.2290626884266,
38.2217001910985,39.2143376937704,40.2069751964424,40.8407044966673),
 .UNSPECIFIED.);
#2413=B_SPLINE_CURVE_WITH_KNOTS('',3,(#19907,#19908,#19909,#19910,#19911,
#19912,#19913,#19914,#19915,#19916),.UNSPECIFIED.,.F.,.F.,(4,1,1,1,1,1,
1,4),(28.2743338823081,28.7338264077309,29.7264639104028,30.7191014130747,
31.7117389157467,32.7043764184186,33.6970139210906,34.5575191894877),
 .UNSPECIFIED.);
#2414=B_SPLINE_CURVE_WITH_KNOTS('',3,(#19917,#19918,#19919,#19920,#19921,
#19922,#19923,#19924,#19925,#19926,#19927),.UNSPECIFIED.,.F.,.F.,(4,1,1,
1,1,1,1,1,4),(28.2743338823081,28.2953251643791,29.287962667051,30.2806001697229,
31.2732376723949,32.2658751750668,33.2585126777388,34.2511501804107,34.5575191894877),
 .UNSPECIFIED.);
#2415=B_SPLINE_CURVE_WITH_KNOTS('',3,(#19932,#19933,#19934,#19935,#19936,
#19937,#19938,#19939,#19940,#19941),.UNSPECIFIED.,.F.,.F.,(4,1,1,1,1,1,
1,4),(21.9911485751285,22.7780013916992,23.7706388943711,24.7632763970431,
25.755913899715,26.748551402387,27.7411889050589,28.2743338823081),
 .UNSPECIFIED.);
#2416=B_SPLINE_CURVE_WITH_KNOTS('',3,(#19942,#19943,#19944,#19945,#19946,
#19947,#19948,#19949,#19950,#19951),.UNSPECIFIED.,.F.,.F.,(4,1,1,1,1,1,
1,4),(21.9911485751285,22.3395001483474,23.3321376510193,24.3247751536913,
25.3174126563632,26.3100501590352,27.3026876617071,28.2743338823081),
 .UNSPECIFIED.);
#2417=B_SPLINE_CURVE_WITH_KNOTS('',3,(#19957,#19958,#19959,#19960,#19961),
 .UNSPECIFIED.,.F.,.F.,(4,1,4),(14.3984001269718,15.3910376296438,15.7079632679489),
 .UNSPECIFIED.);
#2418=B_SPLINE_CURVE_WITH_KNOTS('',3,(#19964,#19965,#19966,#19967,#19968),
 .UNSPECIFIED.,.F.,.F.,(4,1,4),(13.8759337553362,14.8369013703236,15.7079632679489),
 .UNSPECIFIED.);
#2419=B_SPLINE_CURVE_WITH_KNOTS('',3,(#19974,#19975,#19976,#19977),
 .UNSPECIFIED.,.F.,.F.,(4,4),(57.8582309055934,58.5656126576448),
 .UNSPECIFIED.);
#2420=B_SPLINE_CURVE_WITH_KNOTS('',3,(#19985,#19986,#19987,#19988,#19989,
#19990,#19991,#19992,#19993,#19994),.UNSPECIFIED.,.F.,.F.,(4,3,3,4),(-56.5486677646163,
-55.5877001496289,-54.595062646957,-54.1144568630778),.UNSPECIFIED.);
#2421=B_SPLINE_CURVE_WITH_KNOTS('',3,(#19999,#20000,#20001,#20002,#20003,
#20004,#20005,#20006,#20007,#20008,#20009,#20010,#20011,#20012,#20013,#20014,
#20015,#20016,#20017,#20018,#20019,#20020,#20021,#20022,#20023),
 .UNSPECIFIED.,.F.,.F.,(4,3,3,3,3,3,3,3,4),(51.5750455984138,51.6171501389411,
52.6097876416131,53.602425144285,54.595062646957,55.5877001496289,56.5803376523009,
57.5729751549728,57.8582309055934),.UNSPECIFIED.);
#2422=B_SPLINE_CURVE_WITH_KNOTS('',3,(#20024,#20025,#20026,#20027,#20028,
#20029,#20030,#20031,#20032,#20033,#20034,#20035,#20036,#20037,#20038,#20039,
#20040,#20041,#20042,#20043,#20044,#20045),.UNSPECIFIED.,.F.,.F.,(4,3,3,
3,3,3,3,4),(-54.1144568630778,-53.602425144285,-52.6097876416131,-51.6171501389411,
-50.6245126362692,-49.6318751335972,-48.6392376309253,-47.8312715558982),
 .UNSPECIFIED.);
#2423=B_SPLINE_CURVE_WITH_KNOTS('',3,(#20050,#20051,#20052,#20053,#20054,
#20055,#20056,#20057,#20058,#20059,#20060,#20061,#20062,#20063,#20064,#20065,
#20066,#20067,#20068,#20069,#20070,#20071),.UNSPECIFIED.,.F.,.F.,(4,3,3,
3,3,3,3,4),(45.2918602912342,45.6613251229095,46.6539626255814,47.6466001282534,
48.6392376309253,49.6318751335973,50.6245126362692,51.5750455984138),
 .UNSPECIFIED.);
#2424=B_SPLINE_CURVE_WITH_KNOTS('',3,(#20072,#20073,#20074,#20075,#20076,
#20077,#20078,#20079,#20080,#20081,#20082,#20083,#20084,#20085,#20086,#20087,
#20088,#20089,#20090,#20091,#20092,#20093,#20094,#20095,#20096),
 .UNSPECIFIED.,.F.,.F.,(4,3,3,3,3,3,3,3,4),(-47.8312715558982,-47.6466001282533,
-46.6539626255814,-45.6613251229095,-44.6686876202375,-43.6760501175656,
-42.6834126148936,-41.6907751122217,-41.5480862487187),.UNSPECIFIED.);
#2425=B_SPLINE_CURVE_WITH_KNOTS('',3,(#20101,#20102,#20103,#20104,#20105,
#20106,#20107,#20108,#20109,#20110,#20111,#20112,#20113,#20114,#20115,#20116,
#20117,#20118,#20119,#20120,#20121,#20122),.UNSPECIFIED.,.F.,.F.,(4,3,3,
3,3,3,3,4),(39.0086749840546,39.7055001068778,40.6981376095497,41.6907751122217,
42.6834126148936,43.6760501175656,44.6686876202375,45.2918602912342),
 .UNSPECIFIED.);
#2426=B_SPLINE_CURVE_WITH_KNOTS('',3,(#20123,#20124,#20125,#20126,#20127,
#20128,#20129,#20130,#20131,#20132,#20133,#20134,#20135,#20136,#20137,#20138,
#20139,#20140,#20141,#20142,#20143,#20144),.UNSPECIFIED.,.F.,.F.,(4,3,3,
3,3,3,3,4),(-41.5480862487187,-40.6981376095497,-39.7055001068778,-38.7128626042058,
-37.7202251015339,-36.727587598862,-35.73495009619,-35.2649009415391),
 .UNSPECIFIED.);
#2427=B_SPLINE_CURVE_WITH_KNOTS('',3,(#20149,#20150,#20151,#20152,#20153,
#20154,#20155,#20156,#20157,#20158,#20159,#20160,#20161,#20162,#20163,#20164,
#20165,#20166,#20167,#20168,#20169,#20170,#20171,#20172,#20173),
 .UNSPECIFIED.,.F.,.F.,(4,3,3,3,3,3,3,3,4),(32.725489676875,32.7570375881742,
33.7496750908461,34.7423125935181,35.73495009619,36.727587598862,37.7202251015339,
38.7128626042059,39.0086749840546),.UNSPECIFIED.);
#2428=B_SPLINE_CURVE_WITH_KNOTS('',3,(#20174,#20175,#20176,#20177,#20178,
#20179,#20180,#20181,#20182,#20183,#20184,#20185,#20186,#20187,#20188,#20189,
#20190,#20191,#20192,#20193,#20194,#20195),.UNSPECIFIED.,.F.,.F.,(4,3,3,
3,3,3,3,4),(-35.2649009415391,-34.7423125935181,-33.7496750908461,-32.7570375881742,
-31.7644000855022,-30.7717625828303,-29.7791250801584,-28.9817156343595),
 .UNSPECIFIED.);
#2429=B_SPLINE_CURVE_WITH_KNOTS('',3,(#20200,#20201,#20202,#20203,#20204,
#20205,#20206,#20207,#20208,#20209,#20210,#20211,#20212,#20213,#20214,#20215,
#20216,#20217,#20218,#20219,#20220,#20221),.UNSPECIFIED.,.F.,.F.,(4,3,3,
3,3,3,3,4),(26.4423043696954,26.8012125721425,27.7938500748145,28.7864875774864,
29.7791250801583,30.7717625828303,31.7644000855022,32.725489676875),
 .UNSPECIFIED.);
#2430=B_SPLINE_CURVE_WITH_KNOTS('',3,(#20222,#20223,#20224,#20225,#20226,
#20227,#20228,#20229,#20230,#20231,#20232,#20233,#20234,#20235,#20236,#20237,
#20238,#20239,#20240,#20241,#20242,#20243,#20244,#20245,#20246),
 .UNSPECIFIED.,.F.,.F.,(4,3,3,3,3,3,3,3,4),(-28.9817156343595,-28.7864875774864,
-27.7938500748145,-26.8012125721425,-25.8085750694706,-24.8159375667986,
-23.8233000641267,-22.8306625614547,-22.6985303271799),.UNSPECIFIED.);
#2431=B_SPLINE_CURVE_WITH_KNOTS('',3,(#20251,#20252,#20253,#20254,#20255,
#20256,#20257,#20258,#20259,#20260,#20261,#20262,#20263,#20264,#20265,#20266,
#20267,#20268,#20269,#20270,#20271,#20272),.UNSPECIFIED.,.F.,.F.,(4,3,3,
3,3,3,3,4),(20.1591190625158,20.8453875561108,21.8380250587828,22.8306625614547,
23.8233000641267,24.8159375667986,25.8085750694706,26.4423043696954),
 .UNSPECIFIED.);
#2432=B_SPLINE_CURVE_WITH_KNOTS('',3,(#20273,#20274,#20275,#20276,#20277,
#20278,#20279,#20280,#20281,#20282,#20283,#20284,#20285,#20286,#20287,#20288,
#20289,#20290,#20291,#20292,#20293,#20294),.UNSPECIFIED.,.F.,.F.,(4,3,3,
3,3,3,3,4),(-22.6985303271799,-21.8380250587828,-20.8453875561108,-19.8527500534389,
-18.860112550767,-17.867475048095,-16.8748375454231,-16.4153450200003),
 .UNSPECIFIED.);
#2433=B_SPLINE_CURVE_WITH_KNOTS('',3,(#20299,#20300,#20301,#20302,#20303,
#20304,#20305,#20306,#20307,#20308,#20309,#20310,#20311,#20312,#20313,#20314,
#20315,#20316,#20317,#20318,#20319,#20320,#20321,#20322,#20323),
 .UNSPECIFIED.,.F.,.F.,(4,3,3,3,3,3,3,3,4),(13.8759337553362,13.8969250374072,
14.8895625400792,15.8822000427511,16.8748375454231,17.867475048095,18.860112550767,
19.8527500534389,20.1591190625158),.UNSPECIFIED.);
#2434=B_SPLINE_CURVE_WITH_KNOTS('',3,(#20324,#20325,#20326,#20327,#20328,
#20329,#20330,#20331,#20332,#20333,#20334,#20335,#20336,#20337,#20338,#20339,
#20340,#20341,#20342,#20343,#20344,#20345),.UNSPECIFIED.,.F.,.F.,(4,3,3,
3,3,3,3,4),(-16.4153450200003,-15.8822000427511,-14.8895625400792,-13.8969250374072,
-12.9042875347353,-11.9116500320633,-10.9190125293914,-10.1321597128207),
 .UNSPECIFIED.);
#2435=B_SPLINE_CURVE_WITH_KNOTS('',3,(#20351,#20352,#20353,#20354,#20355,
#20356,#20357,#20358,#20359,#20360,#20361,#20362,#20363),.UNSPECIFIED.,
 .F.,.F.,(4,3,3,3,4),(-3.84897440564114,-2.97791250801583,-1.98527500534389,
-0.992637502671945,0.),.UNSPECIFIED.);
#2436=B_SPLINE_CURVE_WITH_KNOTS('',3,(#20366,#20367,#20368,#20369,#20370,
#20371,#20372,#20373,#20374,#20375,#20376,#20377,#20378,#20379,#20380,#20381,
#20382,#20383,#20384),.UNSPECIFIED.,.F.,.F.,(4,3,3,3,3,3,4),(2.01694489302845,
2.97791250801584,3.97055001068779,4.96318751335973,5.95582501603167,6.94846251870361,
7.59274844815666),.UNSPECIFIED.);
#2437=B_SPLINE_CURVE_WITH_KNOTS('',3,(#20390,#20391,#20392,#20393,#20394,
#20395,#20396,#20397),.UNSPECIFIED.,.F.,.F.,(4,1,1,1,1,4),(65.9734457253856,
66.4540515092647,67.4466890119367,68.4393265146086,69.4319640172806,70.4246015199525),
 .UNSPECIFIED.);
#2438=B_SPLINE_CURVE_WITH_KNOTS('',3,(#20400,#20401,#20402,#20403,#20404,
#20405,#20406,#20407,#20408),.UNSPECIFIED.,.F.,.F.,(4,1,1,1,1,1,4),(65.9734457253856,
66.015550265913,67.0081877685849,68.0008252712569,68.9934627739288,69.9861002766008,
70.9470678915881),.UNSPECIFIED.);
#2439=B_SPLINE_CURVE_WITH_KNOTS('',3,(#20413,#20414,#20415,#20416,#20417,
#20418,#20419,#20420,#20421,#20422),.UNSPECIFIED.,.F.,.F.,(4,1,1,1,1,1,
1,4),(59.6902604182061,60.4982264932331,61.490863995905,62.483501498577,
63.4761390012489,64.4687765039209,65.4614140065928,65.9734457253856),
 .UNSPECIFIED.);
#2440=B_SPLINE_CURVE_WITH_KNOTS('',3,(#20423,#20424,#20425,#20426,#20427,
#20428,#20429,#20430,#20431,#20432),.UNSPECIFIED.,.F.,.F.,(4,1,1,1,1,1,
1,4),(59.6902604182061,60.0597252498813,61.0523627525533,62.0450002552252,
63.0376377578971,64.0302752605691,65.022912763241,65.9734457253856),
 .UNSPECIFIED.);
#2441=B_SPLINE_CURVE_WITH_KNOTS('',3,(#20437,#20438,#20439,#20440,#20441,
#20442,#20443,#20444,#20445,#20446,#20447),.UNSPECIFIED.,.F.,.F.,(4,1,1,
1,1,1,1,1,4),(53.4070751110265,53.5497639745295,54.5424014772014,55.5350389798734,
56.5276764825453,57.5203139852172,58.5129514878892,59.5055889905611,59.6902604182061),
 .UNSPECIFIED.);
#2442=B_SPLINE_CURVE_WITH_KNOTS('',3,(#20448,#20449,#20450,#20451,#20452,
#20453,#20454,#20455,#20456,#20457),.UNSPECIFIED.,.F.,.F.,(4,1,1,1,1,1,
1,4),(53.4070751110265,54.1039002338496,55.0965377365216,56.0891752391935,
57.0818127418655,58.0744502445374,59.0670877472094,59.6902604182061),
 .UNSPECIFIED.);
#2443=B_SPLINE_CURVE_WITH_KNOTS('',3,(#20462,#20463,#20464,#20465,#20466,
#20467,#20468,#20469,#20470,#20471),.UNSPECIFIED.,.F.,.F.,(4,1,1,1,1,1,
1,4),(47.1238898038469,47.5939389584978,48.5865764611697,49.5792139638417,
50.5718514665136,51.5644889691856,52.5571264718575,53.4070751110265),
 .UNSPECIFIED.);
#2444=B_SPLINE_CURVE_WITH_KNOTS('',3,(#20472,#20473,#20474,#20475,#20476,
#20477,#20478,#20479,#20480,#20481,#20482),.UNSPECIFIED.,.F.,.F.,(4,1,1,
1,1,1,1,1,4),(47.1238898038469,47.155437715146,48.148075217818,49.1407127204899,
50.1333502231619,51.1259877258338,52.1186252285057,53.1112627311777,53.4070751110265),
 .UNSPECIFIED.);
#2445=B_SPLINE_CURVE_WITH_KNOTS('',3,(#20487,#20488,#20489,#20490,#20491,
#20492,#20493,#20494,#20495,#20496),.UNSPECIFIED.,.F.,.F.,(4,1,1,1,1,1,
1,4),(40.8407044966673,41.6381139424661,42.6307514451381,43.62338894781,
44.616026450482,45.6086639531539,46.6013014558259,47.1238898038469),
 .UNSPECIFIED.);
#2446=B_SPLINE_CURVE_WITH_KNOTS('',3,(#20497,#20498,#20499,#20500,#20501,
#20502,#20503,#20504,#20505,#20506),.UNSPECIFIED.,.F.,.F.,(4,1,1,1,1,1,
1,4),(40.8407044966673,41.1996126991143,42.1922502017863,43.1848877044582,
44.1775252071302,45.1701627098021,46.1628002124741,47.1238898038469),
 .UNSPECIFIED.);
#2447=B_SPLINE_CURVE_WITH_KNOTS('',3,(#20511,#20512,#20513,#20514,#20515,
#20516,#20517,#20518,#20519,#20520,#20521),.UNSPECIFIED.,.F.,.F.,(4,1,1,
1,1,1,1,1,4),(34.5575191894877,34.6896514237625,35.6822889264345,36.6749264291064,
37.6675639317784,38.6602014344503,39.6528389371222,40.6454764397942,40.8407044966673),
 .UNSPECIFIED.);
#2448=B_SPLINE_CURVE_WITH_KNOTS('',3,(#20522,#20523,#20524,#20525,#20526,
#20527,#20528,#20529,#20530,#20531),.UNSPECIFIED.,.F.,.F.,(4,1,1,1,1,1,
1,4),(34.5575191894877,35.2437876830827,36.2364251857546,37.2290626884266,
38.2217001910985,39.2143376937705,40.2069751964424,40.8407044966673),
 .UNSPECIFIED.);
#2449=B_SPLINE_CURVE_WITH_KNOTS('',3,(#20536,#20537,#20538,#20539,#20540,
#20541,#20542,#20543,#20544,#20545),.UNSPECIFIED.,.F.,.F.,(4,1,1,1,1,1,
1,4),(28.2743338823081,28.7338264077309,29.7264639104028,30.7191014130747,
31.7117389157467,32.7043764184186,33.6970139210906,34.5575191894877),
 .UNSPECIFIED.);
#2450=B_SPLINE_CURVE_WITH_KNOTS('',3,(#20546,#20547,#20548,#20549,#20550,
#20551,#20552,#20553,#20554,#20555,#20556),.UNSPECIFIED.,.F.,.F.,(4,1,1,
1,1,1,1,1,4),(28.2743338823081,28.2953251643791,29.287962667051,30.280600169723,
31.2732376723949,32.2658751750668,33.2585126777388,34.2511501804107,34.5575191894877),
 .UNSPECIFIED.);
#2451=B_SPLINE_CURVE_WITH_KNOTS('',3,(#20561,#20562,#20563,#20564,#20565,
#20566,#20567,#20568,#20569,#20570),.UNSPECIFIED.,.F.,.F.,(4,1,1,1,1,1,
1,4),(21.9911485751285,22.7780013916992,23.7706388943711,24.7632763970431,
25.755913899715,26.748551402387,27.7411889050589,28.2743338823081),
 .UNSPECIFIED.);
#2452=B_SPLINE_CURVE_WITH_KNOTS('',3,(#20571,#20572,#20573,#20574,#20575,
#20576,#20577,#20578,#20579,#20580),.UNSPECIFIED.,.F.,.F.,(4,1,1,1,1,1,
1,4),(21.9911485751285,22.3395001483474,23.3321376510193,24.3247751536913,
25.3174126563632,26.3100501590352,27.3026876617071,28.2743338823081),
 .UNSPECIFIED.);
#2453=B_SPLINE_CURVE_WITH_KNOTS('',3,(#20586,#20587,#20588,#20589,#20590),
 .UNSPECIFIED.,.F.,.F.,(4,1,4),(14.3984001269718,15.3910376296438,15.7079632679489),
 .UNSPECIFIED.);
#2454=B_SPLINE_CURVE_WITH_KNOTS('',3,(#20593,#20594,#20595,#20596,#20597),
 .UNSPECIFIED.,.F.,.F.,(4,1,4),(13.8759337553362,14.8369013703236,15.7079632679489),
 .UNSPECIFIED.);
#2455=B_SPLINE_CURVE_WITH_KNOTS('',3,(#20603,#20604,#20605,#20606),
 .UNSPECIFIED.,.F.,.F.,(4,4),(57.8582309055934,58.5656126576448),
 .UNSPECIFIED.);
#2456=B_SPLINE_CURVE_WITH_KNOTS('',3,(#20614,#20615,#20616,#20617,#20618,
#20619,#20620,#20621,#20622,#20623),.UNSPECIFIED.,.F.,.F.,(4,3,3,4),(-56.5486677646163,
-55.5877001496289,-54.595062646957,-54.1144568630778),.UNSPECIFIED.);
#2457=B_SPLINE_CURVE_WITH_KNOTS('',3,(#20628,#20629,#20630,#20631,#20632,
#20633,#20634,#20635,#20636,#20637,#20638,#20639,#20640,#20641,#20642,#20643,
#20644,#20645,#20646,#20647,#20648,#20649,#20650,#20651,#20652),
 .UNSPECIFIED.,.F.,.F.,(4,3,3,3,3,3,3,3,4),(51.5750455984138,51.6171501389411,
52.6097876416131,53.602425144285,54.595062646957,55.5877001496289,56.5803376523009,
57.5729751549728,57.8582309055934),.UNSPECIFIED.);
#2458=B_SPLINE_CURVE_WITH_KNOTS('',3,(#20653,#20654,#20655,#20656,#20657,
#20658,#20659,#20660,#20661,#20662,#20663,#20664,#20665,#20666,#20667,#20668,
#20669,#20670,#20671,#20672,#20673,#20674),.UNSPECIFIED.,.F.,.F.,(4,3,3,
3,3,3,3,4),(-54.1144568630778,-53.602425144285,-52.6097876416131,-51.6171501389411,
-50.6245126362692,-49.6318751335972,-48.6392376309253,-47.8312715558982),
 .UNSPECIFIED.);
#2459=B_SPLINE_CURVE_WITH_KNOTS('',3,(#20679,#20680,#20681,#20682,#20683,
#20684,#20685,#20686,#20687,#20688,#20689,#20690,#20691,#20692,#20693,#20694,
#20695,#20696,#20697,#20698,#20699,#20700),.UNSPECIFIED.,.F.,.F.,(4,3,3,
3,3,3,3,4),(45.2918602912342,45.6613251229095,46.6539626255814,47.6466001282534,
48.6392376309253,49.6318751335973,50.6245126362692,51.5750455984138),
 .UNSPECIFIED.);
#2460=B_SPLINE_CURVE_WITH_KNOTS('',3,(#20701,#20702,#20703,#20704,#20705,
#20706,#20707,#20708,#20709,#20710,#20711,#20712,#20713,#20714,#20715,#20716,
#20717,#20718,#20719,#20720,#20721,#20722,#20723,#20724,#20725),
 .UNSPECIFIED.,.F.,.F.,(4,3,3,3,3,3,3,3,4),(-47.8312715558982,-47.6466001282533,
-46.6539626255814,-45.6613251229095,-44.6686876202375,-43.6760501175656,
-42.6834126148936,-41.6907751122217,-41.5480862487187),.UNSPECIFIED.);
#2461=B_SPLINE_CURVE_WITH_KNOTS('',3,(#20730,#20731,#20732,#20733,#20734,
#20735,#20736,#20737,#20738,#20739,#20740,#20741,#20742,#20743,#20744,#20745,
#20746,#20747,#20748,#20749,#20750,#20751),.UNSPECIFIED.,.F.,.F.,(4,3,3,
3,3,3,3,4),(39.0086749840546,39.7055001068778,40.6981376095497,41.6907751122217,
42.6834126148936,43.6760501175656,44.6686876202375,45.2918602912342),
 .UNSPECIFIED.);
#2462=B_SPLINE_CURVE_WITH_KNOTS('',3,(#20752,#20753,#20754,#20755,#20756,
#20757,#20758,#20759,#20760,#20761,#20762,#20763,#20764,#20765,#20766,#20767,
#20768,#20769,#20770,#20771,#20772,#20773),.UNSPECIFIED.,.F.,.F.,(4,3,3,
3,3,3,3,4),(-41.5480862487187,-40.6981376095497,-39.7055001068778,-38.7128626042058,
-37.7202251015339,-36.727587598862,-35.73495009619,-35.2649009415391),
 .UNSPECIFIED.);
#2463=B_SPLINE_CURVE_WITH_KNOTS('',3,(#20778,#20779,#20780,#20781,#20782,
#20783,#20784,#20785,#20786,#20787,#20788,#20789,#20790,#20791,#20792,#20793,
#20794,#20795,#20796,#20797,#20798,#20799,#20800,#20801,#20802),
 .UNSPECIFIED.,.F.,.F.,(4,3,3,3,3,3,3,3,4),(32.725489676875,32.7570375881742,
33.7496750908461,34.7423125935181,35.73495009619,36.727587598862,37.7202251015339,
38.7128626042059,39.0086749840546),.UNSPECIFIED.);
#2464=B_SPLINE_CURVE_WITH_KNOTS('',3,(#20803,#20804,#20805,#20806,#20807,
#20808,#20809,#20810,#20811,#20812,#20813,#20814,#20815,#20816,#20817,#20818,
#20819,#20820,#20821,#20822,#20823,#20824),.UNSPECIFIED.,.F.,.F.,(4,3,3,
3,3,3,3,4),(-35.2649009415391,-34.7423125935181,-33.7496750908461,-32.7570375881742,
-31.7644000855022,-30.7717625828303,-29.7791250801584,-28.9817156343595),
 .UNSPECIFIED.);
#2465=B_SPLINE_CURVE_WITH_KNOTS('',3,(#20829,#20830,#20831,#20832,#20833,
#20834,#20835,#20836,#20837,#20838,#20839,#20840,#20841,#20842,#20843,#20844,
#20845,#20846,#20847,#20848,#20849,#20850),.UNSPECIFIED.,.F.,.F.,(4,3,3,
3,3,3,3,4),(26.4423043696954,26.8012125721425,27.7938500748145,28.7864875774864,
29.7791250801583,30.7717625828303,31.7644000855022,32.725489676875),
 .UNSPECIFIED.);
#2466=B_SPLINE_CURVE_WITH_KNOTS('',3,(#20851,#20852,#20853,#20854,#20855,
#20856,#20857,#20858,#20859,#20860,#20861,#20862,#20863,#20864,#20865,#20866,
#20867,#20868,#20869,#20870,#20871,#20872,#20873,#20874,#20875),
 .UNSPECIFIED.,.F.,.F.,(4,3,3,3,3,3,3,3,4),(-28.9817156343595,-28.7864875774864,
-27.7938500748145,-26.8012125721425,-25.8085750694706,-24.8159375667986,
-23.8233000641267,-22.8306625614547,-22.6985303271799),.UNSPECIFIED.);
#2467=B_SPLINE_CURVE_WITH_KNOTS('',3,(#20880,#20881,#20882,#20883,#20884,
#20885,#20886,#20887,#20888,#20889,#20890,#20891,#20892,#20893,#20894,#20895,
#20896,#20897,#20898,#20899,#20900,#20901),.UNSPECIFIED.,.F.,.F.,(4,3,3,
3,3,3,3,4),(20.1591190625158,20.8453875561108,21.8380250587828,22.8306625614547,
23.8233000641267,24.8159375667986,25.8085750694706,26.4423043696954),
 .UNSPECIFIED.);
#2468=B_SPLINE_CURVE_WITH_KNOTS('',3,(#20902,#20903,#20904,#20905,#20906,
#20907,#20908,#20909,#20910,#20911,#20912,#20913,#20914,#20915,#20916,#20917,
#20918,#20919,#20920,#20921,#20922,#20923),.UNSPECIFIED.,.F.,.F.,(4,3,3,
3,3,3,3,4),(-22.6985303271799,-21.8380250587828,-20.8453875561108,-19.8527500534389,
-18.860112550767,-17.867475048095,-16.8748375454231,-16.4153450200003),
 .UNSPECIFIED.);
#2469=B_SPLINE_CURVE_WITH_KNOTS('',3,(#20928,#20929,#20930,#20931,#20932,
#20933,#20934,#20935,#20936,#20937,#20938,#20939,#20940,#20941,#20942,#20943,
#20944,#20945,#20946,#20947,#20948,#20949,#20950,#20951,#20952),
 .UNSPECIFIED.,.F.,.F.,(4,3,3,3,3,3,3,3,4),(13.8759337553362,13.8969250374072,
14.8895625400792,15.8822000427511,16.8748375454231,17.867475048095,18.860112550767,
19.8527500534389,20.1591190625158),.UNSPECIFIED.);
#2470=B_SPLINE_CURVE_WITH_KNOTS('',3,(#20953,#20954,#20955,#20956,#20957,
#20958,#20959,#20960,#20961,#20962,#20963,#20964,#20965,#20966,#20967,#20968,
#20969,#20970,#20971,#20972,#20973,#20974),.UNSPECIFIED.,.F.,.F.,(4,3,3,
3,3,3,3,4),(-16.4153450200003,-15.8822000427511,-14.8895625400792,-13.8969250374072,
-12.9042875347353,-11.9116500320633,-10.9190125293914,-10.1321597128207),
 .UNSPECIFIED.);
#2471=B_SPLINE_CURVE_WITH_KNOTS('',3,(#20980,#20981,#20982,#20983,#20984,
#20985,#20986,#20987,#20988,#20989,#20990,#20991,#20992),.UNSPECIFIED.,
 .F.,.F.,(4,3,3,3,4),(-3.84897440564114,-2.97791250801583,-1.98527500534389,
-0.992637502671945,0.),.UNSPECIFIED.);
#2472=B_SPLINE_CURVE_WITH_KNOTS('',3,(#20995,#20996,#20997,#20998,#20999,
#21000,#21001,#21002,#21003,#21004,#21005,#21006,#21007,#21008,#21009,#21010,
#21011,#21012,#21013),.UNSPECIFIED.,.F.,.F.,(4,3,3,3,3,3,4),(2.01694489302845,
2.97791250801584,3.97055001068779,4.96318751335973,5.95582501603167,6.94846251870361,
7.59274844815666),.UNSPECIFIED.);
#2473=B_SPLINE_CURVE_WITH_KNOTS('',3,(#21019,#21020,#21021,#21022,#21023,
#21024,#21025,#21026),.UNSPECIFIED.,.F.,.F.,(4,1,1,1,1,4),(65.9734457253856,
66.4540515092647,67.4466890119367,68.4393265146086,69.4319640172806,70.4246015199525),
 .UNSPECIFIED.);
#2474=B_SPLINE_CURVE_WITH_KNOTS('',3,(#21029,#21030,#21031,#21032,#21033,
#21034,#21035,#21036,#21037),.UNSPECIFIED.,.F.,.F.,(4,1,1,1,1,1,4),(65.9734457253856,
66.015550265913,67.0081877685849,68.0008252712569,68.9934627739288,69.9861002766008,
70.9470678915881),.UNSPECIFIED.);
#2475=B_SPLINE_CURVE_WITH_KNOTS('',3,(#21042,#21043,#21044,#21045,#21046,
#21047,#21048,#21049,#21050,#21051),.UNSPECIFIED.,.F.,.F.,(4,1,1,1,1,1,
1,4),(59.6902604182061,60.4982264932331,61.490863995905,62.483501498577,
63.4761390012489,64.4687765039209,65.4614140065928,65.9734457253856),
 .UNSPECIFIED.);
#2476=B_SPLINE_CURVE_WITH_KNOTS('',3,(#21052,#21053,#21054,#21055,#21056,
#21057,#21058,#21059,#21060,#21061),.UNSPECIFIED.,.F.,.F.,(4,1,1,1,1,1,
1,4),(59.6902604182061,60.0597252498813,61.0523627525533,62.0450002552252,
63.0376377578971,64.0302752605691,65.022912763241,65.9734457253856),
 .UNSPECIFIED.);
#2477=B_SPLINE_CURVE_WITH_KNOTS('',3,(#21066,#21067,#21068,#21069,#21070,
#21071,#21072,#21073,#21074,#21075,#21076),.UNSPECIFIED.,.F.,.F.,(4,1,1,
1,1,1,1,1,4),(53.4070751110265,53.5497639745295,54.5424014772014,55.5350389798734,
56.5276764825453,57.5203139852172,58.5129514878892,59.5055889905611,59.6902604182061),
 .UNSPECIFIED.);
#2478=B_SPLINE_CURVE_WITH_KNOTS('',3,(#21077,#21078,#21079,#21080,#21081,
#21082,#21083,#21084,#21085,#21086),.UNSPECIFIED.,.F.,.F.,(4,1,1,1,1,1,
1,4),(53.4070751110265,54.1039002338496,55.0965377365216,56.0891752391935,
57.0818127418655,58.0744502445374,59.0670877472094,59.6902604182061),
 .UNSPECIFIED.);
#2479=B_SPLINE_CURVE_WITH_KNOTS('',3,(#21091,#21092,#21093,#21094,#21095,
#21096,#21097,#21098,#21099,#21100),.UNSPECIFIED.,.F.,.F.,(4,1,1,1,1,1,
1,4),(47.1238898038469,47.5939389584978,48.5865764611697,49.5792139638417,
50.5718514665136,51.5644889691856,52.5571264718575,53.4070751110265),
 .UNSPECIFIED.);
#2480=B_SPLINE_CURVE_WITH_KNOTS('',3,(#21101,#21102,#21103,#21104,#21105,
#21106,#21107,#21108,#21109,#21110,#21111),.UNSPECIFIED.,.F.,.F.,(4,1,1,
1,1,1,1,1,4),(47.1238898038469,47.155437715146,48.148075217818,49.1407127204899,
50.1333502231619,51.1259877258338,52.1186252285057,53.1112627311777,53.4070751110265),
 .UNSPECIFIED.);
#2481=B_SPLINE_CURVE_WITH_KNOTS('',3,(#21116,#21117,#21118,#21119,#21120,
#21121,#21122,#21123,#21124,#21125),.UNSPECIFIED.,.F.,.F.,(4,1,1,1,1,1,
1,4),(40.8407044966673,41.6381139424661,42.6307514451381,43.62338894781,
44.616026450482,45.6086639531539,46.6013014558259,47.1238898038469),
 .UNSPECIFIED.);
#2482=B_SPLINE_CURVE_WITH_KNOTS('',3,(#21126,#21127,#21128,#21129,#21130,
#21131,#21132,#21133,#21134,#21135),.UNSPECIFIED.,.F.,.F.,(4,1,1,1,1,1,
1,4),(40.8407044966673,41.1996126991143,42.1922502017863,43.1848877044582,
44.1775252071302,45.1701627098021,46.1628002124741,47.1238898038469),
 .UNSPECIFIED.);
#2483=B_SPLINE_CURVE_WITH_KNOTS('',3,(#21140,#21141,#21142,#21143,#21144,
#21145,#21146,#21147,#21148,#21149,#21150),.UNSPECIFIED.,.F.,.F.,(4,1,1,
1,1,1,1,1,4),(34.5575191894877,34.6896514237625,35.6822889264345,36.6749264291064,
37.6675639317784,38.6602014344503,39.6528389371222,40.6454764397942,40.8407044966673),
 .UNSPECIFIED.);
#2484=B_SPLINE_CURVE_WITH_KNOTS('',3,(#21151,#21152,#21153,#21154,#21155,
#21156,#21157,#21158,#21159,#21160),.UNSPECIFIED.,.F.,.F.,(4,1,1,1,1,1,
1,4),(34.5575191894877,35.2437876830827,36.2364251857546,37.2290626884266,
38.2217001910985,39.2143376937705,40.2069751964424,40.8407044966673),
 .UNSPECIFIED.);
#2485=B_SPLINE_CURVE_WITH_KNOTS('',3,(#21165,#21166,#21167,#21168,#21169,
#21170,#21171,#21172,#21173,#21174),.UNSPECIFIED.,.F.,.F.,(4,1,1,1,1,1,
1,4),(28.2743338823081,28.7338264077309,29.7264639104028,30.7191014130747,
31.7117389157467,32.7043764184186,33.6970139210906,34.5575191894877),
 .UNSPECIFIED.);
#2486=B_SPLINE_CURVE_WITH_KNOTS('',3,(#21175,#21176,#21177,#21178,#21179,
#21180,#21181,#21182,#21183,#21184,#21185),.UNSPECIFIED.,.F.,.F.,(4,1,1,
1,1,1,1,1,4),(28.2743338823081,28.2953251643791,29.287962667051,30.280600169723,
31.2732376723949,32.2658751750668,33.2585126777388,34.2511501804107,34.5575191894877),
 .UNSPECIFIED.);
#2487=B_SPLINE_CURVE_WITH_KNOTS('',3,(#21190,#21191,#21192,#21193,#21194,
#21195,#21196,#21197,#21198,#21199),.UNSPECIFIED.,.F.,.F.,(4,1,1,1,1,1,
1,4),(21.9911485751285,22.7780013916992,23.7706388943711,24.7632763970431,
25.755913899715,26.748551402387,27.7411889050589,28.2743338823081),
 .UNSPECIFIED.);
#2488=B_SPLINE_CURVE_WITH_KNOTS('',3,(#21200,#21201,#21202,#21203,#21204,
#21205,#21206,#21207,#21208,#21209),.UNSPECIFIED.,.F.,.F.,(4,1,1,1,1,1,
1,4),(21.9911485751285,22.3395001483474,23.3321376510193,24.3247751536913,
25.3174126563632,26.3100501590352,27.3026876617071,28.2743338823081),
 .UNSPECIFIED.);
#2489=B_SPLINE_CURVE_WITH_KNOTS('',3,(#21215,#21216,#21217,#21218,#21219),
 .UNSPECIFIED.,.F.,.F.,(4,1,4),(14.3984001269718,15.3910376296438,15.7079632679489),
 .UNSPECIFIED.);
#2490=B_SPLINE_CURVE_WITH_KNOTS('',3,(#21222,#21223,#21224,#21225,#21226),
 .UNSPECIFIED.,.F.,.F.,(4,1,4),(13.8759337553362,14.8369013703236,15.7079632679489),
 .UNSPECIFIED.);
#2491=B_SPLINE_CURVE_WITH_KNOTS('',3,(#21232,#21233,#21234,#21235),
 .UNSPECIFIED.,.F.,.F.,(4,4),(57.8582309055934,58.5656126576447),
 .UNSPECIFIED.);
#2492=B_SPLINE_CURVE_WITH_KNOTS('',3,(#21243,#21244,#21245,#21246,#21247,
#21248,#21249,#21250,#21251,#21252),.UNSPECIFIED.,.F.,.F.,(4,3,3,4),(-56.5486677646163,
-55.5877001496289,-54.595062646957,-54.1144568630778),.UNSPECIFIED.);
#2493=B_SPLINE_CURVE_WITH_KNOTS('',3,(#21257,#21258,#21259,#21260,#21261,
#21262,#21263,#21264,#21265,#21266,#21267,#21268,#21269,#21270,#21271,#21272,
#21273,#21274,#21275,#21276,#21277,#21278,#21279,#21280,#21281),
 .UNSPECIFIED.,.F.,.F.,(4,3,3,3,3,3,3,3,4),(51.5750455984138,51.6171501389411,
52.6097876416131,53.602425144285,54.5950626469569,55.5877001496289,56.5803376523008,
57.5729751549728,57.8582309055934),.UNSPECIFIED.);
#2494=B_SPLINE_CURVE_WITH_KNOTS('',3,(#21282,#21283,#21284,#21285,#21286,
#21287,#21288,#21289,#21290,#21291,#21292,#21293,#21294,#21295,#21296,#21297,
#21298,#21299,#21300,#21301,#21302,#21303),.UNSPECIFIED.,.F.,.F.,(4,3,3,
3,3,3,3,4),(-54.1144568630778,-53.602425144285,-52.6097876416131,-51.6171501389411,
-50.6245126362692,-49.6318751335972,-48.6392376309253,-47.8312715558982),
 .UNSPECIFIED.);
#2495=B_SPLINE_CURVE_WITH_KNOTS('',3,(#21308,#21309,#21310,#21311,#21312,
#21313,#21314,#21315,#21316,#21317,#21318,#21319,#21320,#21321,#21322,#21323,
#21324,#21325,#21326,#21327,#21328,#21329),.UNSPECIFIED.,.F.,.F.,(4,3,3,
3,3,3,3,4),(45.2918602912342,45.6613251229094,46.6539626255814,47.6466001282533,
48.6392376309253,49.6318751335972,50.6245126362692,51.5750455984138),
 .UNSPECIFIED.);
#2496=B_SPLINE_CURVE_WITH_KNOTS('',3,(#21330,#21331,#21332,#21333,#21334,
#21335,#21336,#21337,#21338,#21339,#21340,#21341,#21342,#21343,#21344,#21345,
#21346,#21347,#21348,#21349,#21350,#21351,#21352,#21353,#21354),
 .UNSPECIFIED.,.F.,.F.,(4,3,3,3,3,3,3,3,4),(-47.8312715558982,-47.6466001282533,
-46.6539626255814,-45.6613251229095,-44.6686876202375,-43.6760501175656,
-42.6834126148936,-41.6907751122217,-41.5480862487187),.UNSPECIFIED.);
#2497=B_SPLINE_CURVE_WITH_KNOTS('',3,(#21359,#21360,#21361,#21362,#21363,
#21364,#21365,#21366,#21367,#21368,#21369,#21370,#21371,#21372,#21373,#21374,
#21375,#21376,#21377,#21378,#21379,#21380),.UNSPECIFIED.,.F.,.F.,(4,3,3,
3,3,3,3,4),(39.0086749840546,39.7055001068778,40.6981376095497,41.6907751122217,
42.6834126148936,43.6760501175656,44.6686876202375,45.2918602912342),
 .UNSPECIFIED.);
#2498=B_SPLINE_CURVE_WITH_KNOTS('',3,(#21381,#21382,#21383,#21384,#21385,
#21386,#21387,#21388,#21389,#21390,#21391,#21392,#21393,#21394,#21395,#21396,
#21397,#21398,#21399,#21400,#21401,#21402),.UNSPECIFIED.,.F.,.F.,(4,3,3,
3,3,3,3,4),(-41.5480862487187,-40.6981376095497,-39.7055001068778,-38.7128626042058,
-37.7202251015339,-36.727587598862,-35.73495009619,-35.2649009415391),
 .UNSPECIFIED.);
#2499=B_SPLINE_CURVE_WITH_KNOTS('',3,(#21407,#21408,#21409,#21410,#21411,
#21412,#21413,#21414,#21415,#21416,#21417,#21418,#21419,#21420,#21421,#21422,
#21423,#21424,#21425,#21426,#21427,#21428,#21429,#21430,#21431),
 .UNSPECIFIED.,.F.,.F.,(4,3,3,3,3,3,3,3,4),(32.725489676875,32.7570375881742,
33.7496750908461,34.7423125935181,35.73495009619,36.727587598862,37.7202251015339,
38.7128626042058,39.0086749840546),.UNSPECIFIED.);
#2500=B_SPLINE_CURVE_WITH_KNOTS('',3,(#21432,#21433,#21434,#21435,#21436,
#21437,#21438,#21439,#21440,#21441,#21442,#21443,#21444,#21445,#21446,#21447,
#21448,#21449,#21450,#21451,#21452,#21453),.UNSPECIFIED.,.F.,.F.,(4,3,3,
3,3,3,3,4),(-35.2649009415391,-34.7423125935181,-33.7496750908461,-32.7570375881742,
-31.7644000855022,-30.7717625828303,-29.7791250801584,-28.9817156343595),
 .UNSPECIFIED.);
#2501=B_SPLINE_CURVE_WITH_KNOTS('',3,(#21458,#21459,#21460,#21461,#21462,
#21463,#21464,#21465,#21466,#21467,#21468,#21469,#21470,#21471,#21472,#21473,
#21474,#21475,#21476,#21477,#21478,#21479),.UNSPECIFIED.,.F.,.F.,(4,3,3,
3,3,3,3,4),(26.4423043696954,26.8012125721425,27.7938500748145,28.7864875774864,
29.7791250801583,30.7717625828303,31.7644000855022,32.725489676875),
 .UNSPECIFIED.);
#2502=B_SPLINE_CURVE_WITH_KNOTS('',3,(#21480,#21481,#21482,#21483,#21484,
#21485,#21486,#21487,#21488,#21489,#21490,#21491,#21492,#21493,#21494,#21495,
#21496,#21497,#21498,#21499,#21500,#21501,#21502,#21503,#21504),
 .UNSPECIFIED.,.F.,.F.,(4,3,3,3,3,3,3,3,4),(-28.9817156343595,-28.7864875774864,
-27.7938500748145,-26.8012125721425,-25.8085750694706,-24.8159375667986,
-23.8233000641267,-22.8306625614547,-22.6985303271799),.UNSPECIFIED.);
#2503=B_SPLINE_CURVE_WITH_KNOTS('',3,(#21509,#21510,#21511,#21512,#21513,
#21514,#21515,#21516,#21517,#21518,#21519,#21520,#21521,#21522,#21523,#21524,
#21525,#21526,#21527,#21528,#21529,#21530),.UNSPECIFIED.,.F.,.F.,(4,3,3,
3,3,3,3,4),(20.1591190625158,20.8453875561108,21.8380250587828,22.8306625614547,
23.8233000641267,24.8159375667986,25.8085750694706,26.4423043696954),
 .UNSPECIFIED.);
#2504=B_SPLINE_CURVE_WITH_KNOTS('',3,(#21531,#21532,#21533,#21534,#21535,
#21536,#21537,#21538,#21539,#21540,#21541,#21542,#21543,#21544,#21545,#21546,
#21547,#21548,#21549,#21550,#21551,#21552),.UNSPECIFIED.,.F.,.F.,(4,3,3,
3,3,3,3,4),(-22.6985303271799,-21.8380250587828,-20.8453875561108,-19.8527500534389,
-18.8601125507669,-17.867475048095,-16.8748375454231,-16.4153450200003),
 .UNSPECIFIED.);
#2505=B_SPLINE_CURVE_WITH_KNOTS('',3,(#21557,#21558,#21559,#21560,#21561,
#21562,#21563,#21564,#21565,#21566,#21567,#21568,#21569,#21570,#21571,#21572,
#21573,#21574,#21575,#21576,#21577,#21578,#21579,#21580,#21581),
 .UNSPECIFIED.,.F.,.F.,(4,3,3,3,3,3,3,3,4),(13.8759337553362,13.8969250374072,
14.8895625400792,15.8822000427511,16.8748375454231,17.867475048095,18.8601125507669,
19.8527500534389,20.1591190625158),.UNSPECIFIED.);
#2506=B_SPLINE_CURVE_WITH_KNOTS('',3,(#21582,#21583,#21584,#21585,#21586,
#21587,#21588,#21589,#21590,#21591,#21592,#21593,#21594,#21595,#21596,#21597,
#21598,#21599,#21600,#21601,#21602,#21603),.UNSPECIFIED.,.F.,.F.,(4,3,3,
3,3,3,3,4),(-16.4153450200003,-15.8822000427511,-14.8895625400792,-13.8969250374072,
-12.9042875347353,-11.9116500320633,-10.9190125293914,-10.1321597128207),
 .UNSPECIFIED.);
#2507=B_SPLINE_CURVE_WITH_KNOTS('',3,(#21609,#21610,#21611,#21612,#21613,
#21614,#21615,#21616,#21617,#21618,#21619,#21620,#21621),.UNSPECIFIED.,
 .F.,.F.,(4,3,3,3,4),(-3.84897440564114,-2.97791250801584,-1.98527500534389,
-0.992637502671947,0.),.UNSPECIFIED.);
#2508=B_SPLINE_CURVE_WITH_KNOTS('',3,(#21624,#21625,#21626,#21627,#21628,
#21629,#21630,#21631,#21632,#21633,#21634,#21635,#21636,#21637,#21638,#21639,
#21640,#21641,#21642),.UNSPECIFIED.,.F.,.F.,(4,3,3,3,3,3,4),(2.01694489302844,
2.97791250801583,3.97055001068778,4.96318751335972,5.95582501603167,6.94846251870362,
7.59274844815666),.UNSPECIFIED.);
#2509=B_SPLINE_CURVE_WITH_KNOTS('',3,(#21648,#21649,#21650,#21651,#21652,
#21653,#21654,#21655),.UNSPECIFIED.,.F.,.F.,(4,1,1,1,1,4),(65.9734457253856,
66.4540515092647,67.4466890119367,68.4393265146086,69.4319640172806,70.4246015199525),
 .UNSPECIFIED.);
#2510=B_SPLINE_CURVE_WITH_KNOTS('',3,(#21658,#21659,#21660,#21661,#21662,
#21663,#21664,#21665,#21666),.UNSPECIFIED.,.F.,.F.,(4,1,1,1,1,1,4),(65.9734457253856,
66.0155502659129,67.0081877685849,68.0008252712568,68.9934627739288,69.9861002766007,
70.9470678915881),.UNSPECIFIED.);
#2511=B_SPLINE_CURVE_WITH_KNOTS('',3,(#21671,#21672,#21673,#21674,#21675,
#21676,#21677,#21678,#21679,#21680),.UNSPECIFIED.,.F.,.F.,(4,1,1,1,1,1,
1,4),(59.6902604182061,60.4982264932331,61.490863995905,62.483501498577,
63.4761390012489,64.4687765039209,65.4614140065928,65.9734457253856),
 .UNSPECIFIED.);
#2512=B_SPLINE_CURVE_WITH_KNOTS('',3,(#21681,#21682,#21683,#21684,#21685,
#21686,#21687,#21688,#21689,#21690),.UNSPECIFIED.,.F.,.F.,(4,1,1,1,1,1,
1,4),(59.6902604182061,60.0597252498813,61.0523627525532,62.0450002552252,
63.0376377578971,64.0302752605691,65.022912763241,65.9734457253856),
 .UNSPECIFIED.);
#2513=B_SPLINE_CURVE_WITH_KNOTS('',3,(#21695,#21696,#21697,#21698,#21699,
#21700,#21701,#21702,#21703,#21704,#21705),.UNSPECIFIED.,.F.,.F.,(4,1,1,
1,1,1,1,1,4),(53.4070751110265,53.5497639745295,54.5424014772014,55.5350389798734,
56.5276764825453,57.5203139852172,58.5129514878892,59.5055889905611,59.6902604182061),
 .UNSPECIFIED.);
#2514=B_SPLINE_CURVE_WITH_KNOTS('',3,(#21706,#21707,#21708,#21709,#21710,
#21711,#21712,#21713,#21714,#21715),.UNSPECIFIED.,.F.,.F.,(4,1,1,1,1,1,
1,4),(53.4070751110265,54.1039002338496,55.0965377365216,56.0891752391935,
57.0818127418654,58.0744502445374,59.0670877472093,59.6902604182061),
 .UNSPECIFIED.);
#2515=B_SPLINE_CURVE_WITH_KNOTS('',3,(#21720,#21721,#21722,#21723,#21724,
#21725,#21726,#21727,#21728,#21729),.UNSPECIFIED.,.F.,.F.,(4,1,1,1,1,1,
1,4),(47.1238898038469,47.5939389584978,48.5865764611697,49.5792139638417,
50.5718514665136,51.5644889691856,52.5571264718575,53.4070751110265),
 .UNSPECIFIED.);
#2516=B_SPLINE_CURVE_WITH_KNOTS('',3,(#21730,#21731,#21732,#21733,#21734,
#21735,#21736,#21737,#21738,#21739,#21740),.UNSPECIFIED.,.F.,.F.,(4,1,1,
1,1,1,1,1,4),(47.1238898038469,47.155437715146,48.1480752178179,49.1407127204899,
50.1333502231618,51.1259877258338,52.1186252285057,53.1112627311777,53.4070751110265),
 .UNSPECIFIED.);
#2517=B_SPLINE_CURVE_WITH_KNOTS('',3,(#21745,#21746,#21747,#21748,#21749,
#21750,#21751,#21752,#21753,#21754),.UNSPECIFIED.,.F.,.F.,(4,1,1,1,1,1,
1,4),(40.8407044966673,41.6381139424661,42.6307514451381,43.62338894781,
44.616026450482,45.6086639531539,46.6013014558259,47.1238898038469),
 .UNSPECIFIED.);
#2518=B_SPLINE_CURVE_WITH_KNOTS('',3,(#21755,#21756,#21757,#21758,#21759,
#21760,#21761,#21762,#21763,#21764),.UNSPECIFIED.,.F.,.F.,(4,1,1,1,1,1,
1,4),(40.8407044966673,41.1996126991143,42.1922502017863,43.1848877044582,
44.1775252071302,45.1701627098021,46.1628002124741,47.1238898038469),
 .UNSPECIFIED.);
#2519=B_SPLINE_CURVE_WITH_KNOTS('',3,(#21769,#21770,#21771,#21772,#21773,
#21774,#21775,#21776,#21777,#21778,#21779),.UNSPECIFIED.,.F.,.F.,(4,1,1,
1,1,1,1,1,4),(34.5575191894877,34.6896514237625,35.6822889264345,36.6749264291064,
37.6675639317784,38.6602014344503,39.6528389371222,40.6454764397942,40.8407044966673),
 .UNSPECIFIED.);
#2520=B_SPLINE_CURVE_WITH_KNOTS('',3,(#21780,#21781,#21782,#21783,#21784,
#21785,#21786,#21787,#21788,#21789),.UNSPECIFIED.,.F.,.F.,(4,1,1,1,1,1,
1,4),(34.5575191894877,35.2437876830827,36.2364251857546,37.2290626884266,
38.2217001910985,39.2143376937704,40.2069751964424,40.8407044966673),
 .UNSPECIFIED.);
#2521=B_SPLINE_CURVE_WITH_KNOTS('',3,(#21794,#21795,#21796,#21797,#21798,
#21799,#21800,#21801,#21802,#21803),.UNSPECIFIED.,.F.,.F.,(4,1,1,1,1,1,
1,4),(28.2743338823081,28.7338264077309,29.7264639104028,30.7191014130747,
31.7117389157467,32.7043764184186,33.6970139210906,34.5575191894877),
 .UNSPECIFIED.);
#2522=B_SPLINE_CURVE_WITH_KNOTS('',3,(#21804,#21805,#21806,#21807,#21808,
#21809,#21810,#21811,#21812,#21813,#21814),.UNSPECIFIED.,.F.,.F.,(4,1,1,
1,1,1,1,1,4),(28.2743338823081,28.2953251643791,29.287962667051,30.2806001697229,
31.2732376723949,32.2658751750668,33.2585126777388,34.2511501804107,34.5575191894877),
 .UNSPECIFIED.);
#2523=B_SPLINE_CURVE_WITH_KNOTS('',3,(#21819,#21820,#21821,#21822,#21823,
#21824,#21825,#21826,#21827,#21828),.UNSPECIFIED.,.F.,.F.,(4,1,1,1,1,1,
1,4),(21.9911485751285,22.7780013916992,23.7706388943711,24.7632763970431,
25.755913899715,26.748551402387,27.7411889050589,28.2743338823081),
 .UNSPECIFIED.);
#2524=B_SPLINE_CURVE_WITH_KNOTS('',3,(#21829,#21830,#21831,#21832,#21833,
#21834,#21835,#21836,#21837,#21838),.UNSPECIFIED.,.F.,.F.,(4,1,1,1,1,1,
1,4),(21.9911485751285,22.3395001483474,23.3321376510193,24.3247751536913,
25.3174126563632,26.3100501590352,27.3026876617071,28.2743338823081),
 .UNSPECIFIED.);
#2525=B_SPLINE_CURVE_WITH_KNOTS('',3,(#21844,#21845,#21846,#21847,#21848),
 .UNSPECIFIED.,.F.,.F.,(4,1,4),(14.3984001269718,15.3910376296438,15.7079632679489),
 .UNSPECIFIED.);
#2526=B_SPLINE_CURVE_WITH_KNOTS('',3,(#21851,#21852,#21853,#21854,#21855),
 .UNSPECIFIED.,.F.,.F.,(4,1,4),(13.8759337553362,14.8369013703236,15.7079632679489),
 .UNSPECIFIED.);
#2527=B_SPLINE_CURVE_WITH_KNOTS('',3,(#21861,#21862,#21863,#21864),
 .UNSPECIFIED.,.F.,.F.,(4,4),(57.8582309055934,58.5656126576448),
 .UNSPECIFIED.);
#2528=B_SPLINE_CURVE_WITH_KNOTS('',3,(#21872,#21873,#21874,#21875,#21876,
#21877,#21878,#21879,#21880,#21881),.UNSPECIFIED.,.F.,.F.,(4,3,3,4),(-56.5486677646163,
-55.5877001496289,-54.595062646957,-54.1144568630778),.UNSPECIFIED.);
#2529=B_SPLINE_CURVE_WITH_KNOTS('',3,(#21886,#21887,#21888,#21889,#21890,
#21891,#21892,#21893,#21894,#21895,#21896,#21897,#21898,#21899,#21900,#21901,
#21902,#21903,#21904,#21905,#21906,#21907,#21908,#21909,#21910),
 .UNSPECIFIED.,.F.,.F.,(4,3,3,3,3,3,3,3,4),(51.5750455984138,51.6171501389411,
52.6097876416131,53.602425144285,54.595062646957,55.5877001496289,56.5803376523009,
57.5729751549728,57.8582309055934),.UNSPECIFIED.);
#2530=B_SPLINE_CURVE_WITH_KNOTS('',3,(#21911,#21912,#21913,#21914,#21915,
#21916,#21917,#21918,#21919,#21920,#21921,#21922,#21923,#21924,#21925,#21926,
#21927,#21928,#21929,#21930,#21931,#21932),.UNSPECIFIED.,.F.,.F.,(4,3,3,
3,3,3,3,4),(-54.1144568630778,-53.602425144285,-52.6097876416131,-51.6171501389411,
-50.6245126362692,-49.6318751335972,-48.6392376309253,-47.8312715558982),
 .UNSPECIFIED.);
#2531=B_SPLINE_CURVE_WITH_KNOTS('',3,(#21937,#21938,#21939,#21940,#21941,
#21942,#21943,#21944,#21945,#21946,#21947,#21948,#21949,#21950,#21951,#21952,
#21953,#21954,#21955,#21956,#21957,#21958),.UNSPECIFIED.,.F.,.F.,(4,3,3,
3,3,3,3,4),(45.2918602912342,45.6613251229095,46.6539626255814,47.6466001282534,
48.6392376309253,49.6318751335972,50.6245126362692,51.5750455984138),
 .UNSPECIFIED.);
#2532=B_SPLINE_CURVE_WITH_KNOTS('',3,(#21959,#21960,#21961,#21962,#21963,
#21964,#21965,#21966,#21967,#21968,#21969,#21970,#21971,#21972,#21973,#21974,
#21975,#21976,#21977,#21978,#21979,#21980,#21981,#21982,#21983),
 .UNSPECIFIED.,.F.,.F.,(4,3,3,3,3,3,3,3,4),(-47.8312715558982,-47.6466001282533,
-46.6539626255814,-45.6613251229094,-44.6686876202375,-43.6760501175656,
-42.6834126148936,-41.6907751122217,-41.5480862487187),.UNSPECIFIED.);
#2533=B_SPLINE_CURVE_WITH_KNOTS('',3,(#21988,#21989,#21990,#21991,#21992,
#21993,#21994,#21995,#21996,#21997,#21998,#21999,#22000,#22001,#22002,#22003,
#22004,#22005,#22006,#22007,#22008,#22009),.UNSPECIFIED.,.F.,.F.,(4,3,3,
3,3,3,3,4),(39.0086749840546,39.7055001068778,40.6981376095497,41.6907751122217,
42.6834126148936,43.6760501175656,44.6686876202375,45.2918602912342),
 .UNSPECIFIED.);
#2534=B_SPLINE_CURVE_WITH_KNOTS('',3,(#22010,#22011,#22012,#22013,#22014,
#22015,#22016,#22017,#22018,#22019,#22020,#22021,#22022,#22023,#22024,#22025,
#22026,#22027,#22028,#22029,#22030,#22031),.UNSPECIFIED.,.F.,.F.,(4,3,3,
3,3,3,3,4),(-41.5480862487187,-40.6981376095497,-39.7055001068778,-38.7128626042058,
-37.7202251015339,-36.7275875988619,-35.73495009619,-35.2649009415391),
 .UNSPECIFIED.);
#2535=B_SPLINE_CURVE_WITH_KNOTS('',3,(#22036,#22037,#22038,#22039,#22040,
#22041,#22042,#22043,#22044,#22045,#22046,#22047,#22048,#22049,#22050,#22051,
#22052,#22053,#22054,#22055,#22056,#22057,#22058,#22059,#22060),
 .UNSPECIFIED.,.F.,.F.,(4,3,3,3,3,3,3,3,4),(32.725489676875,32.7570375881742,
33.7496750908461,34.7423125935181,35.73495009619,36.727587598862,37.7202251015339,
38.7128626042059,39.0086749840546),.UNSPECIFIED.);
#2536=B_SPLINE_CURVE_WITH_KNOTS('',3,(#22061,#22062,#22063,#22064,#22065,
#22066,#22067,#22068,#22069,#22070,#22071,#22072,#22073,#22074,#22075,#22076,
#22077,#22078,#22079,#22080,#22081,#22082),.UNSPECIFIED.,.F.,.F.,(4,3,3,
3,3,3,3,4),(-35.2649009415391,-34.7423125935181,-33.7496750908461,-32.7570375881742,
-31.7644000855022,-30.7717625828303,-29.7791250801583,-28.9817156343595),
 .UNSPECIFIED.);
#2537=B_SPLINE_CURVE_WITH_KNOTS('',3,(#22087,#22088,#22089,#22090,#22091,
#22092,#22093,#22094,#22095,#22096,#22097,#22098,#22099,#22100,#22101,#22102,
#22103,#22104,#22105,#22106,#22107,#22108),.UNSPECIFIED.,.F.,.F.,(4,3,3,
3,3,3,3,4),(26.4423043696954,26.8012125721425,27.7938500748145,28.7864875774864,
29.7791250801583,30.7717625828303,31.7644000855022,32.725489676875),
 .UNSPECIFIED.);
#2538=B_SPLINE_CURVE_WITH_KNOTS('',3,(#22109,#22110,#22111,#22112,#22113,
#22114,#22115,#22116,#22117,#22118,#22119,#22120,#22121,#22122,#22123,#22124,
#22125,#22126,#22127,#22128,#22129,#22130,#22131,#22132,#22133),
 .UNSPECIFIED.,.F.,.F.,(4,3,3,3,3,3,3,3,4),(-28.9817156343595,-28.7864875774864,
-27.7938500748144,-26.8012125721425,-25.8085750694706,-24.8159375667986,
-23.8233000641267,-22.8306625614547,-22.6985303271799),.UNSPECIFIED.);
#2539=B_SPLINE_CURVE_WITH_KNOTS('',3,(#22138,#22139,#22140,#22141,#22142,
#22143,#22144,#22145,#22146,#22147,#22148,#22149,#22150,#22151,#22152,#22153,
#22154,#22155,#22156,#22157,#22158,#22159),.UNSPECIFIED.,.F.,.F.,(4,3,3,
3,3,3,3,4),(20.1591190625158,20.8453875561108,21.8380250587828,22.8306625614547,
23.8233000641267,24.8159375667986,25.8085750694706,26.4423043696954),
 .UNSPECIFIED.);
#2540=B_SPLINE_CURVE_WITH_KNOTS('',3,(#22160,#22161,#22162,#22163,#22164,
#22165,#22166,#22167,#22168,#22169,#22170,#22171,#22172,#22173,#22174,#22175,
#22176,#22177,#22178,#22179,#22180,#22181),.UNSPECIFIED.,.F.,.F.,(4,3,3,
3,3,3,3,4),(-22.6985303271799,-21.8380250587828,-20.8453875561108,-19.8527500534389,
-18.8601125507669,-17.867475048095,-16.8748375454231,-16.4153450200003),
 .UNSPECIFIED.);
#2541=B_SPLINE_CURVE_WITH_KNOTS('',3,(#22186,#22187,#22188,#22189,#22190,
#22191,#22192,#22193,#22194,#22195,#22196,#22197,#22198,#22199,#22200,#22201,
#22202,#22203,#22204,#22205,#22206,#22207,#22208,#22209,#22210),
 .UNSPECIFIED.,.F.,.F.,(4,3,3,3,3,3,3,3,4),(13.8759337553362,13.8969250374072,
14.8895625400792,15.8822000427511,16.8748375454231,17.867475048095,18.860112550767,
19.8527500534389,20.1591190625158),.UNSPECIFIED.);
#2542=B_SPLINE_CURVE_WITH_KNOTS('',3,(#22211,#22212,#22213,#22214,#22215,
#22216,#22217,#22218,#22219,#22220,#22221,#22222,#22223,#22224,#22225,#22226,
#22227,#22228,#22229,#22230,#22231,#22232),.UNSPECIFIED.,.F.,.F.,(4,3,3,
3,3,3,3,4),(-16.4153450200003,-15.8822000427511,-14.8895625400792,-13.8969250374072,
-12.9042875347353,-11.9116500320633,-10.9190125293914,-10.1321597128207),
 .UNSPECIFIED.);
#2543=B_SPLINE_CURVE_WITH_KNOTS('',3,(#22238,#22239,#22240,#22241,#22242,
#22243,#22244,#22245,#22246,#22247,#22248,#22249,#22250),.UNSPECIFIED.,
 .F.,.F.,(4,3,3,3,4),(-3.84897440564113,-2.97791250801583,-1.98527500534389,
-0.992637502671945,0.),.UNSPECIFIED.);
#2544=B_SPLINE_CURVE_WITH_KNOTS('',3,(#22253,#22254,#22255,#22256,#22257,
#22258,#22259,#22260,#22261,#22262,#22263,#22264,#22265,#22266,#22267,#22268,
#22269,#22270,#22271),.UNSPECIFIED.,.F.,.F.,(4,3,3,3,3,3,4),(2.0169448930284,
2.97791250801584,3.97055001068778,4.96318751335973,5.95582501603167,6.94846251870361,
7.59274844815666),.UNSPECIFIED.);
#2545=B_SPLINE_CURVE_WITH_KNOTS('',3,(#22277,#22278,#22279,#22280,#22281,
#22282,#22283,#22284),.UNSPECIFIED.,.F.,.F.,(4,1,1,1,1,4),(65.9734457253856,
66.4540515092647,67.4466890119367,68.4393265146086,69.4319640172806,70.4246015199525),
 .UNSPECIFIED.);
#2546=B_SPLINE_CURVE_WITH_KNOTS('',3,(#22287,#22288,#22289,#22290,#22291,
#22292,#22293,#22294,#22295),.UNSPECIFIED.,.F.,.F.,(4,1,1,1,1,1,4),(65.9734457253857,
66.015550265913,67.0081877685849,68.0008252712569,68.9934627739288,69.9861002766008,
70.9470678915881),.UNSPECIFIED.);
#2547=B_SPLINE_CURVE_WITH_KNOTS('',3,(#22300,#22301,#22302,#22303,#22304,
#22305,#22306,#22307,#22308,#22309),.UNSPECIFIED.,.F.,.F.,(4,1,1,1,1,1,
1,4),(59.6902604182061,60.4982264932331,61.490863995905,62.483501498577,
63.4761390012489,64.4687765039209,65.4614140065928,65.9734457253856),
 .UNSPECIFIED.);
#2548=B_SPLINE_CURVE_WITH_KNOTS('',3,(#22310,#22311,#22312,#22313,#22314,
#22315,#22316,#22317,#22318,#22319),.UNSPECIFIED.,.F.,.F.,(4,1,1,1,1,1,
1,4),(59.6902604182061,60.0597252498813,61.0523627525533,62.0450002552252,
63.0376377578971,64.0302752605691,65.022912763241,65.9734457253857),
 .UNSPECIFIED.);
#2549=B_SPLINE_CURVE_WITH_KNOTS('',3,(#22324,#22325,#22326,#22327,#22328,
#22329,#22330,#22331,#22332,#22333,#22334),.UNSPECIFIED.,.F.,.F.,(4,1,1,
1,1,1,1,1,4),(53.4070751110265,53.5497639745295,54.5424014772014,55.5350389798734,
56.5276764825453,57.5203139852172,58.5129514878892,59.5055889905611,59.6902604182061),
 .UNSPECIFIED.);
#2550=B_SPLINE_CURVE_WITH_KNOTS('',3,(#22335,#22336,#22337,#22338,#22339,
#22340,#22341,#22342,#22343,#22344),.UNSPECIFIED.,.F.,.F.,(4,1,1,1,1,1,
1,4),(53.4070751110265,54.1039002338496,55.0965377365216,56.0891752391935,
57.0818127418655,58.0744502445374,59.0670877472094,59.6902604182061),
 .UNSPECIFIED.);
#2551=B_SPLINE_CURVE_WITH_KNOTS('',3,(#22349,#22350,#22351,#22352,#22353,
#22354,#22355,#22356,#22357,#22358),.UNSPECIFIED.,.F.,.F.,(4,1,1,1,1,1,
1,4),(47.1238898038469,47.5939389584978,48.5865764611697,49.5792139638417,
50.5718514665136,51.5644889691856,52.5571264718575,53.4070751110265),
 .UNSPECIFIED.);
#2552=B_SPLINE_CURVE_WITH_KNOTS('',3,(#22359,#22360,#22361,#22362,#22363,
#22364,#22365,#22366,#22367,#22368,#22369),.UNSPECIFIED.,.F.,.F.,(4,1,1,
1,1,1,1,1,4),(47.1238898038469,47.155437715146,48.148075217818,49.1407127204899,
50.1333502231619,51.1259877258338,52.1186252285057,53.1112627311777,53.4070751110265),
 .UNSPECIFIED.);
#2553=B_SPLINE_CURVE_WITH_KNOTS('',3,(#22374,#22375,#22376,#22377,#22378,
#22379,#22380,#22381,#22382,#22383),.UNSPECIFIED.,.F.,.F.,(4,1,1,1,1,1,
1,4),(40.8407044966673,41.6381139424661,42.6307514451381,43.62338894781,
44.616026450482,45.6086639531539,46.6013014558259,47.1238898038469),
 .UNSPECIFIED.);
#2554=B_SPLINE_CURVE_WITH_KNOTS('',3,(#22384,#22385,#22386,#22387,#22388,
#22389,#22390,#22391,#22392,#22393),.UNSPECIFIED.,.F.,.F.,(4,1,1,1,1,1,
1,4),(40.8407044966673,41.1996126991143,42.1922502017863,43.1848877044582,
44.1775252071302,45.1701627098021,46.1628002124741,47.1238898038469),
 .UNSPECIFIED.);
#2555=B_SPLINE_CURVE_WITH_KNOTS('',3,(#22398,#22399,#22400,#22401,#22402,
#22403,#22404,#22405,#22406,#22407,#22408),.UNSPECIFIED.,.F.,.F.,(4,1,1,
1,1,1,1,1,4),(34.5575191894877,34.6896514237625,35.6822889264345,36.6749264291064,
37.6675639317784,38.6602014344503,39.6528389371222,40.6454764397942,40.8407044966673),
 .UNSPECIFIED.);
#2556=B_SPLINE_CURVE_WITH_KNOTS('',3,(#22409,#22410,#22411,#22412,#22413,
#22414,#22415,#22416,#22417,#22418),.UNSPECIFIED.,.F.,.F.,(4,1,1,1,1,1,
1,4),(34.5575191894877,35.2437876830827,36.2364251857546,37.2290626884266,
38.2217001910985,39.2143376937705,40.2069751964424,40.8407044966673),
 .UNSPECIFIED.);
#2557=B_SPLINE_CURVE_WITH_KNOTS('',3,(#22423,#22424,#22425,#22426,#22427,
#22428,#22429,#22430,#22431,#22432),.UNSPECIFIED.,.F.,.F.,(4,1,1,1,1,1,
1,4),(28.2743338823081,28.7338264077309,29.7264639104028,30.7191014130747,
31.7117389157467,32.7043764184186,33.6970139210906,34.5575191894877),
 .UNSPECIFIED.);
#2558=B_SPLINE_CURVE_WITH_KNOTS('',3,(#22433,#22434,#22435,#22436,#22437,
#22438,#22439,#22440,#22441,#22442,#22443),.UNSPECIFIED.,.F.,.F.,(4,1,1,
1,1,1,1,1,4),(28.2743338823081,28.2953251643791,29.287962667051,30.280600169723,
31.2732376723949,32.2658751750668,33.2585126777388,34.2511501804107,34.5575191894877),
 .UNSPECIFIED.);
#2559=B_SPLINE_CURVE_WITH_KNOTS('',3,(#22448,#22449,#22450,#22451,#22452,
#22453,#22454,#22455,#22456,#22457),.UNSPECIFIED.,.F.,.F.,(4,1,1,1,1,1,
1,4),(21.9911485751285,22.7780013916992,23.7706388943711,24.7632763970431,
25.755913899715,26.748551402387,27.7411889050589,28.2743338823081),
 .UNSPECIFIED.);
#2560=B_SPLINE_CURVE_WITH_KNOTS('',3,(#22458,#22459,#22460,#22461,#22462,
#22463,#22464,#22465,#22466,#22467),.UNSPECIFIED.,.F.,.F.,(4,1,1,1,1,1,
1,4),(21.9911485751285,22.3395001483474,23.3321376510193,24.3247751536913,
25.3174126563632,26.3100501590352,27.3026876617071,28.2743338823081),
 .UNSPECIFIED.);
#2561=B_SPLINE_CURVE_WITH_KNOTS('',3,(#22473,#22474,#22475,#22476,#22477),
 .UNSPECIFIED.,.F.,.F.,(4,1,4),(14.3984001269718,15.3910376296438,15.7079632679489),
 .UNSPECIFIED.);
#2562=B_SPLINE_CURVE_WITH_KNOTS('',3,(#22480,#22481,#22482,#22483,#22484),
 .UNSPECIFIED.,.F.,.F.,(4,1,4),(13.8759337553362,14.8369013703236,15.7079632679489),
 .UNSPECIFIED.);
#2563=B_SPLINE_CURVE_WITH_KNOTS('',3,(#22490,#22491,#22492,#22493),
 .UNSPECIFIED.,.F.,.F.,(4,4),(57.8582309055934,58.5656126576448),
 .UNSPECIFIED.);
#2564=B_SPLINE_CURVE_WITH_KNOTS('',3,(#22501,#22502,#22503,#22504,#22505,
#22506,#22507,#22508,#22509,#22510),.UNSPECIFIED.,.F.,.F.,(4,3,3,4),(-56.5486677646163,
-55.5877001496289,-54.595062646957,-54.1144568630779),.UNSPECIFIED.);
#2565=B_SPLINE_CURVE_WITH_KNOTS('',3,(#22515,#22516,#22517,#22518,#22519,
#22520,#22521,#22522,#22523,#22524,#22525,#22526,#22527,#22528,#22529,#22530,
#22531,#22532,#22533,#22534,#22535,#22536,#22537,#22538,#22539),
 .UNSPECIFIED.,.F.,.F.,(4,3,3,3,3,3,3,3,4),(51.5750455984138,51.6171501389411,
52.6097876416131,53.602425144285,54.595062646957,55.5877001496289,56.5803376523009,
57.5729751549728,57.8582309055934),.UNSPECIFIED.);
#2566=B_SPLINE_CURVE_WITH_KNOTS('',3,(#22540,#22541,#22542,#22543,#22544,
#22545,#22546,#22547,#22548,#22549,#22550,#22551,#22552,#22553,#22554,#22555,
#22556,#22557,#22558,#22559,#22560,#22561),.UNSPECIFIED.,.F.,.F.,(4,3,3,
3,3,3,3,4),(-54.1144568630779,-53.602425144285,-52.6097876416131,-51.6171501389411,
-50.6245126362692,-49.6318751335972,-48.6392376309253,-47.8312715558983),
 .UNSPECIFIED.);
#2567=B_SPLINE_CURVE_WITH_KNOTS('',3,(#22566,#22567,#22568,#22569,#22570,
#22571,#22572,#22573,#22574,#22575,#22576,#22577,#22578,#22579,#22580,#22581,
#22582,#22583,#22584,#22585,#22586,#22587),.UNSPECIFIED.,.F.,.F.,(4,3,3,
3,3,3,3,4),(45.2918602912342,45.6613251229095,46.6539626255814,47.6466001282534,
48.6392376309253,49.6318751335972,50.6245126362692,51.5750455984138),
 .UNSPECIFIED.);
#2568=B_SPLINE_CURVE_WITH_KNOTS('',3,(#22588,#22589,#22590,#22591,#22592,
#22593,#22594,#22595,#22596,#22597,#22598,#22599,#22600,#22601,#22602,#22603,
#22604,#22605,#22606,#22607,#22608,#22609,#22610,#22611,#22612),
 .UNSPECIFIED.,.F.,.F.,(4,3,3,3,3,3,3,3,4),(-47.8312715558983,-47.6466001282533,
-46.6539626255814,-45.6613251229095,-44.6686876202375,-43.6760501175656,
-42.6834126148936,-41.6907751122217,-41.5480862487187),.UNSPECIFIED.);
#2569=B_SPLINE_CURVE_WITH_KNOTS('',3,(#22617,#22618,#22619,#22620,#22621,
#22622,#22623,#22624,#22625,#22626,#22627,#22628,#22629,#22630,#22631,#22632,
#22633,#22634,#22635,#22636,#22637,#22638),.UNSPECIFIED.,.F.,.F.,(4,3,3,
3,3,3,3,4),(39.0086749840546,39.7055001068778,40.6981376095497,41.6907751122217,
42.6834126148936,43.6760501175656,44.6686876202375,45.2918602912342),
 .UNSPECIFIED.);
#2570=B_SPLINE_CURVE_WITH_KNOTS('',3,(#22639,#22640,#22641,#22642,#22643,
#22644,#22645,#22646,#22647,#22648,#22649,#22650,#22651,#22652,#22653,#22654,
#22655,#22656,#22657,#22658,#22659,#22660),.UNSPECIFIED.,.F.,.F.,(4,3,3,
3,3,3,3,4),(-41.5480862487187,-40.6981376095497,-39.7055001068778,-38.7128626042058,
-37.7202251015339,-36.727587598862,-35.73495009619,-35.2649009415391),
 .UNSPECIFIED.);
#2571=B_SPLINE_CURVE_WITH_KNOTS('',3,(#22665,#22666,#22667,#22668,#22669,
#22670,#22671,#22672,#22673,#22674,#22675,#22676,#22677,#22678,#22679,#22680,
#22681,#22682,#22683,#22684,#22685,#22686,#22687,#22688,#22689),
 .UNSPECIFIED.,.F.,.F.,(4,3,3,3,3,3,3,3,4),(32.725489676875,32.7570375881742,
33.7496750908461,34.7423125935181,35.73495009619,36.727587598862,37.7202251015339,
38.7128626042059,39.0086749840546),.UNSPECIFIED.);
#2572=B_SPLINE_CURVE_WITH_KNOTS('',3,(#22690,#22691,#22692,#22693,#22694,
#22695,#22696,#22697,#22698,#22699,#22700,#22701,#22702,#22703,#22704,#22705,
#22706,#22707,#22708,#22709,#22710,#22711),.UNSPECIFIED.,.F.,.F.,(4,3,3,
3,3,3,3,4),(-35.2649009415391,-34.7423125935181,-33.7496750908461,-32.7570375881742,
-31.7644000855022,-30.7717625828303,-29.7791250801583,-28.9817156343595),
 .UNSPECIFIED.);
#2573=B_SPLINE_CURVE_WITH_KNOTS('',3,(#22716,#22717,#22718,#22719,#22720,
#22721,#22722,#22723,#22724,#22725,#22726,#22727,#22728,#22729,#22730,#22731,
#22732,#22733,#22734,#22735,#22736,#22737),.UNSPECIFIED.,.F.,.F.,(4,3,3,
3,3,3,3,4),(26.4423043696954,26.8012125721425,27.7938500748145,28.7864875774864,
29.7791250801583,30.7717625828303,31.7644000855022,32.725489676875),
 .UNSPECIFIED.);
#2574=B_SPLINE_CURVE_WITH_KNOTS('',3,(#22738,#22739,#22740,#22741,#22742,
#22743,#22744,#22745,#22746,#22747,#22748,#22749,#22750,#22751,#22752,#22753,
#22754,#22755,#22756,#22757,#22758,#22759,#22760,#22761,#22762),
 .UNSPECIFIED.,.F.,.F.,(4,3,3,3,3,3,3,3,4),(-28.9817156343595,-28.7864875774864,
-27.7938500748144,-26.8012125721425,-25.8085750694706,-24.8159375667986,
-23.8233000641267,-22.8306625614547,-22.6985303271799),.UNSPECIFIED.);
#2575=B_SPLINE_CURVE_WITH_KNOTS('',3,(#22767,#22768,#22769,#22770,#22771,
#22772,#22773,#22774,#22775,#22776,#22777,#22778,#22779,#22780,#22781,#22782,
#22783,#22784,#22785,#22786,#22787,#22788),.UNSPECIFIED.,.F.,.F.,(4,3,3,
3,3,3,3,4),(20.1591190625158,20.8453875561108,21.8380250587828,22.8306625614547,
23.8233000641267,24.8159375667986,25.8085750694706,26.4423043696954),
 .UNSPECIFIED.);
#2576=B_SPLINE_CURVE_WITH_KNOTS('',3,(#22789,#22790,#22791,#22792,#22793,
#22794,#22795,#22796,#22797,#22798,#22799,#22800,#22801,#22802,#22803,#22804,
#22805,#22806,#22807,#22808,#22809,#22810),.UNSPECIFIED.,.F.,.F.,(4,3,3,
3,3,3,3,4),(-22.6985303271799,-21.8380250587828,-20.8453875561108,-19.8527500534389,
-18.860112550767,-17.867475048095,-16.8748375454231,-16.4153450200003),
 .UNSPECIFIED.);
#2577=B_SPLINE_CURVE_WITH_KNOTS('',3,(#22815,#22816,#22817,#22818,#22819,
#22820,#22821,#22822,#22823,#22824,#22825,#22826,#22827,#22828,#22829,#22830,
#22831,#22832,#22833,#22834,#22835,#22836,#22837,#22838,#22839),
 .UNSPECIFIED.,.F.,.F.,(4,3,3,3,3,3,3,3,4),(13.8759337553363,13.8969250374072,
14.8895625400792,15.8822000427511,16.8748375454231,17.867475048095,18.860112550767,
19.8527500534389,20.1591190625158),.UNSPECIFIED.);
#2578=B_SPLINE_CURVE_WITH_KNOTS('',3,(#22840,#22841,#22842,#22843,#22844,
#22845,#22846,#22847,#22848,#22849,#22850,#22851,#22852,#22853,#22854,#22855,
#22856,#22857,#22858,#22859,#22860,#22861),.UNSPECIFIED.,.F.,.F.,(4,3,3,
3,3,3,3,4),(-16.4153450200003,-15.8822000427511,-14.8895625400792,-13.8969250374072,
-12.9042875347353,-11.9116500320633,-10.9190125293914,-10.1321597128207),
 .UNSPECIFIED.);
#2579=B_SPLINE_CURVE_WITH_KNOTS('',3,(#22867,#22868,#22869,#22870,#22871,
#22872,#22873,#22874,#22875,#22876,#22877,#22878,#22879),.UNSPECIFIED.,
 .F.,.F.,(4,3,3,3,4),(-3.84897440564114,-2.97791250801584,-1.98527500534389,
-0.992637502671945,0.),.UNSPECIFIED.);
#2580=B_SPLINE_CURVE_WITH_KNOTS('',3,(#22882,#22883,#22884,#22885,#22886,
#22887,#22888,#22889,#22890,#22891,#22892,#22893,#22894,#22895,#22896,#22897,
#22898,#22899,#22900),.UNSPECIFIED.,.F.,.F.,(4,3,3,3,3,3,4),(2.01694489302845,
2.97791250801584,3.97055001068778,4.96318751335972,5.95582501603167,6.94846251870361,
7.59274844815667),.UNSPECIFIED.);
#2581=B_SPLINE_CURVE_WITH_KNOTS('',3,(#22906,#22907,#22908,#22909,#22910,
#22911,#22912,#22913),.UNSPECIFIED.,.F.,.F.,(4,1,1,1,1,4),(65.9734457253856,
66.4540515092647,67.4466890119367,68.4393265146086,69.4319640172806,70.4246015199525),
 .UNSPECIFIED.);
#2582=B_SPLINE_CURVE_WITH_KNOTS('',3,(#22916,#22917,#22918,#22919,#22920,
#22921,#22922,#22923,#22924),.UNSPECIFIED.,.F.,.F.,(4,1,1,1,1,1,4),(65.9734457253856,
66.015550265913,67.0081877685849,68.0008252712569,68.9934627739288,69.9861002766008,
70.9470678915881),.UNSPECIFIED.);
#2583=B_SPLINE_CURVE_WITH_KNOTS('',3,(#22929,#22930,#22931,#22932,#22933,
#22934,#22935,#22936,#22937,#22938),.UNSPECIFIED.,.F.,.F.,(4,1,1,1,1,1,
1,4),(59.690260418206,60.4982264932331,61.490863995905,62.483501498577,
63.4761390012489,64.4687765039209,65.4614140065928,65.9734457253856),
 .UNSPECIFIED.);
#2584=B_SPLINE_CURVE_WITH_KNOTS('',3,(#22939,#22940,#22941,#22942,#22943,
#22944,#22945,#22946,#22947,#22948),.UNSPECIFIED.,.F.,.F.,(4,1,1,1,1,1,
1,4),(59.6902604182061,60.0597252498813,61.0523627525533,62.0450002552252,
63.0376377578971,64.0302752605691,65.022912763241,65.9734457253856),
 .UNSPECIFIED.);
#2585=B_SPLINE_CURVE_WITH_KNOTS('',3,(#22953,#22954,#22955,#22956,#22957,
#22958,#22959,#22960,#22961,#22962,#22963),.UNSPECIFIED.,.F.,.F.,(4,1,1,
1,1,1,1,1,4),(53.4070751110265,53.5497639745295,54.5424014772014,55.5350389798734,
56.5276764825453,57.5203139852172,58.5129514878892,59.5055889905611,59.690260418206),
 .UNSPECIFIED.);
#2586=B_SPLINE_CURVE_WITH_KNOTS('',3,(#22964,#22965,#22966,#22967,#22968,
#22969,#22970,#22971,#22972,#22973),.UNSPECIFIED.,.F.,.F.,(4,1,1,1,1,1,
1,4),(53.4070751110265,54.1039002338496,55.0965377365216,56.0891752391935,
57.0818127418655,58.0744502445374,59.0670877472094,59.6902604182061),
 .UNSPECIFIED.);
#2587=B_SPLINE_CURVE_WITH_KNOTS('',3,(#22978,#22979,#22980,#22981,#22982,
#22983,#22984,#22985,#22986,#22987),.UNSPECIFIED.,.F.,.F.,(4,1,1,1,1,1,
1,4),(47.1238898038469,47.5939389584978,48.5865764611697,49.5792139638417,
50.5718514665136,51.5644889691856,52.5571264718575,53.4070751110265),
 .UNSPECIFIED.);
#2588=B_SPLINE_CURVE_WITH_KNOTS('',3,(#22988,#22989,#22990,#22991,#22992,
#22993,#22994,#22995,#22996,#22997,#22998),.UNSPECIFIED.,.F.,.F.,(4,1,1,
1,1,1,1,1,4),(47.1238898038469,47.155437715146,48.148075217818,49.1407127204899,
50.1333502231619,51.1259877258338,52.1186252285057,53.1112627311777,53.4070751110265),
 .UNSPECIFIED.);
#2589=B_SPLINE_CURVE_WITH_KNOTS('',3,(#23003,#23004,#23005,#23006,#23007,
#23008,#23009,#23010,#23011,#23012),.UNSPECIFIED.,.F.,.F.,(4,1,1,1,1,1,
1,4),(40.8407044966673,41.6381139424661,42.6307514451381,43.62338894781,
44.616026450482,45.6086639531539,46.6013014558259,47.1238898038469),
 .UNSPECIFIED.);
#2590=B_SPLINE_CURVE_WITH_KNOTS('',3,(#23013,#23014,#23015,#23016,#23017,
#23018,#23019,#23020,#23021,#23022),.UNSPECIFIED.,.F.,.F.,(4,1,1,1,1,1,
1,4),(40.8407044966673,41.1996126991143,42.1922502017863,43.1848877044582,
44.1775252071302,45.1701627098021,46.1628002124741,47.1238898038469),
 .UNSPECIFIED.);
#2591=B_SPLINE_CURVE_WITH_KNOTS('',3,(#23027,#23028,#23029,#23030,#23031,
#23032,#23033,#23034,#23035,#23036,#23037),.UNSPECIFIED.,.F.,.F.,(4,1,1,
1,1,1,1,1,4),(34.5575191894877,34.6896514237625,35.6822889264345,36.6749264291064,
37.6675639317784,38.6602014344503,39.6528389371222,40.6454764397942,40.8407044966673),
 .UNSPECIFIED.);
#2592=B_SPLINE_CURVE_WITH_KNOTS('',3,(#23038,#23039,#23040,#23041,#23042,
#23043,#23044,#23045,#23046,#23047),.UNSPECIFIED.,.F.,.F.,(4,1,1,1,1,1,
1,4),(34.5575191894877,35.2437876830827,36.2364251857546,37.2290626884266,
38.2217001910985,39.2143376937705,40.2069751964424,40.8407044966673),
 .UNSPECIFIED.);
#2593=B_SPLINE_CURVE_WITH_KNOTS('',3,(#23052,#23053,#23054,#23055,#23056,
#23057,#23058,#23059,#23060,#23061),.UNSPECIFIED.,.F.,.F.,(4,1,1,1,1,1,
1,4),(28.2743338823081,28.7338264077309,29.7264639104028,30.7191014130747,
31.7117389157467,32.7043764184186,33.6970139210906,34.5575191894877),
 .UNSPECIFIED.);
#2594=B_SPLINE_CURVE_WITH_KNOTS('',3,(#23062,#23063,#23064,#23065,#23066,
#23067,#23068,#23069,#23070,#23071,#23072),.UNSPECIFIED.,.F.,.F.,(4,1,1,
1,1,1,1,1,4),(28.2743338823081,28.2953251643791,29.287962667051,30.280600169723,
31.2732376723949,32.2658751750668,33.2585126777388,34.2511501804107,34.5575191894877),
 .UNSPECIFIED.);
#2595=B_SPLINE_CURVE_WITH_KNOTS('',3,(#23077,#23078,#23079,#23080,#23081,
#23082,#23083,#23084,#23085,#23086),.UNSPECIFIED.,.F.,.F.,(4,1,1,1,1,1,
1,4),(21.9911485751285,22.7780013916992,23.7706388943711,24.7632763970431,
25.755913899715,26.748551402387,27.7411889050589,28.2743338823081),
 .UNSPECIFIED.);
#2596=B_SPLINE_CURVE_WITH_KNOTS('',3,(#23087,#23088,#23089,#23090,#23091,
#23092,#23093,#23094,#23095,#23096),.UNSPECIFIED.,.F.,.F.,(4,1,1,1,1,1,
1,4),(21.9911485751285,22.3395001483474,23.3321376510193,24.3247751536913,
25.3174126563632,26.3100501590352,27.3026876617071,28.2743338823081),
 .UNSPECIFIED.);
#2597=B_SPLINE_CURVE_WITH_KNOTS('',3,(#23102,#23103,#23104,#23105,#23106),
 .UNSPECIFIED.,.F.,.F.,(4,1,4),(14.3984001269718,15.3910376296438,15.7079632679489),
 .UNSPECIFIED.);
#2598=B_SPLINE_CURVE_WITH_KNOTS('',3,(#23109,#23110,#23111,#23112,#23113),
 .UNSPECIFIED.,.F.,.F.,(4,1,4),(13.8759337553362,14.8369013703236,15.7079632679489),
 .UNSPECIFIED.);
#2599=B_SPLINE_CURVE_WITH_KNOTS('',3,(#23119,#23120,#23121,#23122),
 .UNSPECIFIED.,.F.,.F.,(4,4),(57.8582309055934,58.5656126576447),
 .UNSPECIFIED.);
#2600=B_SPLINE_CURVE_WITH_KNOTS('',3,(#23130,#23131,#23132,#23133,#23134,
#23135,#23136,#23137,#23138,#23139),.UNSPECIFIED.,.F.,.F.,(4,3,3,4),(-56.5486677646163,
-55.5877001496289,-54.595062646957,-54.1144568630778),.UNSPECIFIED.);
#2601=B_SPLINE_CURVE_WITH_KNOTS('',3,(#23144,#23145,#23146,#23147,#23148,
#23149,#23150,#23151,#23152,#23153,#23154,#23155,#23156,#23157,#23158,#23159,
#23160,#23161,#23162,#23163,#23164,#23165,#23166,#23167,#23168),
 .UNSPECIFIED.,.F.,.F.,(4,3,3,3,3,3,3,3,4),(51.5750455984138,51.6171501389411,
52.6097876416131,53.602425144285,54.595062646957,55.5877001496289,56.5803376523009,
57.5729751549728,57.8582309055934),.UNSPECIFIED.);
#2602=B_SPLINE_CURVE_WITH_KNOTS('',3,(#23169,#23170,#23171,#23172,#23173,
#23174,#23175,#23176,#23177,#23178,#23179,#23180,#23181,#23182,#23183,#23184,
#23185,#23186,#23187,#23188,#23189,#23190),.UNSPECIFIED.,.F.,.F.,(4,3,3,
3,3,3,3,4),(-54.1144568630778,-53.602425144285,-52.6097876416131,-51.6171501389411,
-50.6245126362692,-49.6318751335972,-48.6392376309253,-47.8312715558982),
 .UNSPECIFIED.);
#2603=B_SPLINE_CURVE_WITH_KNOTS('',3,(#23195,#23196,#23197,#23198,#23199,
#23200,#23201,#23202,#23203,#23204,#23205,#23206,#23207,#23208,#23209,#23210,
#23211,#23212,#23213,#23214,#23215,#23216),.UNSPECIFIED.,.F.,.F.,(4,3,3,
3,3,3,3,4),(45.2918602912342,45.6613251229095,46.6539626255814,47.6466001282534,
48.6392376309253,49.6318751335972,50.6245126362692,51.5750455984138),
 .UNSPECIFIED.);
#2604=B_SPLINE_CURVE_WITH_KNOTS('',3,(#23217,#23218,#23219,#23220,#23221,
#23222,#23223,#23224,#23225,#23226,#23227,#23228,#23229,#23230,#23231,#23232,
#23233,#23234,#23235,#23236,#23237,#23238,#23239,#23240,#23241),
 .UNSPECIFIED.,.F.,.F.,(4,3,3,3,3,3,3,3,4),(-47.8312715558982,-47.6466001282533,
-46.6539626255814,-45.6613251229095,-44.6686876202375,-43.6760501175656,
-42.6834126148936,-41.6907751122217,-41.5480862487187),.UNSPECIFIED.);
#2605=B_SPLINE_CURVE_WITH_KNOTS('',3,(#23246,#23247,#23248,#23249,#23250,
#23251,#23252,#23253,#23254,#23255,#23256,#23257,#23258,#23259,#23260,#23261,
#23262,#23263,#23264,#23265,#23266,#23267),.UNSPECIFIED.,.F.,.F.,(4,3,3,
3,3,3,3,4),(39.0086749840546,39.7055001068778,40.6981376095497,41.6907751122217,
42.6834126148936,43.6760501175656,44.6686876202375,45.2918602912342),
 .UNSPECIFIED.);
#2606=B_SPLINE_CURVE_WITH_KNOTS('',3,(#23268,#23269,#23270,#23271,#23272,
#23273,#23274,#23275,#23276,#23277,#23278,#23279,#23280,#23281,#23282,#23283,
#23284,#23285,#23286,#23287,#23288,#23289),.UNSPECIFIED.,.F.,.F.,(4,3,3,
3,3,3,3,4),(-41.5480862487187,-40.6981376095497,-39.7055001068778,-38.7128626042058,
-37.7202251015339,-36.727587598862,-35.73495009619,-35.2649009415391),
 .UNSPECIFIED.);
#2607=B_SPLINE_CURVE_WITH_KNOTS('',3,(#23294,#23295,#23296,#23297,#23298,
#23299,#23300,#23301,#23302,#23303,#23304,#23305,#23306,#23307,#23308,#23309,
#23310,#23311,#23312,#23313,#23314,#23315,#23316,#23317,#23318),
 .UNSPECIFIED.,.F.,.F.,(4,3,3,3,3,3,3,3,4),(32.725489676875,32.7570375881742,
33.7496750908461,34.7423125935181,35.73495009619,36.727587598862,37.7202251015339,
38.7128626042059,39.0086749840546),.UNSPECIFIED.);
#2608=B_SPLINE_CURVE_WITH_KNOTS('',3,(#23319,#23320,#23321,#23322,#23323,
#23324,#23325,#23326,#23327,#23328,#23329,#23330,#23331,#23332,#23333,#23334,
#23335,#23336,#23337,#23338,#23339,#23340),.UNSPECIFIED.,.F.,.F.,(4,3,3,
3,3,3,3,4),(-35.2649009415391,-34.7423125935181,-33.7496750908461,-32.7570375881742,
-31.7644000855022,-30.7717625828303,-29.7791250801584,-28.9817156343595),
 .UNSPECIFIED.);
#2609=B_SPLINE_CURVE_WITH_KNOTS('',3,(#23345,#23346,#23347,#23348,#23349,
#23350,#23351,#23352,#23353,#23354,#23355,#23356,#23357,#23358,#23359,#23360,
#23361,#23362,#23363,#23364,#23365,#23366),.UNSPECIFIED.,.F.,.F.,(4,3,3,
3,3,3,3,4),(26.4423043696954,26.8012125721425,27.7938500748145,28.7864875774864,
29.7791250801584,30.7717625828303,31.7644000855022,32.725489676875),
 .UNSPECIFIED.);
#2610=B_SPLINE_CURVE_WITH_KNOTS('',3,(#23367,#23368,#23369,#23370,#23371,
#23372,#23373,#23374,#23375,#23376,#23377,#23378,#23379,#23380,#23381,#23382,
#23383,#23384,#23385,#23386,#23387,#23388,#23389,#23390,#23391),
 .UNSPECIFIED.,.F.,.F.,(4,3,3,3,3,3,3,3,4),(-28.9817156343595,-28.7864875774864,
-27.7938500748145,-26.8012125721425,-25.8085750694706,-24.8159375667986,
-23.8233000641267,-22.8306625614547,-22.6985303271799),.UNSPECIFIED.);
#2611=B_SPLINE_CURVE_WITH_KNOTS('',3,(#23396,#23397,#23398,#23399,#23400,
#23401,#23402,#23403,#23404,#23405,#23406,#23407,#23408,#23409,#23410,#23411,
#23412,#23413,#23414,#23415,#23416,#23417),.UNSPECIFIED.,.F.,.F.,(4,3,3,
3,3,3,3,4),(20.1591190625158,20.8453875561108,21.8380250587828,22.8306625614547,
23.8233000641267,24.8159375667986,25.8085750694706,26.4423043696954),
 .UNSPECIFIED.);
#2612=B_SPLINE_CURVE_WITH_KNOTS('',3,(#23418,#23419,#23420,#23421,#23422,
#23423,#23424,#23425,#23426,#23427,#23428,#23429,#23430,#23431,#23432,#23433,
#23434,#23435,#23436,#23437,#23438,#23439),.UNSPECIFIED.,.F.,.F.,(4,3,3,
3,3,3,3,4),(-22.6985303271799,-21.8380250587828,-20.8453875561108,-19.8527500534389,
-18.8601125507669,-17.867475048095,-16.8748375454231,-16.4153450200003),
 .UNSPECIFIED.);
#2613=B_SPLINE_CURVE_WITH_KNOTS('',3,(#23444,#23445,#23446,#23447,#23448,
#23449,#23450,#23451,#23452,#23453,#23454,#23455,#23456,#23457,#23458,#23459,
#23460,#23461,#23462,#23463,#23464,#23465,#23466,#23467,#23468),
 .UNSPECIFIED.,.F.,.F.,(4,3,3,3,3,3,3,3,4),(13.8759337553363,13.8969250374072,
14.8895625400792,15.8822000427511,16.8748375454231,17.867475048095,18.860112550767,
19.8527500534389,20.1591190625158),.UNSPECIFIED.);
#2614=B_SPLINE_CURVE_WITH_KNOTS('',3,(#23469,#23470,#23471,#23472,#23473,
#23474,#23475,#23476,#23477,#23478,#23479,#23480,#23481,#23482,#23483,#23484,
#23485,#23486,#23487,#23488,#23489,#23490),.UNSPECIFIED.,.F.,.F.,(4,3,3,
3,3,3,3,4),(-16.4153450200003,-15.8822000427511,-14.8895625400792,-13.8969250374072,
-12.9042875347353,-11.9116500320633,-10.9190125293914,-10.1321597128207),
 .UNSPECIFIED.);
#2615=B_SPLINE_CURVE_WITH_KNOTS('',3,(#23496,#23497,#23498,#23499,#23500,
#23501,#23502,#23503,#23504,#23505,#23506,#23507,#23508),.UNSPECIFIED.,
 .F.,.F.,(4,3,3,3,4),(-3.84897440564114,-2.97791250801583,-1.98527500534389,
-0.992637502671944,0.),.UNSPECIFIED.);
#2616=B_SPLINE_CURVE_WITH_KNOTS('',3,(#23511,#23512,#23513,#23514,#23515,
#23516,#23517,#23518,#23519,#23520,#23521,#23522,#23523,#23524,#23525,#23526,
#23527,#23528,#23529),.UNSPECIFIED.,.F.,.F.,(4,3,3,3,3,3,4),(2.01694489302844,
2.97791250801584,3.97055001068778,4.96318751335973,5.95582501603167,6.94846251870362,
7.59274844815667),.UNSPECIFIED.);
#2617=B_SPLINE_CURVE_WITH_KNOTS('',3,(#23535,#23536,#23537,#23538,#23539,
#23540,#23541,#23542),.UNSPECIFIED.,.F.,.F.,(4,1,1,1,1,4),(65.9734457253856,
66.4540515092648,67.4466890119367,68.4393265146086,69.4319640172806,70.4246015199525),
 .UNSPECIFIED.);
#2618=B_SPLINE_CURVE_WITH_KNOTS('',3,(#23545,#23546,#23547,#23548,#23549,
#23550,#23551,#23552,#23553),.UNSPECIFIED.,.F.,.F.,(4,1,1,1,1,1,4),(65.9734457253856,
66.015550265913,67.0081877685849,68.0008252712568,68.9934627739288,69.9861002766007,
70.9470678915881),.UNSPECIFIED.);
#2619=B_SPLINE_CURVE_WITH_KNOTS('',3,(#23558,#23559,#23560,#23561,#23562,
#23563,#23564,#23565,#23566,#23567),.UNSPECIFIED.,.F.,.F.,(4,1,1,1,1,1,
1,4),(59.6902604182061,60.4982264932331,61.490863995905,62.483501498577,
63.4761390012489,64.4687765039209,65.4614140065928,65.9734457253856),
 .UNSPECIFIED.);
#2620=B_SPLINE_CURVE_WITH_KNOTS('',3,(#23568,#23569,#23570,#23571,#23572,
#23573,#23574,#23575,#23576,#23577),.UNSPECIFIED.,.F.,.F.,(4,1,1,1,1,1,
1,4),(59.6902604182061,60.0597252498813,61.0523627525532,62.0450002552252,
63.0376377578971,64.0302752605691,65.022912763241,65.9734457253856),
 .UNSPECIFIED.);
#2621=B_SPLINE_CURVE_WITH_KNOTS('',3,(#23582,#23583,#23584,#23585,#23586,
#23587,#23588,#23589,#23590,#23591,#23592),.UNSPECIFIED.,.F.,.F.,(4,1,1,
1,1,1,1,1,4),(53.4070751110265,53.5497639745295,54.5424014772014,55.5350389798734,
56.5276764825453,57.5203139852172,58.5129514878892,59.5055889905611,59.6902604182061),
 .UNSPECIFIED.);
#2622=B_SPLINE_CURVE_WITH_KNOTS('',3,(#23593,#23594,#23595,#23596,#23597,
#23598,#23599,#23600,#23601,#23602),.UNSPECIFIED.,.F.,.F.,(4,1,1,1,1,1,
1,4),(53.4070751110265,54.1039002338496,55.0965377365216,56.0891752391935,
57.0818127418655,58.0744502445374,59.0670877472093,59.6902604182061),
 .UNSPECIFIED.);
#2623=B_SPLINE_CURVE_WITH_KNOTS('',3,(#23607,#23608,#23609,#23610,#23611,
#23612,#23613,#23614,#23615,#23616),.UNSPECIFIED.,.F.,.F.,(4,1,1,1,1,1,
1,4),(47.1238898038469,47.5939389584978,48.5865764611697,49.5792139638417,
50.5718514665136,51.5644889691856,52.5571264718575,53.4070751110265),
 .UNSPECIFIED.);
#2624=B_SPLINE_CURVE_WITH_KNOTS('',3,(#23617,#23618,#23619,#23620,#23621,
#23622,#23623,#23624,#23625,#23626,#23627),.UNSPECIFIED.,.F.,.F.,(4,1,1,
1,1,1,1,1,4),(47.1238898038469,47.155437715146,48.1480752178179,49.1407127204899,
50.1333502231618,51.1259877258338,52.1186252285057,53.1112627311777,53.4070751110265),
 .UNSPECIFIED.);
#2625=B_SPLINE_CURVE_WITH_KNOTS('',3,(#23632,#23633,#23634,#23635,#23636,
#23637,#23638,#23639,#23640,#23641),.UNSPECIFIED.,.F.,.F.,(4,1,1,1,1,1,
1,4),(40.8407044966673,41.6381139424661,42.6307514451381,43.62338894781,
44.616026450482,45.6086639531539,46.6013014558259,47.1238898038469),
 .UNSPECIFIED.);
#2626=B_SPLINE_CURVE_WITH_KNOTS('',3,(#23642,#23643,#23644,#23645,#23646,
#23647,#23648,#23649,#23650,#23651),.UNSPECIFIED.,.F.,.F.,(4,1,1,1,1,1,
1,4),(40.8407044966673,41.1996126991143,42.1922502017863,43.1848877044582,
44.1775252071302,45.1701627098021,46.1628002124741,47.1238898038469),
 .UNSPECIFIED.);
#2627=B_SPLINE_CURVE_WITH_KNOTS('',3,(#23656,#23657,#23658,#23659,#23660,
#23661,#23662,#23663,#23664,#23665,#23666),.UNSPECIFIED.,.F.,.F.,(4,1,1,
1,1,1,1,1,4),(34.5575191894877,34.6896514237625,35.6822889264345,36.6749264291064,
37.6675639317784,38.6602014344503,39.6528389371222,40.6454764397942,40.8407044966673),
 .UNSPECIFIED.);
#2628=B_SPLINE_CURVE_WITH_KNOTS('',3,(#23667,#23668,#23669,#23670,#23671,
#23672,#23673,#23674,#23675,#23676),.UNSPECIFIED.,.F.,.F.,(4,1,1,1,1,1,
1,4),(34.5575191894877,35.2437876830827,36.2364251857546,37.2290626884266,
38.2217001910985,39.2143376937704,40.2069751964424,40.8407044966673),
 .UNSPECIFIED.);
#2629=B_SPLINE_CURVE_WITH_KNOTS('',3,(#23681,#23682,#23683,#23684,#23685,
#23686,#23687,#23688,#23689,#23690),.UNSPECIFIED.,.F.,.F.,(4,1,1,1,1,1,
1,4),(28.2743338823081,28.7338264077309,29.7264639104028,30.7191014130747,
31.7117389157467,32.7043764184186,33.6970139210906,34.5575191894877),
 .UNSPECIFIED.);
#2630=B_SPLINE_CURVE_WITH_KNOTS('',3,(#23691,#23692,#23693,#23694,#23695,
#23696,#23697,#23698,#23699,#23700,#23701),.UNSPECIFIED.,.F.,.F.,(4,1,1,
1,1,1,1,1,4),(28.2743338823081,28.2953251643791,29.287962667051,30.2806001697229,
31.2732376723949,32.2658751750668,33.2585126777388,34.2511501804107,34.5575191894877),
 .UNSPECIFIED.);
#2631=B_SPLINE_CURVE_WITH_KNOTS('',3,(#23706,#23707,#23708,#23709,#23710,
#23711,#23712,#23713,#23714,#23715),.UNSPECIFIED.,.F.,.F.,(4,1,1,1,1,1,
1,4),(21.9911485751285,22.7780013916992,23.7706388943711,24.7632763970431,
25.755913899715,26.748551402387,27.7411889050589,28.2743338823081),
 .UNSPECIFIED.);
#2632=B_SPLINE_CURVE_WITH_KNOTS('',3,(#23716,#23717,#23718,#23719,#23720,
#23721,#23722,#23723,#23724,#23725),.UNSPECIFIED.,.F.,.F.,(4,1,1,1,1,1,
1,4),(21.9911485751285,22.3395001483474,23.3321376510193,24.3247751536913,
25.3174126563632,26.3100501590352,27.3026876617071,28.2743338823081),
 .UNSPECIFIED.);
#2633=B_SPLINE_CURVE_WITH_KNOTS('',3,(#23731,#23732,#23733,#23734,#23735),
 .UNSPECIFIED.,.F.,.F.,(4,1,4),(14.3984001269718,15.3910376296438,15.7079632679489),
 .UNSPECIFIED.);
#2634=B_SPLINE_CURVE_WITH_KNOTS('',3,(#23738,#23739,#23740,#23741,#23742),
 .UNSPECIFIED.,.F.,.F.,(4,1,4),(13.8759337553362,14.8369013703236,15.7079632679489),
 .UNSPECIFIED.);
#2635=B_SPLINE_CURVE_WITH_KNOTS('',3,(#23796,#23797,#23798,#23799,#23800,
#23801,#23802,#23803,#23804,#23805,#23806,#23807,#23808,#23809,#23810,#23811,
#23812,#23813,#23814,#23815,#23816,#23817,#23818,#23819,#23820,#23821,#23822,
#23823,#23824,#23825,#23826,#23827,#23828,#23829,#23830,#23831,#23832,#23833,
#23834,#23835,#23836,#23837,#23838,#23839,#23840,#23841,#23842,#23843,#23844,
#23845,#23846,#23847,#23848,#23849,#23850,#23851,#23852,#23853,#23854,#23855,
#23856,#23857,#23858,#23859,#23860,#23861,#23862,#23863,#23864,#23865,#23866,
#23867,#23868,#23869,#23870,#23871,#23872,#23873,#23874,#23875,#23876,#23877,
#23878,#23879,#23880,#23881,#23882,#23883,#23884,#23885,#23886,#23887,#23888,
#23889),.UNSPECIFIED.,.F.,.F.,(4,3,3,3,3,3,3,3,3,3,3,3,3,3,3,3,3,3,3,3,
3,3,3,3,3,3,3,3,3,3,3,4),(-0.569248610399519,-0.543573521275112,-0.517270334894588,
-0.510403597501912,-0.504800301943937,-0.477738562936544,-0.455893959419014,
-0.447075871895859,-0.442407285930102,-0.414674892956538,-0.386513329416069,
-0.358572400845104,-0.344674734332904,-0.340104787267607,-0.311173962811257,
-0.302981734796303,-0.275165122896056,-0.246719621409672,-0.236777833320522,
-0.231757247321404,-0.227578652734185,-0.198579230964211,-0.169010642259111,
-0.139211776300183,-0.123031160575437,-0.117998606549764,-0.113391716242956,
-0.0828441510686728,-0.0522701024998839,-0.0223137899294547,-0.00976685050221584,
0.),.UNSPECIFIED.);
#2636=B_SPLINE_CURVE_WITH_KNOTS('',3,(#23890,#23891,#23892,#23893,#23894,
#23895,#23896,#23897,#23898,#23899,#23900,#23901,#23902,#23903,#23904,#23905,
#23906,#23907,#23908,#23909,#23910,#23911,#23912,#23913,#23914,#23915,#23916,
#23917,#23918,#23919,#23920,#23921,#23922,#23923,#23924,#23925,#23926,#23927,
#23928,#23929,#23930,#23931,#23932,#23933,#23934,#23935,#23936,#23937,#23938,
#23939,#23940,#23941,#23942,#23943,#23944,#23945,#23946,#23947,#23948,#23949,
#23950,#23951,#23952,#23953,#23954,#23955,#23956,#23957,#23958,#23959,#23960,
#23961,#23962,#23963,#23964,#23965,#23966,#23967,#23968,#23969,#23970,#23971,
#23972,#23973,#23974,#23975,#23976,#23977,#23978,#23979,#23980,#23981,#23982,
#23983),.UNSPECIFIED.,.F.,.F.,(4,3,3,3,3,3,3,3,3,3,3,3,3,3,3,3,3,3,3,3,
3,3,3,3,3,3,3,3,3,3,3,4),(-0.566847306048109,-0.536665088445275,-0.506058869929166,
-0.497416819810769,-0.490479649741127,-0.46033271574735,-0.437086681478693,
-0.424703687019547,-0.42046272258324,-0.391037834184797,-0.361869486038122,
-0.333545859254429,-0.318750504840346,-0.313020117693916,-0.30866018151949,
-0.280670752475326,-0.274364441598099,-0.245887082813539,-0.21615615821092,
-0.204673879614289,-0.200549632065964,-0.172713962599083,-0.14494922019829,
-0.117659631761598,-0.103957138540472,-0.0999252379237537,-0.0958138251359032,
-0.0691413140129682,-0.0429166578991969,-0.017493208914001,-0.00803968599259055,
0.),.UNSPECIFIED.);
#2637=B_SPLINE_CURVE_WITH_KNOTS('',3,(#23985,#23986,#23987,#23988,#23989,
#23990,#23991,#23992,#23993,#23994,#23995),.UNSPECIFIED.,.F.,.F.,(4,1,1,
1,1,1,1,1,4),(15.7079632679489,15.8295388729956,16.8221763756675,17.8148138783395,
18.8074513810114,19.8000888836834,20.7927263863553,21.7853638890272,21.9911485751285),
 .UNSPECIFIED.);
#2638=B_SPLINE_CURVE_WITH_KNOTS('',3,(#23996,#23997,#23998,#23999,#24000,
#24001,#24002,#24003,#24004,#24005),.UNSPECIFIED.,.F.,.F.,(4,1,1,1,1,1,
1,4),(15.7079632679489,16.3836751323157,17.3763126349877,18.3689501376596,
19.3615876403316,20.3542251430035,21.3468626456754,21.9911485751285),
 .UNSPECIFIED.);
#2639=B_SPLINE_CURVE_WITH_KNOTS('',3,(#24254,#24255,#24256,#24257,#24258,
#24259,#24260,#24261,#24262,#24263,#24264,#24265,#24266,#24267,#24268,#24269,
#24270,#24271,#24272,#24273,#24274,#24275,#24276,#24277,#24278,#24279,#24280,
#24281,#24282,#24283,#24284,#24285,#24286,#24287,#24288,#24289,#24290,#24291,
#24292,#24293,#24294,#24295,#24296,#24297,#24298,#24299,#24300,#24301,#24302,
#24303,#24304,#24305,#24306,#24307,#24308,#24309,#24310,#24311,#24312,#24313,
#24314,#24315,#24316,#24317,#24318,#24319,#24320,#24321,#24322,#24323,#24324,
#24325,#24326,#24327,#24328,#24329,#24330,#24331,#24332,#24333,#24334,#24335,
#24336,#24337,#24338,#24339,#24340,#24341,#24342,#24343,#24344),
 .UNSPECIFIED.,.F.,.F.,(4,3,3,3,3,3,3,3,3,3,3,3,3,3,3,3,3,3,3,3,3,3,3,3,
3,3,3,3,3,3,4),(0.,0.025364227043299,0.0513999158242781,0.0781558845304562,
0.0899177963079168,0.0966255877899614,0.102679521308728,0.129980995912345,
0.157733300312116,0.184661891602512,0.195928358257316,0.202971023563161,
0.20709884911213,0.236273257292916,0.265447665473703,0.293340547237465,
0.302677560574438,0.308745297675078,0.31452875584614,0.34260671879725,0.371727098701369,
0.401175544565762,0.421351009768009,0.42675374067059,0.456805248025141,
0.481883952215566,0.490048831459895,0.498378778112269,0.528887549635078,
0.557120064786841,0.566847306048159),.UNSPECIFIED.);
#2640=B_SPLINE_CURVE_WITH_KNOTS('',3,(#24345,#24346,#24347,#24348,#24349,
#24350,#24351,#24352,#24353,#24354,#24355,#24356,#24357,#24358,#24359,#24360,
#24361,#24362,#24363,#24364,#24365,#24366,#24367,#24368,#24369),
 .UNSPECIFIED.,.F.,.F.,(4,3,3,3,3,3,3,3,4),(-10.1321597128207,-9.92637502671944,
-8.9337375240475,-7.94110002137556,-6.94846251870361,-5.95582501603167,
-4.96318751335973,-3.97055001068778,-3.84897440564114),.UNSPECIFIED.);
#2641=B_SPLINE_CURVE_WITH_KNOTS('',3,(#24618,#24619,#24620,#24621,#24622,
#24623,#24624,#24625,#24626,#24627,#24628,#24629,#24630,#24631,#24632,#24633,
#24634,#24635,#24636,#24637,#24638,#24639),.UNSPECIFIED.,.F.,.F.,(4,3,3,
3,3,3,3,4),(7.59274844815667,7.94110002137556,8.9337375240475,9.92637502671945,
10.9190125293914,11.9116500320633,12.9042875347353,13.8759337553363),
 .UNSPECIFIED.);
#2642=B_SPLINE_CURVE_WITH_KNOTS('',3,(#24640,#24641,#24642,#24643,#24644,
#24645,#24646,#24647,#24648,#24649,#24650,#24651,#24652,#24653,#24654,#24655,
#24656,#24657,#24658,#24659,#24660,#24661,#24662,#24663,#24664,#24665,#24666,
#24667,#24668,#24669,#24670,#24671,#24672,#24673,#24674,#24675,#24676,#24677,
#24678,#24679,#24680,#24681,#24682,#24683,#24684,#24685,#24686,#24687,#24688,
#24689,#24690,#24691,#24692,#24693,#24694,#24695,#24696,#24697,#24698,#24699,
#24700,#24701,#24702,#24703,#24704,#24705,#24706,#24707,#24708,#24709,#24710,
#24711,#24712,#24713,#24714,#24715,#24716,#24717,#24718,#24719,#24720,#24721,
#24722,#24723,#24724,#24725,#24726,#24727,#24728,#24729,#24730),
 .UNSPECIFIED.,.F.,.F.,(4,3,3,3,3,3,3,3,3,3,3,3,3,3,3,3,3,3,3,3,3,3,3,3,
3,3,3,3,3,3,4),(0.,0.0297250789974743,0.0601087924509222,0.0893485781496982,
0.114933390636127,0.120627516286913,0.150386820364465,0.179982109044272,
0.208493351293487,0.220471801725418,0.228882355327184,0.234177134950228,
0.264102106495679,0.29200679839712,0.29402707804113,0.322973448322085,0.339362620925793,
0.343535829100154,0.371629352207137,0.399767745756159,0.427502104297442,
0.437970824675921,0.445641165257623,0.450375052516567,0.478076743972786,
0.498853012564951,0.508250460865973,0.513369595206828,0.539284549530519,
0.561181818341445,0.569248610399484),.UNSPECIFIED.);
#2643=B_SPLINE_CURVE_WITH_KNOTS('',3,(#24733,#24734,#24735,#24736,#24737,
#24738,#24739,#24740,#24741,#24742,#24743,#24744,#24745,#24746,#24747,#24748,
#24749,#24750,#24751,#24752,#24753,#24754,#24755,#24756,#24757,#24758,#24759,
#24760,#24761,#24762,#24763,#24764,#24765,#24766,#24767,#24768,#24769,#24770,
#24771,#24772,#24773,#24774,#24775,#24776,#24777,#24778,#24779,#24780,#24781,
#24782,#24783,#24784,#24785,#24786,#24787,#24788,#24789,#24790,#24791,#24792,
#24793,#24794,#24795,#24796,#24797,#24798,#24799,#24800,#24801,#24802,#24803,
#24804,#24805,#24806,#24807,#24808,#24809,#24810,#24811,#24812,#24813,#24814,
#24815,#24816,#24817,#24818,#24819,#24820,#24821,#24822,#24823,#24824,#24825,
#24826),.UNSPECIFIED.,.F.,.F.,(4,3,3,3,3,3,3,3,3,3,3,3,3,3,3,3,3,3,3,3,
3,3,3,3,3,3,3,3,3,3,3,4),(-0.569248610399391,-0.543573485199943,-0.517270268565312,
-0.51040343212095,-0.504800294612885,-0.477738530287438,-0.455893930851042,
-0.447075593991324,-0.442407019766337,-0.414674597913133,-0.386513035378128,
-0.358572122738531,-0.344674525752965,-0.340104447556141,-0.311173623171527,
-0.302981734796268,-0.27516514613859,-0.246719659301531,-0.236777951845204,
-0.231757521912826,-0.227579246481702,-0.198579856955019,-0.169011286171866,
-0.139212421577441,-0.12303172519304,-0.118001035990282,-0.113392013031005,
-0.0828444532672019,-0.0522704025528943,-0.0223140889578805,-0.00976685050222891,
0.),.UNSPECIFIED.);
#2644=B_SPLINE_CURVE_WITH_KNOTS('',3,(#24827,#24828,#24829,#24830,#24831,
#24832,#24833,#24834,#24835,#24836,#24837,#24838,#24839,#24840,#24841,#24842,
#24843,#24844,#24845,#24846,#24847,#24848,#24849,#24850,#24851,#24852,#24853,
#24854,#24855,#24856,#24857,#24858,#24859,#24860,#24861,#24862,#24863,#24864,
#24865,#24866,#24867,#24868,#24869,#24870,#24871,#24872,#24873,#24874,#24875,
#24876,#24877,#24878,#24879,#24880,#24881,#24882,#24883,#24884,#24885,#24886,
#24887,#24888,#24889,#24890,#24891,#24892,#24893,#24894,#24895,#24896,#24897,
#24898,#24899,#24900,#24901,#24902,#24903,#24904,#24905,#24906,#24907,#24908,
#24909,#24910,#24911,#24912,#24913,#24914,#24915,#24916,#24917,#24918,#24919,
#24920),.UNSPECIFIED.,.F.,.F.,(4,3,3,3,3,3,3,3,3,3,3,3,3,3,3,3,3,3,3,3,
3,3,3,3,3,3,3,3,3,3,3,4),(-0.566847306048135,-0.536665109075417,-0.506058896071854,
-0.497416851909175,-0.49047965571675,-0.460332721088332,-0.437086686152057,
-0.424703698099728,-0.420462735133408,-0.39103784434011,-0.361869493654616,
-0.33354585979786,-0.318750505247928,-0.313020123387797,-0.308660184852524,
-0.280670747442105,-0.274364441598135,-0.245887082189052,-0.216156157664495,
-0.204673880739737,-0.200549631762214,-0.172713963704145,-0.144949220452659,
-0.117659624553142,-0.103957132233074,-0.0999252283847502,-0.0958138212739285,
-0.0691413054179344,-0.0429166386626297,-0.0174931714382136,-0.00803968599259392,
0.),.UNSPECIFIED.);
#2645=B_SPLINE_CURVE_WITH_KNOTS('',3,(#24922,#24923,#24924,#24925,#24926,
#24927,#24928,#24929,#24930,#24931,#24932),.UNSPECIFIED.,.F.,.F.,(4,1,1,
1,1,1,1,1,4),(15.7079632679489,15.8295388729956,16.8221763756675,17.8148138783395,
18.8074513810114,19.8000888836834,20.7927263863553,21.7853638890272,21.9911485751285),
 .UNSPECIFIED.);
#2646=B_SPLINE_CURVE_WITH_KNOTS('',3,(#24933,#24934,#24935,#24936,#24937,
#24938,#24939,#24940,#24941,#24942),.UNSPECIFIED.,.F.,.F.,(4,1,1,1,1,1,
1,4),(15.7079632679489,16.3836751323157,17.3763126349877,18.3689501376596,
19.3615876403316,20.3542251430035,21.3468626456754,21.9911485751285),
 .UNSPECIFIED.);
#2647=B_SPLINE_CURVE_WITH_KNOTS('',3,(#25191,#25192,#25193,#25194,#25195,
#25196,#25197,#25198,#25199,#25200,#25201,#25202,#25203,#25204,#25205,#25206,
#25207,#25208,#25209,#25210,#25211,#25212,#25213,#25214,#25215,#25216,#25217,
#25218,#25219,#25220,#25221,#25222,#25223,#25224,#25225,#25226,#25227,#25228,
#25229,#25230,#25231,#25232,#25233,#25234,#25235,#25236,#25237,#25238,#25239,
#25240,#25241,#25242,#25243,#25244,#25245,#25246,#25247,#25248,#25249,#25250,
#25251,#25252,#25253,#25254,#25255,#25256,#25257,#25258,#25259,#25260,#25261,
#25262,#25263,#25264,#25265,#25266,#25267,#25268,#25269,#25270,#25271,#25272,
#25273,#25274,#25275,#25276,#25277,#25278,#25279,#25280,#25281),
 .UNSPECIFIED.,.F.,.F.,(4,3,3,3,3,3,3,3,3,3,3,3,3,3,3,3,3,3,3,3,3,3,3,3,
3,3,3,3,3,3,4),(0.,0.0253641940060491,0.0513998528853357,0.0781558294588739,
0.0899177835126812,0.096625586076476,0.102679521314574,0.129980972716582,
0.157733265563707,0.18466186554119,0.195928352608436,0.202971020906728,
0.20709884412475,0.236273254799196,0.265447665473641,0.293340562931045,
0.302677593280724,0.308745430621993,0.314528754610798,0.34260673975117,
0.371727130037291,0.401175578671832,0.421351088041328,0.426753710423992,
0.456805222326454,0.481883932941516,0.490048800165398,0.498378785902177,
0.528887556975208,0.557120064786702,0.566847306048017),.UNSPECIFIED.);
#2648=B_SPLINE_CURVE_WITH_KNOTS('',3,(#25282,#25283,#25284,#25285,#25286,
#25287,#25288,#25289,#25290,#25291,#25292,#25293,#25294,#25295,#25296,#25297,
#25298,#25299,#25300,#25301,#25302,#25303,#25304,#25305,#25306),
 .UNSPECIFIED.,.F.,.F.,(4,3,3,3,3,3,3,3,4),(-10.1321597128207,-9.92637502671944,
-8.9337375240475,-7.94110002137556,-6.94846251870361,-5.95582501603167,
-4.96318751335972,-3.97055001068778,-3.84897440564114),.UNSPECIFIED.);
#2649=B_SPLINE_CURVE_WITH_KNOTS('',3,(#25555,#25556,#25557,#25558,#25559,
#25560,#25561,#25562,#25563,#25564,#25565,#25566,#25567,#25568,#25569,#25570,
#25571,#25572,#25573,#25574,#25575,#25576),.UNSPECIFIED.,.F.,.F.,(4,3,3,
3,3,3,3,4),(7.59274844815667,7.94110002137556,8.9337375240475,9.92637502671945,
10.9190125293914,11.9116500320633,12.9042875347353,13.8759337553363),
 .UNSPECIFIED.);
#2650=B_SPLINE_CURVE_WITH_KNOTS('',3,(#25577,#25578,#25579,#25580,#25581,
#25582,#25583,#25584,#25585,#25586,#25587,#25588,#25589,#25590,#25591,#25592,
#25593,#25594,#25595,#25596,#25597,#25598,#25599,#25600,#25601,#25602,#25603,
#25604,#25605,#25606,#25607,#25608,#25609,#25610,#25611,#25612,#25613,#25614,
#25615,#25616,#25617,#25618,#25619,#25620,#25621,#25622,#25623,#25624,#25625,
#25626,#25627,#25628,#25629,#25630,#25631,#25632,#25633,#25634,#25635,#25636,
#25637,#25638,#25639,#25640,#25641,#25642,#25643,#25644,#25645,#25646,#25647,
#25648,#25649,#25650,#25651,#25652,#25653,#25654,#25655,#25656,#25657,#25658,
#25659,#25660,#25661,#25662,#25663,#25664,#25665,#25666,#25667),
 .UNSPECIFIED.,.F.,.F.,(4,3,3,3,3,3,3,3,3,3,3,3,3,3,3,3,3,3,3,3,3,3,3,3,
3,3,3,3,3,3,4),(0.,0.0297251106276555,0.060108839848521,0.0893486196225938,
0.114933426924907,0.120627518834092,0.150386823450882,0.179982103762232,
0.20849334733195,0.220471792278386,0.22888232925389,0.234177127568146,0.264102102804625,
0.292006786872335,0.294027078041103,0.322973449904451,0.339362616990066,
0.343535824371297,0.371629348477673,0.399767742470069,0.427502094759513,
0.437970801715733,0.445641085172893,0.450375033464681,0.478076729683868,
0.498853001848258,0.508250421438057,0.513369584444669,0.539284522924145,
0.561181818341429,0.569248610399466),.UNSPECIFIED.);
#2651=B_SPLINE_CURVE_WITH_KNOTS('',3,(#25670,#25671,#25672,#25673,#25674,
#25675,#25676,#25677,#25678,#25679,#25680,#25681,#25682,#25683,#25684,#25685,
#25686,#25687,#25688,#25689,#25690,#25691,#25692,#25693,#25694,#25695,#25696,
#25697,#25698,#25699,#25700,#25701,#25702,#25703,#25704,#25705,#25706,#25707,
#25708,#25709,#25710,#25711,#25712,#25713,#25714,#25715,#25716,#25717,#25718,
#25719,#25720,#25721,#25722,#25723,#25724,#25725,#25726,#25727,#25728,#25729,
#25730,#25731,#25732,#25733,#25734,#25735,#25736,#25737,#25738,#25739,#25740,
#25741,#25742,#25743,#25744,#25745,#25746,#25747,#25748,#25749,#25750,#25751,
#25752,#25753,#25754,#25755,#25756,#25757,#25758,#25759,#25760,#25761,#25762,
#25763),.UNSPECIFIED.,.F.,.F.,(4,3,3,3,3,3,3,3,3,3,3,3,3,3,3,3,3,3,3,3,
3,3,3,3,3,3,3,3,3,3,3,4),(-0.569248610399449,-0.543573504102472,-0.517270303312747,
-0.510403518760422,-0.504800298462602,-0.477738547398343,-0.455893945823089,
-0.447075739640472,-0.442407159267797,-0.414674752545088,-0.38651318948242,
-0.358572268495855,-0.344674635070969,-0.340104625623979,-0.311173801204194,
-0.302981734796311,-0.275165133963676,-0.246719639454603,-0.236777889761598,
-0.231757378131509,-0.227578935732346,-0.198579529322731,-0.169010949155984,
-0.139212083849189,-0.12303142968082,-0.117999764723668,-0.113391857955279,
-0.0828442953573812,-0.0522702457649171,-0.022313932701136,-0.00976685050223398,
0.),.UNSPECIFIED.);
#2652=B_SPLINE_CURVE_WITH_KNOTS('',3,(#25764,#25765,#25766,#25767,#25768,
#25769,#25770,#25771,#25772,#25773,#25774,#25775,#25776,#25777,#25778,#25779,
#25780,#25781,#25782,#25783,#25784,#25785,#25786,#25787,#25788,#25789,#25790,
#25791,#25792,#25793,#25794,#25795,#25796,#25797,#25798,#25799,#25800,#25801,
#25802,#25803,#25804,#25805,#25806,#25807,#25808,#25809,#25810,#25811,#25812,
#25813,#25814,#25815,#25816,#25817,#25818,#25819,#25820,#25821,#25822,#25823,
#25824,#25825,#25826,#25827,#25828,#25829,#25830,#25831,#25832,#25833,#25834,
#25835,#25836,#25837,#25838,#25839,#25840,#25841,#25842,#25843,#25844,#25845,
#25846,#25847,#25848,#25849,#25850,#25851,#25852,#25853,#25854,#25855,#25856,
#25857),.UNSPECIFIED.,.F.,.F.,(4,3,3,3,3,3,3,3,3,3,3,3,3,3,3,3,3,3,3,3,
3,3,3,3,3,3,3,3,3,3,3,4),(-0.566847306048014,-0.536665117697509,-0.506058906999567,
-0.497416865326767,-0.490479658240677,-0.460332723347166,-0.437086688128531,
-0.424703702775148,-0.420462740381493,-0.391037848587686,-0.361869496840286,
-0.333545860028828,-0.318750505421142,-0.31302012577693,-0.308660186240849,
-0.28067074533307,-0.274364441598086,-0.245887081933056,-0.216156157440498,
-0.204673881207202,-0.200549631596289,-0.172713964128302,-0.144949220523049,
-0.117659621509534,-0.103957129569916,-0.0999252244321675,-0.095813819666998,
-0.0691413018378718,-0.0429166306421052,-0.0174931558038003,-0.00803968599259028,
0.),.UNSPECIFIED.);
#2653=B_SPLINE_CURVE_WITH_KNOTS('',3,(#25859,#25860,#25861,#25862,#25863,
#25864,#25865,#25866,#25867,#25868,#25869),.UNSPECIFIED.,.F.,.F.,(4,1,1,
1,1,1,1,1,4),(15.7079632679489,15.8295388729956,16.8221763756675,17.8148138783395,
18.8074513810114,19.8000888836834,20.7927263863553,21.7853638890272,21.9911485751285),
 .UNSPECIFIED.);
#2654=B_SPLINE_CURVE_WITH_KNOTS('',3,(#25870,#25871,#25872,#25873,#25874,
#25875,#25876,#25877,#25878,#25879),.UNSPECIFIED.,.F.,.F.,(4,1,1,1,1,1,
1,4),(15.7079632679489,16.3836751323157,17.3763126349877,18.3689501376596,
19.3615876403316,20.3542251430035,21.3468626456755,21.9911485751285),
 .UNSPECIFIED.);
#2655=B_SPLINE_CURVE_WITH_KNOTS('',3,(#26128,#26129,#26130,#26131,#26132,
#26133,#26134,#26135,#26136,#26137,#26138,#26139,#26140,#26141,#26142,#26143,
#26144,#26145,#26146,#26147,#26148,#26149,#26150,#26151,#26152,#26153,#26154,
#26155,#26156,#26157,#26158,#26159,#26160,#26161,#26162,#26163,#26164,#26165,
#26166,#26167,#26168,#26169,#26170,#26171,#26172,#26173,#26174,#26175,#26176,
#26177,#26178,#26179,#26180,#26181,#26182,#26183,#26184,#26185,#26186,#26187,
#26188,#26189,#26190,#26191,#26192,#26193,#26194,#26195,#26196,#26197,#26198,
#26199,#26200,#26201,#26202,#26203,#26204,#26205,#26206,#26207,#26208,#26209,
#26210,#26211,#26212,#26213,#26214,#26215,#26216,#26217,#26218),
 .UNSPECIFIED.,.F.,.F.,(4,3,3,3,3,3,3,3,3,3,3,3,3,3,3,3,3,3,3,3,3,3,3,3,
3,3,3,3,3,3,4),(0.,0.0253641802043484,0.0513998265906757,0.0781558064510469,
0.0899177781668214,0.0966255853603576,0.102679521324914,0.129980963033573,
0.157733251052733,0.184661854657961,0.195928350249662,0.202971019794835,
0.207098842071563,0.236273253772604,0.265447665473645,0.293340569486741,
0.302677606942409,0.308745486155756,0.314528754108539,0.342606748516018,
0.371727143138761,0.401175592930875,0.421351120763801,0.426753697797161,
0.45680521160119,0.481883924897573,0.49004878710534,0.498378789150779,0.528887560035012,
0.557120064786721,0.566847306048034),.UNSPECIFIED.);
#2656=B_SPLINE_CURVE_WITH_KNOTS('',3,(#26219,#26220,#26221,#26222,#26223,
#26224,#26225,#26226,#26227,#26228,#26229,#26230,#26231,#26232,#26233,#26234,
#26235,#26236,#26237,#26238,#26239,#26240,#26241,#26242,#26243),
 .UNSPECIFIED.,.F.,.F.,(4,3,3,3,3,3,3,3,4),(-10.1321597128207,-9.92637502671944,
-8.9337375240475,-7.94110002137556,-6.94846251870361,-5.95582501603167,
-4.96318751335972,-3.97055001068778,-3.84897440564113),.UNSPECIFIED.);
#2657=B_SPLINE_CURVE_WITH_KNOTS('',3,(#26492,#26493,#26494,#26495,#26496,
#26497,#26498,#26499,#26500,#26501,#26502,#26503,#26504,#26505,#26506,#26507,
#26508,#26509,#26510,#26511,#26512,#26513),.UNSPECIFIED.,.F.,.F.,(4,3,3,
3,3,3,3,4),(7.59274844815666,7.94110002137556,8.9337375240475,9.92637502671945,
10.9190125293914,11.9116500320633,12.9042875347353,13.8759337553362),
 .UNSPECIFIED.);
#2658=B_SPLINE_CURVE_WITH_KNOTS('',3,(#26514,#26515,#26516,#26517,#26518,
#26519,#26520,#26521,#26522,#26523,#26524,#26525,#26526,#26527,#26528,#26529,
#26530,#26531,#26532,#26533,#26534,#26535,#26536,#26537,#26538,#26539,#26540,
#26541,#26542,#26543,#26544,#26545,#26546,#26547,#26548,#26549,#26550,#26551,
#26552,#26553,#26554,#26555,#26556,#26557,#26558,#26559,#26560,#26561,#26562,
#26563,#26564,#26565,#26566,#26567,#26568,#26569,#26570,#26571,#26572,#26573,
#26574,#26575,#26576,#26577,#26578,#26579,#26580,#26581,#26582,#26583,#26584,
#26585,#26586,#26587,#26588,#26589,#26590,#26591,#26592,#26593,#26594,#26595,
#26596,#26597,#26598,#26599,#26600,#26601,#26602,#26603,#26604),
 .UNSPECIFIED.,.F.,.F.,(4,3,3,3,3,3,3,3,3,3,3,3,3,3,3,3,3,3,3,3,3,3,3,3,
3,3,3,3,3,3,4),(0.,0.0297250940603701,0.0601088150228865,0.0893485979001609,
0.114933407917776,0.120627517502826,0.150386821838171,0.179982106532903,
0.208493349409947,0.220471797231655,0.228882342926144,0.234177131447686,
0.264102104744384,0.292006792915222,0.294027078041082,0.322973449076703,
0.339362619054412,0.34353582684914,0.371629350432206,0.399767744193081,
0.427502099759356,0.437970813749853,0.445641127145106,0.45037504344892,
0.478076737172018,0.498853007464342,0.508250442098983,0.513369590083379,
0.539284536863559,0.561181818341313,0.56924861039935),.UNSPECIFIED.);
#2659=B_SPLINE_CURVE_WITH_KNOTS('',3,(#26607,#26608,#26609,#26610,#26611,
#26612,#26613,#26614,#26615,#26616,#26617,#26618,#26619,#26620,#26621,#26622,
#26623,#26624,#26625,#26626,#26627,#26628,#26629,#26630,#26631,#26632,#26633,
#26634,#26635,#26636,#26637,#26638,#26639,#26640,#26641,#26642,#26643,#26644,
#26645,#26646,#26647,#26648,#26649,#26650,#26651,#26652,#26653,#26654,#26655,
#26656,#26657,#26658,#26659,#26660,#26661,#26662,#26663,#26664,#26665,#26666,
#26667,#26668,#26669,#26670,#26671,#26672,#26673,#26674,#26675,#26676,#26677,
#26678,#26679,#26680,#26681,#26682,#26683,#26684,#26685,#26686,#26687,#26688,
#26689,#26690,#26691,#26692,#26693,#26694,#26695,#26696,#26697,#26698,#26699,
#26700),.UNSPECIFIED.,.F.,.F.,(4,3,3,3,3,3,3,3,3,3,3,3,3,3,3,3,3,3,3,3,
3,3,3,3,3,3,3,3,3,3,3,4),(-0.569248610399476,-0.543573485205502,-0.517270268573132,
-0.510403432146651,-0.50480029464855,-0.477738530324984,-0.4558939308839,
-0.447075594297702,-0.442407020006122,-0.414674598149304,-0.386513035614215,
-0.358572122969062,-0.344674525925876,-0.340104447830039,-0.3111736234517,
-0.302981734796315,-0.275165146138309,-0.246719659299767,-0.236777951841385,
-0.231757521910833,-0.227579246473126,-0.198579856945078,-0.169011286162167,
-0.139212421569045,-0.123031725185693,-0.118001036018665,-0.113392013034907,
-0.0828444532722089,-0.0522704025570408,-0.0223140889611495,-0.0097668505022249,
0.),.UNSPECIFIED.);
#2660=B_SPLINE_CURVE_WITH_KNOTS('',3,(#26701,#26702,#26703,#26704,#26705,
#26706,#26707,#26708,#26709,#26710,#26711,#26712,#26713,#26714,#26715,#26716,
#26717,#26718,#26719,#26720,#26721,#26722,#26723,#26724,#26725,#26726,#26727,
#26728,#26729,#26730,#26731,#26732,#26733,#26734,#26735,#26736,#26737,#26738,
#26739,#26740,#26741,#26742,#26743,#26744,#26745,#26746,#26747,#26748,#26749,
#26750,#26751,#26752,#26753,#26754,#26755,#26756,#26757,#26758,#26759,#26760,
#26761,#26762,#26763,#26764,#26765,#26766,#26767,#26768,#26769,#26770,#26771,
#26772,#26773,#26774,#26775,#26776,#26777,#26778,#26779,#26780,#26781,#26782,
#26783,#26784,#26785,#26786,#26787,#26788,#26789,#26790,#26791,#26792,#26793,
#26794),.UNSPECIFIED.,.F.,.F.,(4,3,3,3,3,3,3,3,3,3,3,3,3,3,3,3,3,3,3,3,
3,3,3,3,3,3,3,3,3,3,3,4),(-0.5668473060481,-0.536665109079502,-0.506058896073369,
-0.497416851912877,-0.490479655811324,-0.460332721180406,-0.43708668623262,
-0.424703698246803,-0.420462735243598,-0.391037844452743,-0.361869493739087,
-0.333545859882985,-0.318750505311769,-0.313020123569819,-0.308660184935363,
-0.280670747518966,-0.27436444159812,-0.245887082194013,-0.216156157668836,
-0.20467388073518,-0.200549631773281,-0.172713963716999,-0.144949220465045,
-0.117659624577274,-0.103957132254189,-0.0999252285358155,-0.0958138213027416,
-0.0691413054476691,-0.04291663869175,-0.017493171464394,-0.00803968599259441,
0.),.UNSPECIFIED.);
#2661=B_SPLINE_CURVE_WITH_KNOTS('',3,(#26796,#26797,#26798,#26799,#26800,
#26801,#26802,#26803,#26804,#26805,#26806),.UNSPECIFIED.,.F.,.F.,(4,1,1,
1,1,1,1,1,4),(15.7079632679489,15.8295388729956,16.8221763756675,17.8148138783395,
18.8074513810114,19.8000888836834,20.7927263863553,21.7853638890272,21.9911485751285),
 .UNSPECIFIED.);
#2662=B_SPLINE_CURVE_WITH_KNOTS('',3,(#26807,#26808,#26809,#26810,#26811,
#26812,#26813,#26814,#26815,#26816),.UNSPECIFIED.,.F.,.F.,(4,1,1,1,1,1,
1,4),(15.7079632679489,16.3836751323157,17.3763126349877,18.3689501376596,
19.3615876403316,20.3542251430035,21.3468626456754,21.9911485751285),
 .UNSPECIFIED.);
#2663=B_SPLINE_CURVE_WITH_KNOTS('',3,(#27065,#27066,#27067,#27068,#27069,
#27070,#27071,#27072,#27073,#27074,#27075,#27076,#27077,#27078,#27079,#27080,
#27081,#27082,#27083,#27084,#27085,#27086,#27087,#27088,#27089,#27090,#27091,
#27092,#27093,#27094,#27095,#27096,#27097,#27098,#27099,#27100,#27101,#27102,
#27103,#27104,#27105,#27106,#27107,#27108,#27109,#27110,#27111,#27112,#27113,
#27114,#27115,#27116,#27117,#27118,#27119,#27120,#27121,#27122,#27123,#27124,
#27125,#27126,#27127,#27128,#27129,#27130,#27131,#27132,#27133,#27134,#27135,
#27136,#27137,#27138,#27139,#27140,#27141,#27142,#27143,#27144,#27145,#27146,
#27147,#27148,#27149,#27150,#27151,#27152,#27153,#27154,#27155),
 .UNSPECIFIED.,.F.,.F.,(4,3,3,3,3,3,3,3,3,3,3,3,3,3,3,3,3,3,3,3,3,3,3,3,
3,3,3,3,3,3,4),(0.,0.0253641940059154,0.0513998528845501,0.0781558294581879,
0.0899177835124791,0.0966255860763879,0.102679521323728,0.129980972726384,
0.157733265573268,0.184661865548364,0.195928352610419,0.202971020904623,
0.207098844127634,0.236273254800643,0.265447665473653,0.293340562930928,
0.302677593280407,0.30874543062048,0.314528754623958,0.342606739764072,
0.371727130050435,0.401175578685423,0.421351088070314,0.426753710426087,
0.45680522232921,0.4818839329436,0.490048800169418,0.498378785911953,0.52888755698416,
0.557120064786771,0.566847306048087),.UNSPECIFIED.);
#2664=B_SPLINE_CURVE_WITH_KNOTS('',3,(#27156,#27157,#27158,#27159,#27160,
#27161,#27162,#27163,#27164,#27165,#27166,#27167,#27168,#27169,#27170,#27171,
#27172,#27173,#27174,#27175,#27176,#27177,#27178,#27179,#27180),
 .UNSPECIFIED.,.F.,.F.,(4,3,3,3,3,3,3,3,4),(-10.1321597128207,-9.92637502671944,
-8.9337375240475,-7.94110002137556,-6.94846251870361,-5.95582501603167,
-4.96318751335973,-3.97055001068778,-3.84897440564114),.UNSPECIFIED.);
#2665=B_SPLINE_CURVE_WITH_KNOTS('',3,(#27429,#27430,#27431,#27432,#27433,
#27434,#27435,#27436,#27437,#27438,#27439,#27440,#27441,#27442,#27443,#27444,
#27445,#27446,#27447,#27448,#27449,#27450),.UNSPECIFIED.,.F.,.F.,(4,3,3,
3,3,3,3,4),(7.59274844815666,7.94110002137556,8.9337375240475,9.92637502671945,
10.9190125293914,11.9116500320633,12.9042875347353,13.8759337553362),
 .UNSPECIFIED.);
#2666=B_SPLINE_CURVE_WITH_KNOTS('',3,(#27451,#27452,#27453,#27454,#27455,
#27456,#27457,#27458,#27459,#27460,#27461,#27462,#27463,#27464,#27465,#27466,
#27467,#27468,#27469,#27470,#27471,#27472,#27473,#27474,#27475,#27476,#27477,
#27478,#27479,#27480,#27481,#27482,#27483,#27484,#27485,#27486,#27487,#27488,
#27489,#27490,#27491,#27492,#27493,#27494,#27495,#27496,#27497,#27498,#27499,
#27500,#27501,#27502,#27503,#27504,#27505,#27506,#27507,#27508,#27509,#27510,
#27511,#27512,#27513,#27514,#27515,#27516,#27517,#27518,#27519,#27520,#27521,
#27522,#27523,#27524,#27525,#27526,#27527,#27528,#27529,#27530,#27531,#27532,
#27533,#27534,#27535,#27536,#27537,#27538,#27539,#27540,#27541),
 .UNSPECIFIED.,.F.,.F.,(4,3,3,3,3,3,3,3,3,3,3,3,3,3,3,3,3,3,3,3,3,3,3,3,
3,3,3,3,3,3,4),(0.,0.0297251106280497,0.0601088398490155,0.0893486196230253,
0.114933426925284,0.120627518834333,0.150386823451848,0.179982103763167,
0.208493347332649,0.220471792279509,0.228882329257328,0.234177127564844,
0.264102102802969,0.292006786870997,0.294027078041094,0.322973449904779,
0.339362616990787,0.343535824361368,0.371629348467577,0.399767742460233,
0.427502094749591,0.437970801695254,0.445641085107272,0.45037503345148,
0.47807672967396,0.498853001840821,0.508250421414146,0.513369584440127,
0.539284522919995,0.561181818341402,0.569248610399439),.UNSPECIFIED.);
#2667=B_SPLINE_CURVE_WITH_KNOTS('',3,(#27544,#27545,#27546,#27547,#27548,
#27549,#27550,#27551,#27552,#27553,#27554,#27555,#27556,#27557,#27558,#27559,
#27560,#27561,#27562,#27563,#27564,#27565,#27566,#27567,#27568,#27569,#27570,
#27571,#27572,#27573,#27574,#27575,#27576,#27577,#27578,#27579,#27580,#27581,
#27582,#27583,#27584,#27585,#27586,#27587,#27588,#27589,#27590,#27591,#27592,
#27593,#27594,#27595,#27596,#27597,#27598,#27599,#27600,#27601,#27602,#27603,
#27604,#27605,#27606,#27607,#27608,#27609,#27610,#27611,#27612,#27613,#27614,
#27615,#27616,#27617,#27618,#27619,#27620,#27621,#27622,#27623,#27624,#27625,
#27626,#27627,#27628,#27629,#27630,#27631,#27632,#27633,#27634,#27635,#27636,
#27637),.UNSPECIFIED.,.F.,.F.,(4,3,3,3,3,3,3,3,3,3,3,3,3,3,3,3,3,3,3,3,
3,3,3,3,3,3,3,3,3,3,3,4),(-0.569248610399503,-0.543573536725572,-0.517270363300643,
-0.510403668322967,-0.504800305048166,-0.47773857688201,-0.455893971621299,
-0.447075990604545,-0.442407399438625,-0.414675018820766,-0.386513454853249,
-0.35857251946668,-0.34467482329909,-0.340104931946522,-0.311174107463772,
-0.302981734796321,-0.275165112945586,-0.246719605186861,-0.236777782574912,
-0.231757129804548,-0.227578398489937,-0.198578962914807,-0.169010366535306,
-0.139211499993959,-0.123030918807493,-0.117997565283917,-0.113391588480745,
-0.0828440209838422,-0.0522699733385328,-0.0223136612161147,-0.00976685050222925,
0.),.UNSPECIFIED.);
#2668=B_SPLINE_CURVE_WITH_KNOTS('',3,(#27638,#27639,#27640,#27641,#27642,
#27643,#27644,#27645,#27646,#27647,#27648,#27649,#27650,#27651,#27652,#27653,
#27654,#27655,#27656,#27657,#27658,#27659,#27660,#27661,#27662,#27663,#27664,
#27665,#27666,#27667,#27668,#27669,#27670,#27671,#27672,#27673,#27674,#27675,
#27676,#27677,#27678,#27679,#27680,#27681,#27682,#27683,#27684,#27685,#27686,
#27687,#27688,#27689,#27690,#27691,#27692,#27693,#27694,#27695,#27696,#27697,
#27698,#27699,#27700,#27701,#27702,#27703,#27704,#27705,#27706,#27707,#27708,
#27709,#27710,#27711,#27712,#27713,#27714,#27715,#27716,#27717,#27718,#27719,
#27720,#27721,#27722,#27723,#27724,#27725,#27726,#27727,#27728,#27729,#27730,
#27731),.UNSPECIFIED.,.F.,.F.,(4,3,3,3,3,3,3,3,3,3,3,3,3,3,3,3,3,3,3,3,
3,3,3,3,3,3,3,3,3,3,3,4),(-0.566847306048007,-0.536665099326187,-0.50605888371953,
-0.497416836745447,-0.490479652851239,-0.460332718522974,-0.437086683907363,
-0.424703692798494,-0.420462729215447,-0.391037839556167,-0.361869490066648,
-0.333545859553922,-0.318750505064964,-0.31302012072499,-0.308660183331501,
-0.280670749875022,-0.27436444159809,-0.245887082485289,-0.216156157923702,
-0.204673880207543,-0.200549631930185,-0.172713963206743,-0.144949220356295,
-0.117659627980649,-0.103957135232142,-0.099925232967256,-0.0958138231131305,
-0.069141309492666,-0.042916647764108,-0.017493189155658,-0.00803968599259752,
0.),.UNSPECIFIED.);
#2669=B_SPLINE_CURVE_WITH_KNOTS('',3,(#27733,#27734,#27735,#27736,#27737,
#27738,#27739,#27740,#27741,#27742,#27743),.UNSPECIFIED.,.F.,.F.,(4,1,1,
1,1,1,1,1,4),(15.7079632679489,15.8295388729956,16.8221763756675,17.8148138783395,
18.8074513810114,19.8000888836834,20.7927263863553,21.7853638890272,21.9911485751285),
 .UNSPECIFIED.);
#2670=B_SPLINE_CURVE_WITH_KNOTS('',3,(#27744,#27745,#27746,#27747,#27748,
#27749,#27750,#27751,#27752,#27753),.UNSPECIFIED.,.F.,.F.,(4,1,1,1,1,1,
1,4),(15.7079632679489,16.3836751323157,17.3763126349877,18.3689501376596,
19.3615876403316,20.3542251430035,21.3468626456754,21.9911485751285),
 .UNSPECIFIED.);
#2671=B_SPLINE_CURVE_WITH_KNOTS('',3,(#28002,#28003,#28004,#28005,#28006,
#28007,#28008,#28009,#28010,#28011,#28012,#28013,#28014,#28015,#28016,#28017,
#28018,#28019,#28020,#28021,#28022,#28023,#28024,#28025,#28026,#28027,#28028,
#28029,#28030,#28031,#28032,#28033,#28034,#28035,#28036,#28037,#28038,#28039,
#28040,#28041,#28042,#28043,#28044,#28045,#28046,#28047,#28048,#28049,#28050,
#28051,#28052,#28053,#28054,#28055,#28056,#28057,#28058,#28059,#28060,#28061,
#28062,#28063,#28064,#28065,#28066,#28067,#28068,#28069,#28070,#28071,#28072,
#28073,#28074,#28075,#28076,#28077,#28078,#28079,#28080,#28081,#28082,#28083,
#28084,#28085,#28086,#28087,#28088,#28089,#28090,#28091,#28092),
 .UNSPECIFIED.,.F.,.F.,(4,3,3,3,3,3,3,3,3,3,3,3,3,3,3,3,3,3,3,3,3,3,3,3,
3,3,3,3,3,3,4),(0.,0.0253642096190117,0.0513998826294253,0.078155855484953,
0.0899177895597073,0.0966255868864595,0.102679521322493,0.129980983690104,
0.157733281997098,0.184661877866235,0.195928355280655,0.20297102215946,
0.207098846520249,0.236273255996948,0.265447665473647,0.293340555515042,
0.302677577825464,0.308745367797819,0.314528755194195,0.342606729849992,
0.37172711523001,0.401175562555647,0.421351051054358,0.426753724713226,
0.45680523446668,0.481883942046697,0.490048814948903,0.498378782214203,
0.528887553499741,0.557120064786748,0.566847306048067),.UNSPECIFIED.);
#2672=B_SPLINE_CURVE_WITH_KNOTS('',3,(#28093,#28094,#28095,#28096,#28097,
#28098,#28099,#28100,#28101,#28102,#28103,#28104,#28105,#28106,#28107,#28108,
#28109,#28110,#28111,#28112,#28113,#28114,#28115,#28116,#28117),
 .UNSPECIFIED.,.F.,.F.,(4,3,3,3,3,3,3,3,4),(-10.1321597128207,-9.92637502671945,
-8.93373752404751,-7.94110002137556,-6.94846251870361,-5.95582501603167,
-4.96318751335972,-3.97055001068778,-3.84897440564114),.UNSPECIFIED.);
#2673=B_SPLINE_CURVE_WITH_KNOTS('',3,(#28366,#28367,#28368,#28369,#28370,
#28371,#28372,#28373,#28374,#28375,#28376,#28377,#28378,#28379,#28380,#28381,
#28382,#28383,#28384,#28385,#28386,#28387),.UNSPECIFIED.,.F.,.F.,(4,3,3,
3,3,3,3,4),(7.59274844815666,7.94110002137556,8.93373752404751,9.92637502671945,
10.9190125293914,11.9116500320633,12.9042875347353,13.8759337553362),
 .UNSPECIFIED.);
#2674=B_SPLINE_CURVE_WITH_KNOTS('',3,(#28388,#28389,#28390,#28391,#28392,
#28393,#28394,#28395,#28396,#28397,#28398,#28399,#28400,#28401,#28402,#28403,
#28404,#28405,#28406,#28407,#28408,#28409,#28410,#28411,#28412,#28413,#28414,
#28415,#28416,#28417,#28418,#28419,#28420,#28421,#28422,#28423,#28424,#28425,
#28426,#28427,#28428,#28429,#28430,#28431,#28432,#28433,#28434,#28435,#28436,
#28437,#28438,#28439,#28440,#28441,#28442,#28443,#28444,#28445,#28446,#28447,
#28448,#28449,#28450,#28451,#28452,#28453,#28454,#28455,#28456,#28457,#28458,
#28459,#28460,#28461,#28462,#28463,#28464,#28465,#28466,#28467,#28468,#28469,
#28470,#28471,#28472,#28473,#28474,#28475,#28476,#28477,#28478),
 .UNSPECIFIED.,.F.,.F.,(4,3,3,3,3,3,3,3,3,3,3,3,3,3,3,3,3,3,3,3,3,3,3,3,
3,3,3,3,3,3,4),(0.,0.029725065450369,0.060108772149361,0.0893485603858319,
0.114933375092744,0.120627515201239,0.150386819046978,0.179982111308832,
0.208493352991906,0.220471805772867,0.228882366497282,0.234177138099837,
0.264102108070482,0.292006803324548,0.294027078041128,0.322973447643439,
0.339362622606945,0.343535831117231,0.371629353795543,0.399767747153013,
0.427502108367365,0.437970834477791,0.445641199459811,0.450375060656323,
0.478076750077611,0.498853017143577,0.50825047771638,0.513369599808131,
0.539284560911353,0.561181818341475,0.569248610399517),.UNSPECIFIED.);
#2675=B_SPLINE_CURVE_WITH_KNOTS('',3,(#28481,#28482,#28483,#28484,#28485,
#28486,#28487,#28488,#28489,#28490,#28491,#28492,#28493,#28494,#28495,#28496,
#28497,#28498,#28499,#28500,#28501,#28502,#28503,#28504,#28505,#28506,#28507,
#28508,#28509,#28510,#28511,#28512,#28513,#28514,#28515,#28516,#28517,#28518,
#28519,#28520,#28521,#28522,#28523,#28524,#28525,#28526,#28527,#28528,#28529,
#28530,#28531,#28532,#28533,#28534,#28535,#28536,#28537,#28538,#28539,#28540,
#28541,#28542,#28543,#28544,#28545,#28546,#28547,#28548,#28549,#28550,#28551,
#28552,#28553,#28554,#28555,#28556,#28557,#28558,#28559,#28560,#28561,#28562,
#28563,#28564,#28565,#28566,#28567,#28568,#28569,#28570,#28571,#28572,#28573,
#28574),.UNSPECIFIED.,.F.,.F.,(4,3,3,3,3,3,3,3,3,3,3,3,3,3,3,3,3,3,3,3,
3,3,3,3,3,3,3,3,3,3,3,4),(-0.569248610399503,-0.543573521277575,-0.51727033489437,
-0.510403597501007,-0.504800301984927,-0.477738562977673,-0.455893959455004,
-0.447075872238583,-0.442407286260358,-0.414674893289812,-0.386513329748341,
-0.358572401173164,-0.344674734578953,-0.340104787662881,-0.311173963212057,
-0.302981734796321,-0.275165122896258,-0.246719621408367,-0.236777833316757,
-0.231757247392069,-0.22757865289815,-0.198579231130546,-0.169010642427486,
-0.139211776471259,-0.12303116072513,-0.117998607181915,-0.113391716319945,
-0.0828441511418465,-0.0522701025755355,-0.0223137900019766,-0.00976685050222925,
0.),.UNSPECIFIED.);
#2676=B_SPLINE_CURVE_WITH_KNOTS('',3,(#28575,#28576,#28577,#28578,#28579,
#28580,#28581,#28582,#28583,#28584,#28585,#28586,#28587,#28588,#28589,#28590,
#28591,#28592,#28593,#28594,#28595,#28596,#28597,#28598,#28599,#28600,#28601,
#28602,#28603,#28604,#28605,#28606,#28607,#28608,#28609,#28610,#28611,#28612,
#28613,#28614,#28615,#28616,#28617,#28618,#28619,#28620,#28621,#28622,#28623,
#28624,#28625,#28626,#28627,#28628,#28629,#28630,#28631,#28632,#28633,#28634,
#28635,#28636,#28637,#28638,#28639,#28640,#28641,#28642,#28643,#28644,#28645,
#28646,#28647,#28648,#28649,#28650,#28651,#28652,#28653,#28654,#28655,#28656,
#28657,#28658,#28659,#28660,#28661,#28662,#28663,#28664,#28665,#28666,#28667,
#28668),.UNSPECIFIED.,.F.,.F.,(4,3,3,3,3,3,3,3,3,3,3,3,3,3,3,3,3,3,3,3,
3,3,3,3,3,3,3,3,3,3,3,4),(-0.566847306048007,-0.536665088443819,-0.506058869926945,
-0.497416819812331,-0.490479649708581,-0.4603327157151,-0.437086681450474,
-0.424703686967728,-0.420462722527238,-0.391037834128131,-0.36186948599562,
-0.333545859211528,-0.318750504808168,-0.313020117605598,-0.308660181455267,
-0.280670752414333,-0.27436444159809,-0.24588708281337,-0.216156158210774,
-0.204673879612822,-0.200549632067082,-0.172713962600946,-0.144949220202067,
-0.117659631764077,-0.103957138542642,-0.0999252379790372,-0.0958138251467766,
-0.0691413140230926,-0.0429166579078794,-0.0174932089177672,-0.00803968599259752,
0.),.UNSPECIFIED.);
#2677=B_SPLINE_CURVE_WITH_KNOTS('',3,(#28670,#28671,#28672,#28673,#28674,
#28675,#28676,#28677,#28678,#28679,#28680),.UNSPECIFIED.,.F.,.F.,(4,1,1,
1,1,1,1,1,4),(15.7079632679489,15.8295388729956,16.8221763756675,17.8148138783395,
18.8074513810114,19.8000888836834,20.7927263863553,21.7853638890272,21.9911485751285),
 .UNSPECIFIED.);
#2678=B_SPLINE_CURVE_WITH_KNOTS('',3,(#28681,#28682,#28683,#28684,#28685,
#28686,#28687,#28688,#28689,#28690),.UNSPECIFIED.,.F.,.F.,(4,1,1,1,1,1,
1,4),(15.7079632679489,16.3836751323157,17.3763126349877,18.3689501376596,
19.3615876403316,20.3542251430035,21.3468626456754,21.9911485751285),
 .UNSPECIFIED.);
#2679=B_SPLINE_CURVE_WITH_KNOTS('',3,(#28939,#28940,#28941,#28942,#28943,
#28944,#28945,#28946,#28947,#28948,#28949,#28950,#28951,#28952,#28953,#28954,
#28955,#28956,#28957,#28958,#28959,#28960,#28961,#28962,#28963,#28964,#28965,
#28966,#28967,#28968,#28969,#28970,#28971,#28972,#28973,#28974,#28975,#28976,
#28977,#28978,#28979,#28980,#28981,#28982,#28983,#28984,#28985,#28986,#28987,
#28988,#28989,#28990,#28991,#28992,#28993,#28994,#28995,#28996,#28997,#28998,
#28999,#29000,#29001,#29002,#29003,#29004,#29005,#29006,#29007,#29008,#29009,
#29010,#29011,#29012,#29013,#29014,#29015,#29016,#29017,#29018,#29019,#29020,
#29021,#29022,#29023,#29024,#29025,#29026,#29027,#29028,#29029),
 .UNSPECIFIED.,.F.,.F.,(4,3,3,3,3,3,3,3,3,3,3,3,3,3,3,3,3,3,3,3,3,3,3,3,
3,3,3,3,3,3,4),(0.,0.0253642270426691,0.0513999158235613,0.0781558845298221,
0.0899177963077374,0.0966255877901253,0.102679521320011,0.12998099592429,
0.157733300324819,0.184661891612026,0.195928358260196,0.202971023559155,
0.207098849097602,0.236273257285624,0.265447665473647,0.293340547237358,
0.302677560574417,0.30874529767522,0.314528755850086,0.342606718802077,
0.371727098706227,0.401175544570548,0.421351009778467,0.426753740647144,
0.456805248003638,0.481883952199416,0.490048831431489,0.498378778130755,
0.528887549653182,0.557120064786748,0.566847306048067),.UNSPECIFIED.);
#2680=B_SPLINE_CURVE_WITH_KNOTS('',3,(#29030,#29031,#29032,#29033,#29034,
#29035,#29036,#29037,#29038,#29039,#29040,#29041,#29042,#29043,#29044,#29045,
#29046,#29047,#29048,#29049,#29050,#29051,#29052,#29053,#29054),
 .UNSPECIFIED.,.F.,.F.,(4,3,3,3,3,3,3,3,4),(-10.1321597128207,-9.92637502671945,
-8.93373752404751,-7.94110002137556,-6.94846251870361,-5.95582501603167,
-4.96318751335972,-3.97055001068778,-3.84897440564114),.UNSPECIFIED.);
#2681=B_SPLINE_CURVE_WITH_KNOTS('',3,(#29303,#29304,#29305,#29306,#29307,
#29308,#29309,#29310,#29311,#29312,#29313,#29314,#29315,#29316,#29317,#29318,
#29319,#29320,#29321,#29322,#29323,#29324),.UNSPECIFIED.,.F.,.F.,(4,3,3,
3,3,3,3,4),(7.59274844815666,7.94110002137556,8.93373752404751,9.92637502671945,
10.9190125293914,11.9116500320633,12.9042875347353,13.8759337553362),
 .UNSPECIFIED.);
#2682=B_SPLINE_CURVE_WITH_KNOTS('',3,(#29325,#29326,#29327,#29328,#29329,
#29330,#29331,#29332,#29333,#29334,#29335,#29336,#29337,#29338,#29339,#29340,
#29341,#29342,#29343,#29344,#29345,#29346,#29347,#29348,#29349,#29350,#29351,
#29352,#29353,#29354,#29355,#29356,#29357,#29358,#29359,#29360,#29361,#29362,
#29363,#29364,#29365,#29366,#29367,#29368,#29369,#29370,#29371,#29372,#29373,
#29374,#29375,#29376,#29377,#29378,#29379,#29380,#29381,#29382,#29383,#29384,
#29385,#29386,#29387,#29388,#29389,#29390,#29391,#29392,#29393,#29394,#29395,
#29396,#29397,#29398,#29399,#29400,#29401,#29402,#29403,#29404,#29405,#29406,
#29407,#29408,#29409,#29410,#29411,#29412,#29413,#29414,#29415),
 .UNSPECIFIED.,.F.,.F.,(4,3,3,3,3,3,3,3,3,3,3,3,3,3,3,3,3,3,3,3,3,3,3,3,
3,3,3,3,3,3,4),(0.,0.0297250789967798,0.0601087924493119,0.0893485781482889,
0.114933390634894,0.120627516294312,0.150386820372194,0.179982109051852,
0.208493351299171,0.220471801734144,0.228882355353164,0.234177134961176,
0.264102106501152,0.292006798402076,0.294027078041128,0.32297344832203,
0.339362620925334,0.343535829103202,0.371629352210162,0.399767745759375,
0.427502104300572,0.437970824682022,0.445641165284965,0.450375052521985,
0.478076743976858,0.498853012568012,0.508250460876233,0.513369595208601,
0.539284549532082,0.561181818341475,0.569248610399517),.UNSPECIFIED.);
#2683=B_SPLINE_CURVE_WITH_KNOTS('',3,(#29418,#29419,#29420,#29421,#29422,
#29423,#29424,#29425,#29426,#29427,#29428,#29429,#29430,#29431,#29432,#29433,
#29434,#29435,#29436,#29437,#29438,#29439,#29440,#29441,#29442,#29443,#29444,
#29445,#29446,#29447,#29448,#29449,#29450,#29451,#29452,#29453,#29454,#29455,
#29456,#29457,#29458,#29459,#29460,#29461,#29462,#29463,#29464,#29465,#29466,
#29467,#29468,#29469,#29470,#29471,#29472,#29473,#29474,#29475,#29476,#29477,
#29478,#29479,#29480,#29481,#29482,#29483,#29484,#29485,#29486,#29487,#29488,
#29489,#29490,#29491,#29492,#29493,#29494,#29495,#29496,#29497,#29498,#29499,
#29500,#29501,#29502,#29503,#29504,#29505,#29506,#29507,#29508,#29509,#29510,
#29511),.UNSPECIFIED.,.F.,.F.,(4,3,3,3,3,3,3,3,3,3,3,3,3,3,3,3,3,3,3,3,
3,3,3,3,3,3,3,3,3,3,3,4),(-0.569248610399476,-0.543573504098887,-0.517270303307527,
-0.510403518746194,-0.504800298512377,-0.477738547447543,-0.45589394586614,
-0.447075740045164,-0.442407159583378,-0.414674752859423,-0.386513189796536,
-0.358572268806566,-0.344674635304004,-0.340104625965199,-0.3111738015465,
-0.302981734796315,-0.275165133962666,-0.246719639451408,-0.236777889756063,
-0.23175737813359,-0.227578935587986,-0.19857952917295,-0.16901094900184,
-0.139212083695293,-0.12303142954616,-0.117999764265674,-0.113391857900451,
-0.0828442953049202,-0.0522702457140997,-0.0223139326486197,-0.0097668505022249,
0.),.UNSPECIFIED.);
#2684=B_SPLINE_CURVE_WITH_KNOTS('',3,(#29512,#29513,#29514,#29515,#29516,
#29517,#29518,#29519,#29520,#29521,#29522,#29523,#29524,#29525,#29526,#29527,
#29528,#29529,#29530,#29531,#29532,#29533,#29534,#29535,#29536,#29537,#29538,
#29539,#29540,#29541,#29542,#29543,#29544,#29545,#29546,#29547,#29548,#29549,
#29550,#29551,#29552,#29553,#29554,#29555,#29556,#29557,#29558,#29559,#29560,
#29561,#29562,#29563,#29564,#29565,#29566,#29567,#29568,#29569,#29570,#29571,
#29572,#29573,#29574,#29575,#29576,#29577,#29578,#29579,#29580,#29581,#29582,
#29583,#29584,#29585,#29586,#29587,#29588,#29589,#29590,#29591,#29592,#29593,
#29594,#29595,#29596,#29597,#29598,#29599,#29600,#29601,#29602,#29603,#29604,
#29605),.UNSPECIFIED.,.F.,.F.,(4,3,3,3,3,3,3,3,3,3,3,3,3,3,3,3,3,3,3,3,
3,3,3,3,3,3,3,3,3,3,3,4),(-0.5668473060481,-0.536665117700605,-0.506058907018577,
-0.497416865349869,-0.490479658256923,-0.460332723361999,-0.437086688141514,
-0.424703702797736,-0.420462740364944,-0.391037848573074,-0.361869496829336,
-0.333545860020099,-0.318750505414604,-0.313020125757269,-0.308660186231234,
-0.280670745320505,-0.27436444159812,-0.245887081934671,-0.216156157441912,
-0.204673881207046,-0.200549631648242,-0.172713964179309,-0.1449492205742,
-0.117659621562307,-0.103957129616093,-0.099925224573015,-0.0958138196940146,
-0.0691413018599106,-0.0429166306649946,-0.017493155823278,-0.00803968599259441,
0.),.UNSPECIFIED.);
#2685=B_SPLINE_CURVE_WITH_KNOTS('',3,(#29607,#29608,#29609,#29610,#29611,
#29612,#29613,#29614,#29615,#29616,#29617),.UNSPECIFIED.,.F.,.F.,(4,1,1,
1,1,1,1,1,4),(15.7079632679489,15.8295388729956,16.8221763756675,17.8148138783395,
18.8074513810114,19.8000888836834,20.7927263863553,21.7853638890272,21.9911485751285),
 .UNSPECIFIED.);
#2686=B_SPLINE_CURVE_WITH_KNOTS('',3,(#29618,#29619,#29620,#29621,#29622,
#29623,#29624,#29625,#29626,#29627),.UNSPECIFIED.,.F.,.F.,(4,1,1,1,1,1,
1,4),(15.7079632679489,16.3836751323157,17.3763126349877,18.3689501376596,
19.3615876403316,20.3542251430035,21.3468626456754,21.9911485751285),
 .UNSPECIFIED.);
#2687=B_SPLINE_CURVE_WITH_KNOTS('',3,(#29876,#29877,#29878,#29879,#29880,
#29881,#29882,#29883,#29884,#29885,#29886,#29887,#29888,#29889,#29890,#29891,
#29892,#29893,#29894,#29895,#29896,#29897,#29898,#29899,#29900,#29901,#29902,
#29903,#29904,#29905,#29906,#29907,#29908,#29909,#29910,#29911,#29912,#29913,
#29914,#29915,#29916,#29917,#29918,#29919,#29920,#29921,#29922,#29923,#29924,
#29925,#29926,#29927,#29928,#29929,#29930,#29931,#29932,#29933,#29934,#29935,
#29936,#29937,#29938,#29939,#29940,#29941,#29942,#29943,#29944,#29945,#29946,
#29947,#29948,#29949,#29950,#29951,#29952,#29953,#29954,#29955,#29956,#29957,
#29958,#29959,#29960,#29961,#29962,#29963,#29964,#29965,#29966),
 .UNSPECIFIED.,.F.,.F.,(4,3,3,3,3,3,3,3,3,3,3,3,3,3,3,3,3,3,3,3,3,3,3,3,
3,3,3,3,3,3,4),(0.,0.0253641802036794,0.0513998265899383,0.0781558064504026,
0.0899177781666192,0.0966255853603217,0.102679521312511,0.129980963020898,
0.157733251039943,0.18466185464837,0.195928350246773,0.202971019797871,
0.207098842066092,0.236273253769872,0.265447665473653,0.293340569485815,
0.302677606940801,0.308745486149141,0.314528754111136,0.342606748517284,
0.371727143140112,0.401175592932008,0.421351120766356,0.426753697775984,
0.456805211578956,0.48188392488091,0.490048787075816,0.498378789152568,
0.528887560036472,0.557120064786771,0.566847306048087),.UNSPECIFIED.);
#2688=B_SPLINE_CURVE_WITH_KNOTS('',3,(#29967,#29968,#29969,#29970,#29971,
#29972,#29973,#29974,#29975,#29976,#29977,#29978,#29979,#29980,#29981,#29982,
#29983,#29984,#29985,#29986,#29987,#29988,#29989,#29990,#29991),
 .UNSPECIFIED.,.F.,.F.,(4,3,3,3,3,3,3,3,4),(-10.1321597128207,-9.92637502671944,
-8.9337375240475,-7.94110002137556,-6.94846251870361,-5.95582501603167,
-4.96318751335973,-3.97055001068778,-3.84897440564114),.UNSPECIFIED.);
#2689=B_SPLINE_CURVE_WITH_KNOTS('',3,(#30240,#30241,#30242,#30243,#30244,
#30245,#30246,#30247,#30248,#30249,#30250,#30251,#30252,#30253,#30254,#30255,
#30256,#30257,#30258,#30259,#30260,#30261),.UNSPECIFIED.,.F.,.F.,(4,3,3,
3,3,3,3,4),(7.59274844815666,7.94110002137556,8.9337375240475,9.92637502671945,
10.9190125293914,11.9116500320633,12.9042875347353,13.8759337553362),
 .UNSPECIFIED.);
#2690=B_SPLINE_CURVE_WITH_KNOTS('',3,(#30262,#30263,#30264,#30265,#30266,
#30267,#30268,#30269,#30270,#30271,#30272,#30273,#30274,#30275,#30276,#30277,
#30278,#30279,#30280,#30281,#30282,#30283,#30284,#30285,#30286,#30287,#30288,
#30289,#30290,#30291,#30292,#30293,#30294,#30295,#30296,#30297,#30298,#30299,
#30300,#30301,#30302,#30303,#30304,#30305,#30306,#30307,#30308,#30309,#30310,
#30311,#30312,#30313,#30314,#30315,#30316,#30317,#30318,#30319,#30320,#30321,
#30322,#30323,#30324,#30325,#30326,#30327,#30328,#30329,#30330,#30331,#30332,
#30333,#30334,#30335,#30336,#30337,#30338,#30339,#30340,#30341,#30342,#30343,
#30344,#30345,#30346,#30347,#30348,#30349,#30350,#30351,#30352),
 .UNSPECIFIED.,.F.,.F.,(4,3,3,3,3,3,3,3,3,3,3,3,3,3,3,3,3,3,3,3,3,3,3,3,
3,3,3,3,3,3,4),(0.,0.0297250940606226,0.0601088150228004,0.0893485979000871,
0.114933407917713,0.120627517505873,0.150386821840842,0.179982106535776,
0.208493349412105,0.220471797235071,0.228882342936493,0.234177131450068,
0.264102104745581,0.292006792916583,0.294027078041094,0.322973449076029,
0.339362619052793,0.343535826866069,0.371629350449308,0.399767744210079,
0.42750209977512,0.437970813781883,0.445641127259269,0.450375043472223,
0.478076737189517,0.498853007477489,0.508250442141124,0.513369590092699,
0.539284536873453,0.561181818341402,0.569248610399439),.UNSPECIFIED.);
#2691=B_SPLINE_CURVE_WITH_KNOTS('',3,(#30355,#30356,#30357,#30358,#30359,
#30360,#30361,#30362,#30363,#30364,#30365,#30366,#30367,#30368,#30369,#30370,
#30371,#30372,#30373,#30374,#30375,#30376,#30377,#30378,#30379,#30380,#30381,
#30382,#30383,#30384,#30385,#30386,#30387,#30388,#30389,#30390,#30391,#30392,
#30393,#30394,#30395,#30396,#30397,#30398,#30399,#30400,#30401,#30402,#30403,
#30404,#30405,#30406,#30407,#30408,#30409,#30410,#30411,#30412,#30413,#30414,
#30415,#30416,#30417,#30418,#30419,#30420,#30421,#30422,#30423,#30424,#30425,
#30426,#30427,#30428,#30429,#30430,#30431,#30432,#30433,#30434,#30435,#30436,
#30437,#30438,#30439,#30440,#30441,#30442,#30443,#30444,#30445,#30446,#30447,
#30448),.UNSPECIFIED.,.F.,.F.,(4,3,3,3,3,3,3,3,3,3,3,3,3,3,3,3,3,3,3,3,
3,3,3,3,3,3,3,3,3,3,3,4),(-0.569248610399398,-0.543573536722457,-0.517270363294533,
-0.51040366831408,-0.504800304920549,-0.477738576752391,-0.455893971507876,
-0.447075989543432,-0.442407398493899,-0.414675017857191,-0.386513453890818,
-0.358572518516808,-0.344674822586674,-0.340104930814443,-0.311174106326863,
-0.30298173479627,-0.275165112946267,-0.246719605185614,-0.236777782571111,
-0.231757129783002,-0.227578398430794,-0.19857896285462,-0.169010366474117,
-0.13921149993454,-0.1230309187555,-0.11799756500965,-0.1133915884468,-0.0828440209407878,
-0.0522699732955569,-0.0223136611739256,-0.009766850502225,0.),
 .UNSPECIFIED.);
#2692=B_SPLINE_CURVE_WITH_KNOTS('',3,(#30449,#30450,#30451,#30452,#30453,
#30454,#30455,#30456,#30457,#30458,#30459,#30460,#30461,#30462,#30463,#30464,
#30465,#30466,#30467,#30468,#30469,#30470,#30471,#30472,#30473,#30474,#30475,
#30476,#30477,#30478,#30479,#30480,#30481,#30482,#30483,#30484,#30485,#30486,
#30487,#30488,#30489,#30490,#30491,#30492,#30493,#30494,#30495,#30496,#30497,
#30498,#30499,#30500,#30501,#30502,#30503,#30504,#30505,#30506,#30507,#30508,
#30509,#30510,#30511,#30512,#30513,#30514,#30515,#30516,#30517,#30518,#30519,
#30520,#30521,#30522,#30523,#30524,#30525,#30526,#30527,#30528,#30529,#30530,
#30531,#30532,#30533,#30534,#30535,#30536,#30537,#30538,#30539,#30540,#30541,
#30542),.UNSPECIFIED.,.F.,.F.,(4,3,3,3,3,3,3,3,3,3,3,3,3,3,3,3,3,3,3,3,
3,3,3,3,3,3,3,3,3,3,3,4),(-0.566847306048064,-0.53666509932804,-0.506058883722337,
-0.49741683674965,-0.490479652915231,-0.460332718584937,-0.437086683961585,
-0.424703692897771,-0.420462729229891,-0.391037839573047,-0.361869490079316,
-0.333545859563191,-0.318750505071923,-0.313020120746328,-0.308660183205439,
-0.280670749749197,-0.274364441598121,-0.245887082486665,-0.216156157924906,
-0.204673880202647,-0.200549631865089,-0.172713963141432,-0.144949220293018,
-0.117659627928902,-0.103957135186863,-0.0999252328769017,-0.0958138230959625,
-0.0691413094734294,-0.0429166477463372,-0.0174931891367085,-0.00803968599259447,
0.),.UNSPECIFIED.);
#2693=B_SPLINE_CURVE_WITH_KNOTS('',3,(#30544,#30545,#30546,#30547,#30548,
#30549,#30550,#30551,#30552,#30553,#30554),.UNSPECIFIED.,.F.,.F.,(4,1,1,
1,1,1,1,1,4),(15.7079632679489,15.8295388729956,16.8221763756675,17.8148138783395,
18.8074513810114,19.8000888836834,20.7927263863553,21.7853638890272,21.9911485751285),
 .UNSPECIFIED.);
#2694=B_SPLINE_CURVE_WITH_KNOTS('',3,(#30555,#30556,#30557,#30558,#30559,
#30560,#30561,#30562,#30563,#30564),.UNSPECIFIED.,.F.,.F.,(4,1,1,1,1,1,
1,4),(15.7079632679489,16.3836751323157,17.3763126349877,18.3689501376596,
19.3615876403316,20.3542251430035,21.3468626456754,21.9911485751285),
 .UNSPECIFIED.);
#2695=B_SPLINE_CURVE_WITH_KNOTS('',3,(#30813,#30814,#30815,#30816,#30817,
#30818,#30819,#30820,#30821,#30822,#30823,#30824,#30825,#30826,#30827,#30828,
#30829,#30830,#30831,#30832,#30833,#30834,#30835,#30836,#30837,#30838,#30839,
#30840,#30841,#30842,#30843,#30844,#30845,#30846,#30847,#30848,#30849,#30850,
#30851,#30852,#30853,#30854,#30855,#30856,#30857,#30858,#30859,#30860,#30861,
#30862,#30863,#30864,#30865,#30866,#30867,#30868,#30869,#30870,#30871,#30872,
#30873,#30874,#30875,#30876,#30877,#30878,#30879,#30880,#30881,#30882,#30883,
#30884,#30885,#30886,#30887,#30888,#30889,#30890,#30891,#30892,#30893,#30894,
#30895,#30896,#30897,#30898,#30899,#30900,#30901,#30902,#30903),
 .UNSPECIFIED.,.F.,.F.,(4,3,3,3,3,3,3,3,3,3,3,3,3,3,3,3,3,3,3,3,3,3,3,3,
3,3,3,3,3,3,4),(0.,0.0253642096188033,0.0513998826295139,0.0781558554850298,
0.0899177895596805,0.0966255868861821,0.102679521310141,0.129980983678453,
0.157733281985931,0.184661877857859,0.195928355278117,0.202971022163091,
0.207098846486765,0.236273255980203,0.265447665473641,0.293340555515088,
0.302677577825616,0.308745367798475,0.314528755200454,0.342606729855242,
0.371727115235203,0.401175562560648,0.421351051065242,0.426753724704252,
0.456805234460622,0.481883942042153,0.490048814940579,0.498378782229001,
0.528887553514328,0.557120064786745,0.566847306048064),.UNSPECIFIED.);
#2696=B_SPLINE_CURVE_WITH_KNOTS('',3,(#30904,#30905,#30906,#30907,#30908,
#30909,#30910,#30911,#30912,#30913,#30914,#30915,#30916,#30917,#30918,#30919,
#30920,#30921,#30922,#30923,#30924,#30925,#30926,#30927,#30928),
 .UNSPECIFIED.,.F.,.F.,(4,3,3,3,3,3,3,3,4),(-10.1321597128207,-9.92637502671944,
-8.9337375240475,-7.94110002137556,-6.94846251870361,-5.95582501603167,
-4.96318751335973,-3.97055001068778,-3.84897440564114),.UNSPECIFIED.);
#2697=B_SPLINE_CURVE_WITH_KNOTS('',3,(#31177,#31178,#31179,#31180,#31181,
#31182,#31183,#31184,#31185,#31186,#31187,#31188,#31189,#31190,#31191,#31192,
#31193,#31194,#31195,#31196,#31197,#31198),.UNSPECIFIED.,.F.,.F.,(4,3,3,
3,3,3,3,4),(7.59274844815666,7.94110002137555,8.9337375240475,9.92637502671945,
10.9190125293914,11.9116500320633,12.9042875347353,13.8759337553362),
 .UNSPECIFIED.);
#2698=B_SPLINE_CURVE_WITH_KNOTS('',3,(#31199,#31200,#31201,#31202,#31203,
#31204,#31205,#31206,#31207,#31208,#31209,#31210,#31211,#31212,#31213,#31214,
#31215,#31216,#31217,#31218,#31219,#31220,#31221,#31222,#31223,#31224,#31225,
#31226,#31227,#31228,#31229,#31230,#31231,#31232,#31233,#31234,#31235,#31236,
#31237,#31238,#31239,#31240,#31241,#31242,#31243,#31244,#31245,#31246,#31247,
#31248,#31249,#31250,#31251,#31252,#31253,#31254,#31255,#31256,#31257,#31258,
#31259,#31260,#31261,#31262,#31263,#31264,#31265,#31266,#31267,#31268,#31269,
#31270,#31271,#31272,#31273,#31274,#31275,#31276,#31277,#31278,#31279,#31280,
#31281,#31282,#31283,#31284,#31285,#31286,#31287,#31288,#31289),
 .UNSPECIFIED.,.F.,.F.,(4,3,3,3,3,3,3,3,3,3,3,3,3,3,3,3,3,3,3,3,3,3,3,3,
3,3,3,3,3,3,4),(0.,0.0297250654509073,0.0601087721503145,0.0893485603866636,
0.114933375093469,0.120627515201004,0.150386819046398,0.179982111307967,
0.208493352991252,0.220471805771853,0.22888236649448,0.234177138111355,
0.264102108076231,0.292006803331058,0.294027078041107,0.322973447641599,
0.33936262260274,0.34353583112749,0.371629353805975,0.399767747163329,0.427502108378127,
0.43797083449966,0.445641199537009,0.450375060671855,0.478076750089239,
0.498853017152278,0.50825047774578,0.513369599814417,0.539284560918029,
0.561181818341393,0.569248610399432),.UNSPECIFIED.);
#3527=LINE('',#18714,#4375);
#3528=LINE('',#18723,#4376);
#3529=LINE('',#18740,#4377);
#3530=LINE('',#18791,#4378);
#3531=LINE('',#18842,#4379);
#3532=LINE('',#18890,#4380);
#3533=LINE('',#18941,#4381);
#3534=LINE('',#18992,#4382);
#3535=LINE('',#19040,#4383);
#3536=LINE('',#19091,#4384);
#3537=LINE('',#19130,#4385);
#3538=LINE('',#19154,#4386);
#3539=LINE('',#19178,#4387);
#3540=LINE('',#19203,#4388);
#3541=LINE('',#19228,#4389);
#3542=LINE('',#19252,#4390);
#3543=LINE('',#19277,#4391);
#3544=LINE('',#19302,#4392);
#3545=LINE('',#19326,#4393);
#3546=LINE('',#19343,#4394);
#3547=LINE('',#19352,#4395);
#3548=LINE('',#19369,#4396);
#3549=LINE('',#19420,#4397);
#3550=LINE('',#19471,#4398);
#3551=LINE('',#19519,#4399);
#3552=LINE('',#19570,#4400);
#3553=LINE('',#19621,#4401);
#3554=LINE('',#19669,#4402);
#3555=LINE('',#19720,#4403);
#3556=LINE('',#19759,#4404);
#3557=LINE('',#19783,#4405);
#3558=LINE('',#19807,#4406);
#3559=LINE('',#19832,#4407);
#3560=LINE('',#19857,#4408);
#3561=LINE('',#19881,#4409);
#3562=LINE('',#19906,#4410);
#3563=LINE('',#19931,#4411);
#3564=LINE('',#19955,#4412);
#3565=LINE('',#19972,#4413);
#3566=LINE('',#19981,#4414);
#3567=LINE('',#19998,#4415);
#3568=LINE('',#20049,#4416);
#3569=LINE('',#20100,#4417);
#3570=LINE('',#20148,#4418);
#3571=LINE('',#20199,#4419);
#3572=LINE('',#20250,#4420);
#3573=LINE('',#20298,#4421);
#3574=LINE('',#20349,#4422);
#3575=LINE('',#20388,#4423);
#3576=LINE('',#20412,#4424);
#3577=LINE('',#20436,#4425);
#3578=LINE('',#20461,#4426);
#3579=LINE('',#20486,#4427);
#3580=LINE('',#20510,#4428);
#3581=LINE('',#20535,#4429);
#3582=LINE('',#20560,#4430);
#3583=LINE('',#20584,#4431);
#3584=LINE('',#20601,#4432);
#3585=LINE('',#20610,#4433);
#3586=LINE('',#20627,#4434);
#3587=LINE('',#20678,#4435);
#3588=LINE('',#20729,#4436);
#3589=LINE('',#20777,#4437);
#3590=LINE('',#20828,#4438);
#3591=LINE('',#20879,#4439);
#3592=LINE('',#20927,#4440);
#3593=LINE('',#20978,#4441);
#3594=LINE('',#21017,#4442);
#3595=LINE('',#21041,#4443);
#3596=LINE('',#21065,#4444);
#3597=LINE('',#21090,#4445);
#3598=LINE('',#21115,#4446);
#3599=LINE('',#21139,#4447);
#3600=LINE('',#21164,#4448);
#3601=LINE('',#21189,#4449);
#3602=LINE('',#21213,#4450);
#3603=LINE('',#21230,#4451);
#3604=LINE('',#21239,#4452);
#3605=LINE('',#21256,#4453);
#3606=LINE('',#21307,#4454);
#3607=LINE('',#21358,#4455);
#3608=LINE('',#21406,#4456);
#3609=LINE('',#21457,#4457);
#3610=LINE('',#21508,#4458);
#3611=LINE('',#21556,#4459);
#3612=LINE('',#21607,#4460);
#3613=LINE('',#21646,#4461);
#3614=LINE('',#21670,#4462);
#3615=LINE('',#21694,#4463);
#3616=LINE('',#21719,#4464);
#3617=LINE('',#21744,#4465);
#3618=LINE('',#21768,#4466);
#3619=LINE('',#21793,#4467);
#3620=LINE('',#21818,#4468);
#3621=LINE('',#21842,#4469);
#3622=LINE('',#21859,#4470);
#3623=LINE('',#21868,#4471);
#3624=LINE('',#21885,#4472);
#3625=LINE('',#21936,#4473);
#3626=LINE('',#21987,#4474);
#3627=LINE('',#22035,#4475);
#3628=LINE('',#22086,#4476);
#3629=LINE('',#22137,#4477);
#3630=LINE('',#22185,#4478);
#3631=LINE('',#22236,#4479);
#3632=LINE('',#22275,#4480);
#3633=LINE('',#22299,#4481);
#3634=LINE('',#22323,#4482);
#3635=LINE('',#22348,#4483);
#3636=LINE('',#22373,#4484);
#3637=LINE('',#22397,#4485);
#3638=LINE('',#22422,#4486);
#3639=LINE('',#22447,#4487);
#3640=LINE('',#22471,#4488);
#3641=LINE('',#22488,#4489);
#3642=LINE('',#22497,#4490);
#3643=LINE('',#22514,#4491);
#3644=LINE('',#22565,#4492);
#3645=LINE('',#22616,#4493);
#3646=LINE('',#22664,#4494);
#3647=LINE('',#22715,#4495);
#3648=LINE('',#22766,#4496);
#3649=LINE('',#22814,#4497);
#3650=LINE('',#22865,#4498);
#3651=LINE('',#22904,#4499);
#3652=LINE('',#22928,#4500);
#3653=LINE('',#22952,#4501);
#3654=LINE('',#22977,#4502);
#3655=LINE('',#23002,#4503);
#3656=LINE('',#23026,#4504);
#3657=LINE('',#23051,#4505);
#3658=LINE('',#23076,#4506);
#3659=LINE('',#23100,#4507);
#3660=LINE('',#23117,#4508);
#3661=LINE('',#23126,#4509);
#3662=LINE('',#23143,#4510);
#3663=LINE('',#23194,#4511);
#3664=LINE('',#23245,#4512);
#3665=LINE('',#23293,#4513);
#3666=LINE('',#23344,#4514);
#3667=LINE('',#23395,#4515);
#3668=LINE('',#23443,#4516);
#3669=LINE('',#23494,#4517);
#3670=LINE('',#23533,#4518);
#3671=LINE('',#23557,#4519);
#3672=LINE('',#23581,#4520);
#3673=LINE('',#23606,#4521);
#3674=LINE('',#23631,#4522);
#3675=LINE('',#23655,#4523);
#3676=LINE('',#23680,#4524);
#3677=LINE('',#23705,#4525);
#3678=LINE('',#23729,#4526);
#3679=LINE('',#23747,#4527);
#3680=LINE('',#23756,#4528);
#3681=LINE('',#23765,#4529);
#3682=LINE('',#23774,#4530);
#3683=LINE('',#23781,#4531);
#3684=LINE('',#23785,#4532);
#3685=LINE('',#23789,#4533);
#3686=LINE('',#23793,#4534);
#3687=LINE('',#31294,#4535);
#3688=LINE('',#31296,#4536);
#3689=LINE('',#31298,#4537);
#3690=LINE('',#31299,#4538);
#3691=LINE('',#31303,#4539);
#3692=LINE('',#31304,#4540);
#3693=LINE('',#31306,#4541);
#3694=LINE('',#31308,#4542);
#3695=LINE('',#31310,#4543);
#3696=LINE('',#31312,#4544);
#3697=LINE('',#31314,#4545);
#3698=LINE('',#31316,#4546);
#3699=LINE('',#31318,#4547);
#3700=LINE('',#31320,#4548);
#3701=LINE('',#31321,#4549);
#3702=LINE('',#31325,#4550);
#3703=LINE('',#31326,#4551);
#3704=LINE('',#31327,#4552);
#3705=LINE('',#31333,#4553);
#3706=LINE('',#31335,#4554);
#3707=LINE('',#31337,#4555);
#3708=LINE('',#31339,#4556);
#3709=LINE('',#31341,#4557);
#3710=LINE('',#31343,#4558);
#3711=LINE('',#31345,#4559);
#3712=LINE('',#31347,#4560);
#3713=LINE('',#31349,#4561);
#3714=LINE('',#31351,#4562);
#3715=LINE('',#31353,#4563);
#3716=LINE('',#31354,#4564);
#3717=LINE('',#31358,#4565);
#3718=LINE('',#31359,#4566);
#3719=LINE('',#31360,#4567);
#3720=LINE('',#31364,#4568);
#3721=LINE('',#31365,#4569);
#3722=LINE('',#31366,#4570);
#3723=LINE('',#31371,#4571);
#3724=LINE('',#31373,#4572);
#3725=LINE('',#31377,#4573);
#3726=LINE('',#31378,#4574);
#3727=LINE('',#31381,#4575);
#3728=LINE('',#31382,#4576);
#3729=LINE('',#31387,#4577);
#3730=LINE('',#31389,#4578);
#3731=LINE('',#31391,#4579);
#3732=LINE('',#31393,#4580);
#3733=LINE('',#31397,#4581);
#3734=LINE('',#31398,#4582);
#3735=LINE('',#31401,#4583);
#3736=LINE('',#31403,#4584);
#3737=LINE('',#31407,#4585);
#3738=LINE('',#31409,#4586);
#3739=LINE('',#31411,#4587);
#3740=LINE('',#31413,#4588);
#3741=LINE('',#31417,#4589);
#3742=LINE('',#31418,#4590);
#3743=LINE('',#31420,#4591);
#3744=LINE('',#31423,#4592);
#3745=LINE('',#31425,#4593);
#3746=LINE('',#31429,#4594);
#3747=LINE('',#31430,#4595);
#3748=LINE('',#31433,#4596);
#3749=LINE('',#31434,#4597);
#3750=LINE('',#31437,#4598);
#3751=LINE('',#31438,#4599);
#3752=LINE('',#31441,#4600);
#3753=LINE('',#31442,#4601);
#3754=LINE('',#31447,#4602);
#3755=LINE('',#31449,#4603);
#3756=LINE('',#31451,#4604);
#3757=LINE('',#31453,#4605);
#3758=LINE('',#31456,#4606);
#3759=LINE('',#31459,#4607);
#3760=LINE('',#31460,#4608);
#3761=LINE('',#31463,#4609);
#3762=LINE('',#31464,#4610);
#3763=LINE('',#31467,#4611);
#3764=LINE('',#31469,#4612);
#3765=LINE('',#31470,#4613);
#3766=LINE('',#31472,#4614);
#3767=LINE('',#31474,#4615);
#3768=LINE('',#31475,#4616);
#3769=LINE('',#31477,#4617);
#3770=LINE('',#31481,#4618);
#3771=LINE('',#31484,#4619);
#3772=LINE('',#31485,#4620);
#3773=LINE('',#31487,#4621);
#3774=LINE('',#31491,#4622);
#3775=LINE('',#31495,#4623);
#3776=LINE('',#31497,#4624);
#3777=LINE('',#31498,#4625);
#3778=LINE('',#31500,#4626);
#3779=LINE('',#31503,#4627);
#3780=LINE('',#31506,#4628);
#3781=LINE('',#31507,#4629);
#3782=LINE('',#31508,#4630);
#3783=LINE('',#31510,#4631);
#3784=LINE('',#31513,#4632);
#3785=LINE('',#31515,#4633);
#3786=LINE('',#31516,#4634);
#3787=LINE('',#31521,#4635);
#3788=LINE('',#31523,#4636);
#3789=LINE('',#31527,#4637);
#3790=LINE('',#31529,#4638);
#3791=LINE('',#31531,#4639);
#3792=LINE('',#31533,#4640);
#3793=LINE('',#31535,#4641);
#3794=LINE('',#31537,#4642);
#3795=LINE('',#31538,#4643);
#3796=LINE('',#31539,#4644);
#3797=LINE('',#31541,#4645);
#3798=LINE('',#31544,#4646);
#3799=LINE('',#31546,#4647);
#3800=LINE('',#31547,#4648);
#3801=LINE('',#31550,#4649);
#3802=LINE('',#31552,#4650);
#3803=LINE('',#31554,#4651);
#3804=LINE('',#31556,#4652);
#3805=LINE('',#31558,#4653);
#3806=LINE('',#31560,#4654);
#3807=LINE('',#31562,#4655);
#3808=LINE('',#31564,#4656);
#3809=LINE('',#31566,#4657);
#3810=LINE('',#31567,#4658);
#3811=LINE('',#31571,#4659);
#3812=LINE('',#31572,#4660);
#3813=LINE('',#31573,#4661);
#3814=LINE('',#31577,#4662);
#3815=LINE('',#31578,#4663);
#3816=LINE('',#31581,#4664);
#3817=LINE('',#31582,#4665);
#3818=LINE('',#31584,#4666);
#3819=LINE('',#31587,#4667);
#3820=LINE('',#31592,#4668);
#3821=LINE('',#31593,#4669);
#3822=LINE('',#31595,#4670);
#3823=LINE('',#31596,#4671);
#3824=LINE('',#31599,#4672);
#3825=LINE('',#31600,#4673);
#3826=LINE('',#31602,#4674);
#3827=LINE('',#31604,#4675);
#3828=LINE('',#31605,#4676);
#3829=LINE('',#31606,#4677);
#3830=LINE('',#31608,#4678);
#3831=LINE('',#31610,#4679);
#3832=LINE('',#31611,#4680);
#3833=LINE('',#31612,#4681);
#3834=LINE('',#31614,#4682);
#3835=LINE('',#31616,#4683);
#3836=LINE('',#31617,#4684);
#3837=LINE('',#31621,#4685);
#3838=LINE('',#31622,#4686);
#3839=LINE('',#31625,#4687);
#3840=LINE('',#31629,#4688);
#3841=LINE('',#31635,#4689);
#4375=VECTOR('',#15869,3.);
#4376=VECTOR('',#15872,3.);
#4377=VECTOR('',#15879,3.);
#4378=VECTOR('',#15882,3.);
#4379=VECTOR('',#15885,3.);
#4380=VECTOR('',#15888,3.);
#4381=VECTOR('',#15891,3.);
#4382=VECTOR('',#15894,3.);
#4383=VECTOR('',#15897,3.);
#4384=VECTOR('',#15900,3.);
#4385=VECTOR('',#15905,3.0735);
#4386=VECTOR('',#15910,3.0735);
#4387=VECTOR('',#15913,3.0735);
#4388=VECTOR('',#15916,3.0735);
#4389=VECTOR('',#15919,3.0735);
#4390=VECTOR('',#15922,3.0735);
#4391=VECTOR('',#15925,3.0735);
#4392=VECTOR('',#15928,3.0735);
#4393=VECTOR('',#15931,3.0735);
#4394=VECTOR('',#15936,3.);
#4395=VECTOR('',#15939,3.);
#4396=VECTOR('',#15946,3.);
#4397=VECTOR('',#15949,3.);
#4398=VECTOR('',#15952,3.);
#4399=VECTOR('',#15955,3.);
#4400=VECTOR('',#15958,3.);
#4401=VECTOR('',#15961,3.);
#4402=VECTOR('',#15964,3.);
#4403=VECTOR('',#15967,3.);
#4404=VECTOR('',#15972,3.0735);
#4405=VECTOR('',#15977,3.0735);
#4406=VECTOR('',#15980,3.0735);
#4407=VECTOR('',#15983,3.0735);
#4408=VECTOR('',#15986,3.0735);
#4409=VECTOR('',#15989,3.0735);
#4410=VECTOR('',#15992,3.0735);
#4411=VECTOR('',#15995,3.0735);
#4412=VECTOR('',#15998,3.0735);
#4413=VECTOR('',#16003,3.);
#4414=VECTOR('',#16006,3.);
#4415=VECTOR('',#16013,3.);
#4416=VECTOR('',#16016,3.);
#4417=VECTOR('',#16019,3.);
#4418=VECTOR('',#16022,3.);
#4419=VECTOR('',#16025,3.);
#4420=VECTOR('',#16028,3.);
#4421=VECTOR('',#16031,3.);
#4422=VECTOR('',#16034,3.);
#4423=VECTOR('',#16039,3.0735);
#4424=VECTOR('',#16044,3.0735);
#4425=VECTOR('',#16047,3.0735);
#4426=VECTOR('',#16050,3.0735);
#4427=VECTOR('',#16053,3.0735);
#4428=VECTOR('',#16056,3.0735);
#4429=VECTOR('',#16059,3.0735);
#4430=VECTOR('',#16062,3.0735);
#4431=VECTOR('',#16065,3.0735);
#4432=VECTOR('',#16070,3.);
#4433=VECTOR('',#16073,3.);
#4434=VECTOR('',#16080,3.);
#4435=VECTOR('',#16083,3.);
#4436=VECTOR('',#16086,3.);
#4437=VECTOR('',#16089,3.);
#4438=VECTOR('',#16092,3.);
#4439=VECTOR('',#16095,3.);
#4440=VECTOR('',#16098,3.);
#4441=VECTOR('',#16101,3.);
#4442=VECTOR('',#16106,3.0735);
#4443=VECTOR('',#16111,3.0735);
#4444=VECTOR('',#16114,3.0735);
#4445=VECTOR('',#16117,3.0735);
#4446=VECTOR('',#16120,3.0735);
#4447=VECTOR('',#16123,3.0735);
#4448=VECTOR('',#16126,3.0735);
#4449=VECTOR('',#16129,3.0735);
#4450=VECTOR('',#16132,3.0735);
#4451=VECTOR('',#16137,3.);
#4452=VECTOR('',#16140,3.);
#4453=VECTOR('',#16147,3.);
#4454=VECTOR('',#16150,3.);
#4455=VECTOR('',#16153,3.);
#4456=VECTOR('',#16156,3.);
#4457=VECTOR('',#16159,3.);
#4458=VECTOR('',#16162,3.);
#4459=VECTOR('',#16165,3.);
#4460=VECTOR('',#16168,3.);
#4461=VECTOR('',#16173,3.0735);
#4462=VECTOR('',#16178,3.0735);
#4463=VECTOR('',#16181,3.0735);
#4464=VECTOR('',#16184,3.0735);
#4465=VECTOR('',#16187,3.0735);
#4466=VECTOR('',#16190,3.0735);
#4467=VECTOR('',#16193,3.0735);
#4468=VECTOR('',#16196,3.0735);
#4469=VECTOR('',#16199,3.0735);
#4470=VECTOR('',#16204,3.);
#4471=VECTOR('',#16207,3.);
#4472=VECTOR('',#16214,3.);
#4473=VECTOR('',#16217,3.);
#4474=VECTOR('',#16220,3.);
#4475=VECTOR('',#16223,3.);
#4476=VECTOR('',#16226,3.);
#4477=VECTOR('',#16229,3.);
#4478=VECTOR('',#16232,3.);
#4479=VECTOR('',#16235,3.);
#4480=VECTOR('',#16240,3.0735);
#4481=VECTOR('',#16245,3.0735);
#4482=VECTOR('',#16248,3.0735);
#4483=VECTOR('',#16251,3.0735);
#4484=VECTOR('',#16254,3.0735);
#4485=VECTOR('',#16257,3.0735);
#4486=VECTOR('',#16260,3.0735);
#4487=VECTOR('',#16263,3.0735);
#4488=VECTOR('',#16266,3.0735);
#4489=VECTOR('',#16271,3.);
#4490=VECTOR('',#16274,3.);
#4491=VECTOR('',#16281,3.);
#4492=VECTOR('',#16284,3.);
#4493=VECTOR('',#16287,3.);
#4494=VECTOR('',#16290,3.);
#4495=VECTOR('',#16293,3.);
#4496=VECTOR('',#16296,3.);
#4497=VECTOR('',#16299,3.);
#4498=VECTOR('',#16302,3.);
#4499=VECTOR('',#16307,3.0735);
#4500=VECTOR('',#16312,3.0735);
#4501=VECTOR('',#16315,3.0735);
#4502=VECTOR('',#16318,3.0735);
#4503=VECTOR('',#16321,3.0735);
#4504=VECTOR('',#16324,3.0735);
#4505=VECTOR('',#16327,3.0735);
#4506=VECTOR('',#16330,3.0735);
#4507=VECTOR('',#16333,3.0735);
#4508=VECTOR('',#16338,3.);
#4509=VECTOR('',#16341,3.);
#4510=VECTOR('',#16348,3.);
#4511=VECTOR('',#16351,3.);
#4512=VECTOR('',#16354,3.);
#4513=VECTOR('',#16357,3.);
#4514=VECTOR('',#16360,3.);
#4515=VECTOR('',#16363,3.);
#4516=VECTOR('',#16366,3.);
#4517=VECTOR('',#16369,3.);
#4518=VECTOR('',#16374,3.0735);
#4519=VECTOR('',#16379,3.0735);
#4520=VECTOR('',#16382,3.0735);
#4521=VECTOR('',#16385,3.0735);
#4522=VECTOR('',#16388,3.0735);
#4523=VECTOR('',#16391,3.0735);
#4524=VECTOR('',#16394,3.0735);
#4525=VECTOR('',#16397,3.0735);
#4526=VECTOR('',#16400,3.0735);
#4527=VECTOR('',#16407,7.);
#4528=VECTOR('',#16418,7.);
#4529=VECTOR('',#16429,7.);
#4530=VECTOR('',#16440,7.);
#4531=VECTOR('',#16449,4.5);
#4532=VECTOR('',#16454,4.5);
#4533=VECTOR('',#16459,4.5);
#4534=VECTOR('',#16464,4.5);
#4535=VECTOR('',#16517,10.);
#4536=VECTOR('',#16518,10.);
#4537=VECTOR('',#16519,10.);
#4538=VECTOR('',#16520,10.);
#4539=VECTOR('',#16523,10.);
#4540=VECTOR('',#16524,10.);
#4541=VECTOR('',#16525,10.);
#4542=VECTOR('',#16526,10.);
#4543=VECTOR('',#16527,10.);
#4544=VECTOR('',#16528,10.);
#4545=VECTOR('',#16529,10.);
#4546=VECTOR('',#16530,10.);
#4547=VECTOR('',#16531,10.);
#4548=VECTOR('',#16532,10.);
#4549=VECTOR('',#16533,10.);
#4550=VECTOR('',#16536,10.);
#4551=VECTOR('',#16537,10.);
#4552=VECTOR('',#16538,10.);
#4553=VECTOR('',#16545,10.);
#4554=VECTOR('',#16546,10.);
#4555=VECTOR('',#16547,10.);
#4556=VECTOR('',#16548,10.);
#4557=VECTOR('',#16549,10.);
#4558=VECTOR('',#16550,10.);
#4559=VECTOR('',#16551,10.);
#4560=VECTOR('',#16552,10.);
#4561=VECTOR('',#16553,10.);
#4562=VECTOR('',#16554,10.);
#4563=VECTOR('',#16555,10.);
#4564=VECTOR('',#16556,10.);
#4565=VECTOR('',#16559,10.);
#4566=VECTOR('',#16560,10.);
#4567=VECTOR('',#16561,10.);
#4568=VECTOR('',#16564,10.);
#4569=VECTOR('',#16565,10.);
#4570=VECTOR('',#16566,10.);
#4571=VECTOR('',#16573,10.);
#4572=VECTOR('',#16574,10.);
#4573=VECTOR('',#16577,10.);
#4574=VECTOR('',#16578,10.);
#4575=VECTOR('',#16581,10.);
#4576=VECTOR('',#16582,10.);
#4577=VECTOR('',#16587,10.);
#4578=VECTOR('',#16588,10.);
#4579=VECTOR('',#16589,10.);
#4580=VECTOR('',#16590,10.);
#4581=VECTOR('',#16593,10.);
#4582=VECTOR('',#16594,10.);
#4583=VECTOR('',#16597,10.);
#4584=VECTOR('',#16598,10.);
#4585=VECTOR('',#16601,10.);
#4586=VECTOR('',#16602,10.);
#4587=VECTOR('',#16603,10.);
#4588=VECTOR('',#16604,10.);
#4589=VECTOR('',#16609,10.);
#4590=VECTOR('',#16610,10.);
#4591=VECTOR('',#16613,10.);
#4592=VECTOR('',#16616,10.);
#4593=VECTOR('',#16617,10.);
#4594=VECTOR('',#16620,10.);
#4595=VECTOR('',#16621,10.);
#4596=VECTOR('',#16624,10.);
#4597=VECTOR('',#16625,10.);
#4598=VECTOR('',#16628,10.);
#4599=VECTOR('',#16629,10.);
#4600=VECTOR('',#16632,10.);
#4601=VECTOR('',#16633,10.);
#4602=VECTOR('',#16638,10.);
#4603=VECTOR('',#16639,10.);
#4604=VECTOR('',#16640,10.);
#4605=VECTOR('',#16641,10.);
#4606=VECTOR('',#16644,10.);
#4607=VECTOR('',#16647,10.);
#4608=VECTOR('',#16648,10.);
#4609=VECTOR('',#16651,10.);
#4610=VECTOR('',#16652,10.);
#4611=VECTOR('',#16655,10.);
#4612=VECTOR('',#16656,10.);
#4613=VECTOR('',#16657,10.);
#4614=VECTOR('',#16660,10.);
#4615=VECTOR('',#16663,10.);
#4616=VECTOR('',#16664,10.);
#4617=VECTOR('',#16665,10.);
#4618=VECTOR('',#16668,10.);
#4619=VECTOR('',#16671,10.);
#4620=VECTOR('',#16672,10.);
#4621=VECTOR('',#16673,10.);
#4622=VECTOR('',#16676,20.);
#4623=VECTOR('',#16681,10.);
#4624=VECTOR('',#16684,10.);
#4625=VECTOR('',#16685,10.);
#4626=VECTOR('',#16688,10.);
#4627=VECTOR('',#16693,10.);
#4628=VECTOR('',#16696,10.);
#4629=VECTOR('',#16697,10.);
#4630=VECTOR('',#16698,10.);
#4631=VECTOR('',#16701,10.);
#4632=VECTOR('',#16704,10.);
#4633=VECTOR('',#16705,10.);
#4634=VECTOR('',#16706,10.);
#4635=VECTOR('',#16711,10.);
#4636=VECTOR('',#16712,10.);
#4637=VECTOR('',#16717,10.);
#4638=VECTOR('',#16718,10.);
#4639=VECTOR('',#16719,10.);
#4640=VECTOR('',#16720,10.);
#4641=VECTOR('',#16721,10.);
#4642=VECTOR('',#16722,10.);
#4643=VECTOR('',#16723,10.);
#4644=VECTOR('',#16724,10.);
#4645=VECTOR('',#16727,10.);
#4646=VECTOR('',#16730,10.);
#4647=VECTOR('',#16731,10.);
#4648=VECTOR('',#16732,10.);
#4649=VECTOR('',#16735,10.);
#4650=VECTOR('',#16736,10.);
#4651=VECTOR('',#16737,10.);
#4652=VECTOR('',#16738,10.);
#4653=VECTOR('',#16739,10.);
#4654=VECTOR('',#16740,10.);
#4655=VECTOR('',#16741,10.);
#4656=VECTOR('',#16742,10.);
#4657=VECTOR('',#16743,10.);
#4658=VECTOR('',#16744,10.);
#4659=VECTOR('',#16747,10.);
#4660=VECTOR('',#16748,10.);
#4661=VECTOR('',#16749,10.);
#4662=VECTOR('',#16756,10.);
#4663=VECTOR('',#16757,10.);
#4664=VECTOR('',#16760,10.);
#4665=VECTOR('',#16761,10.);
#4666=VECTOR('',#16764,10.);
#4667=VECTOR('',#16767,100.);
#4668=VECTOR('',#16774,10.);
#4669=VECTOR('',#16775,10.);
#4670=VECTOR('',#16778,10.);
#4671=VECTOR('',#16779,10.);
#4672=VECTOR('',#16782,10.);
#4673=VECTOR('',#16783,10.);
#4674=VECTOR('',#16786,10.);
#4675=VECTOR('',#16789,10.);
#4676=VECTOR('',#16790,10.);
#4677=VECTOR('',#16791,10.);
#4678=VECTOR('',#16794,10.);
#4679=VECTOR('',#16797,10.);
#4680=VECTOR('',#16798,10.);
#4681=VECTOR('',#16799,10.);
#4682=VECTOR('',#16802,10.);
#4683=VECTOR('',#16803,10.);
#4684=VECTOR('',#16804,10.);
#4685=VECTOR('',#16809,10.);
#4686=VECTOR('',#16810,10.);
#4687=VECTOR('',#16815,10.);
#4688=VECTOR('',#16822,10.);
#4689=VECTOR('',#16829,40.);
#5223=VERTEX_POINT('',#18712);
#5224=VERTEX_POINT('',#18713);
#5225=VERTEX_POINT('',#18715);
#5226=VERTEX_POINT('',#18720);
#5227=VERTEX_POINT('',#18722);
#5228=VERTEX_POINT('',#18725);
#5229=VERTEX_POINT('',#18738);
#5230=VERTEX_POINT('',#18739);
#5231=VERTEX_POINT('',#18789);
#5232=VERTEX_POINT('',#18790);
#5233=VERTEX_POINT('',#18840);
#5234=VERTEX_POINT('',#18841);
#5235=VERTEX_POINT('',#18888);
#5236=VERTEX_POINT('',#18889);
#5237=VERTEX_POINT('',#18939);
#5238=VERTEX_POINT('',#18940);
#5239=VERTEX_POINT('',#18990);
#5240=VERTEX_POINT('',#18991);
#5241=VERTEX_POINT('',#19038);
#5242=VERTEX_POINT('',#19039);
#5243=VERTEX_POINT('',#19089);
#5244=VERTEX_POINT('',#19090);
#5245=VERTEX_POINT('',#19092);
#5246=VERTEX_POINT('',#19106);
#5247=VERTEX_POINT('',#19128);
#5248=VERTEX_POINT('',#19129);
#5249=VERTEX_POINT('',#19131);
#5250=VERTEX_POINT('',#19140);
#5251=VERTEX_POINT('',#19152);
#5252=VERTEX_POINT('',#19153);
#5253=VERTEX_POINT('',#19176);
#5254=VERTEX_POINT('',#19177);
#5255=VERTEX_POINT('',#19201);
#5256=VERTEX_POINT('',#19202);
#5257=VERTEX_POINT('',#19226);
#5258=VERTEX_POINT('',#19227);
#5259=VERTEX_POINT('',#19250);
#5260=VERTEX_POINT('',#19251);
#5261=VERTEX_POINT('',#19275);
#5262=VERTEX_POINT('',#19276);
#5263=VERTEX_POINT('',#19300);
#5264=VERTEX_POINT('',#19301);
#5265=VERTEX_POINT('',#19324);
#5266=VERTEX_POINT('',#19325);
#5267=VERTEX_POINT('',#19327);
#5268=VERTEX_POINT('',#19333);
#5269=VERTEX_POINT('',#19341);
#5270=VERTEX_POINT('',#19342);
#5271=VERTEX_POINT('',#19344);
#5272=VERTEX_POINT('',#19349);
#5273=VERTEX_POINT('',#19351);
#5274=VERTEX_POINT('',#19354);
#5275=VERTEX_POINT('',#19367);
#5276=VERTEX_POINT('',#19368);
#5277=VERTEX_POINT('',#19418);
#5278=VERTEX_POINT('',#19419);
#5279=VERTEX_POINT('',#19469);
#5280=VERTEX_POINT('',#19470);
#5281=VERTEX_POINT('',#19517);
#5282=VERTEX_POINT('',#19518);
#5283=VERTEX_POINT('',#19568);
#5284=VERTEX_POINT('',#19569);
#5285=VERTEX_POINT('',#19619);
#5286=VERTEX_POINT('',#19620);
#5287=VERTEX_POINT('',#19667);
#5288=VERTEX_POINT('',#19668);
#5289=VERTEX_POINT('',#19718);
#5290=VERTEX_POINT('',#19719);
#5291=VERTEX_POINT('',#19721);
#5292=VERTEX_POINT('',#19735);
#5293=VERTEX_POINT('',#19757);
#5294=VERTEX_POINT('',#19758);
#5295=VERTEX_POINT('',#19760);
#5296=VERTEX_POINT('',#19769);
#5297=VERTEX_POINT('',#19781);
#5298=VERTEX_POINT('',#19782);
#5299=VERTEX_POINT('',#19805);
#5300=VERTEX_POINT('',#19806);
#5301=VERTEX_POINT('',#19830);
#5302=VERTEX_POINT('',#19831);
#5303=VERTEX_POINT('',#19855);
#5304=VERTEX_POINT('',#19856);
#5305=VERTEX_POINT('',#19879);
#5306=VERTEX_POINT('',#19880);
#5307=VERTEX_POINT('',#19904);
#5308=VERTEX_POINT('',#19905);
#5309=VERTEX_POINT('',#19929);
#5310=VERTEX_POINT('',#19930);
#5311=VERTEX_POINT('',#19953);
#5312=VERTEX_POINT('',#19954);
#5313=VERTEX_POINT('',#19956);
#5314=VERTEX_POINT('',#19962);
#5315=VERTEX_POINT('',#19970);
#5316=VERTEX_POINT('',#19971);
#5317=VERTEX_POINT('',#19973);
#5318=VERTEX_POINT('',#19978);
#5319=VERTEX_POINT('',#19980);
#5320=VERTEX_POINT('',#19983);
#5321=VERTEX_POINT('',#19996);
#5322=VERTEX_POINT('',#19997);
#5323=VERTEX_POINT('',#20047);
#5324=VERTEX_POINT('',#20048);
#5325=VERTEX_POINT('',#20098);
#5326=VERTEX_POINT('',#20099);
#5327=VERTEX_POINT('',#20146);
#5328=VERTEX_POINT('',#20147);
#5329=VERTEX_POINT('',#20197);
#5330=VERTEX_POINT('',#20198);
#5331=VERTEX_POINT('',#20248);
#5332=VERTEX_POINT('',#20249);
#5333=VERTEX_POINT('',#20296);
#5334=VERTEX_POINT('',#20297);
#5335=VERTEX_POINT('',#20347);
#5336=VERTEX_POINT('',#20348);
#5337=VERTEX_POINT('',#20350);
#5338=VERTEX_POINT('',#20364);
#5339=VERTEX_POINT('',#20386);
#5340=VERTEX_POINT('',#20387);
#5341=VERTEX_POINT('',#20389);
#5342=VERTEX_POINT('',#20398);
#5343=VERTEX_POINT('',#20410);
#5344=VERTEX_POINT('',#20411);
#5345=VERTEX_POINT('',#20434);
#5346=VERTEX_POINT('',#20435);
#5347=VERTEX_POINT('',#20459);
#5348=VERTEX_POINT('',#20460);
#5349=VERTEX_POINT('',#20484);
#5350=VERTEX_POINT('',#20485);
#5351=VERTEX_POINT('',#20508);
#5352=VERTEX_POINT('',#20509);
#5353=VERTEX_POINT('',#20533);
#5354=VERTEX_POINT('',#20534);
#5355=VERTEX_POINT('',#20558);
#5356=VERTEX_POINT('',#20559);
#5357=VERTEX_POINT('',#20582);
#5358=VERTEX_POINT('',#20583);
#5359=VERTEX_POINT('',#20585);
#5360=VERTEX_POINT('',#20591);
#5361=VERTEX_POINT('',#20599);
#5362=VERTEX_POINT('',#20600);
#5363=VERTEX_POINT('',#20602);
#5364=VERTEX_POINT('',#20607);
#5365=VERTEX_POINT('',#20609);
#5366=VERTEX_POINT('',#20612);
#5367=VERTEX_POINT('',#20625);
#5368=VERTEX_POINT('',#20626);
#5369=VERTEX_POINT('',#20676);
#5370=VERTEX_POINT('',#20677);
#5371=VERTEX_POINT('',#20727);
#5372=VERTEX_POINT('',#20728);
#5373=VERTEX_POINT('',#20775);
#5374=VERTEX_POINT('',#20776);
#5375=VERTEX_POINT('',#20826);
#5376=VERTEX_POINT('',#20827);
#5377=VERTEX_POINT('',#20877);
#5378=VERTEX_POINT('',#20878);
#5379=VERTEX_POINT('',#20925);
#5380=VERTEX_POINT('',#20926);
#5381=VERTEX_POINT('',#20976);
#5382=VERTEX_POINT('',#20977);
#5383=VERTEX_POINT('',#20979);
#5384=VERTEX_POINT('',#20993);
#5385=VERTEX_POINT('',#21015);
#5386=VERTEX_POINT('',#21016);
#5387=VERTEX_POINT('',#21018);
#5388=VERTEX_POINT('',#21027);
#5389=VERTEX_POINT('',#21039);
#5390=VERTEX_POINT('',#21040);
#5391=VERTEX_POINT('',#21063);
#5392=VERTEX_POINT('',#21064);
#5393=VERTEX_POINT('',#21088);
#5394=VERTEX_POINT('',#21089);
#5395=VERTEX_POINT('',#21113);
#5396=VERTEX_POINT('',#21114);
#5397=VERTEX_POINT('',#21137);
#5398=VERTEX_POINT('',#21138);
#5399=VERTEX_POINT('',#21162);
#5400=VERTEX_POINT('',#21163);
#5401=VERTEX_POINT('',#21187);
#5402=VERTEX_POINT('',#21188);
#5403=VERTEX_POINT('',#21211);
#5404=VERTEX_POINT('',#21212);
#5405=VERTEX_POINT('',#21214);
#5406=VERTEX_POINT('',#21220);
#5407=VERTEX_POINT('',#21228);
#5408=VERTEX_POINT('',#21229);
#5409=VERTEX_POINT('',#21231);
#5410=VERTEX_POINT('',#21236);
#5411=VERTEX_POINT('',#21238);
#5412=VERTEX_POINT('',#21241);
#5413=VERTEX_POINT('',#21254);
#5414=VERTEX_POINT('',#21255);
#5415=VERTEX_POINT('',#21305);
#5416=VERTEX_POINT('',#21306);
#5417=VERTEX_POINT('',#21356);
#5418=VERTEX_POINT('',#21357);
#5419=VERTEX_POINT('',#21404);
#5420=VERTEX_POINT('',#21405);
#5421=VERTEX_POINT('',#21455);
#5422=VERTEX_POINT('',#21456);
#5423=VERTEX_POINT('',#21506);
#5424=VERTEX_POINT('',#21507);
#5425=VERTEX_POINT('',#21554);
#5426=VERTEX_POINT('',#21555);
#5427=VERTEX_POINT('',#21605);
#5428=VERTEX_POINT('',#21606);
#5429=VERTEX_POINT('',#21608);
#5430=VERTEX_POINT('',#21622);
#5431=VERTEX_POINT('',#21644);
#5432=VERTEX_POINT('',#21645);
#5433=VERTEX_POINT('',#21647);
#5434=VERTEX_POINT('',#21656);
#5435=VERTEX_POINT('',#21668);
#5436=VERTEX_POINT('',#21669);
#5437=VERTEX_POINT('',#21692);
#5438=VERTEX_POINT('',#21693);
#5439=VERTEX_POINT('',#21717);
#5440=VERTEX_POINT('',#21718);
#5441=VERTEX_POINT('',#21742);
#5442=VERTEX_POINT('',#21743);
#5443=VERTEX_POINT('',#21766);
#5444=VERTEX_POINT('',#21767);
#5445=VERTEX_POINT('',#21791);
#5446=VERTEX_POINT('',#21792);
#5447=VERTEX_POINT('',#21816);
#5448=VERTEX_POINT('',#21817);
#5449=VERTEX_POINT('',#21840);
#5450=VERTEX_POINT('',#21841);
#5451=VERTEX_POINT('',#21843);
#5452=VERTEX_POINT('',#21849);
#5453=VERTEX_POINT('',#21857);
#5454=VERTEX_POINT('',#21858);
#5455=VERTEX_POINT('',#21860);
#5456=VERTEX_POINT('',#21865);
#5457=VERTEX_POINT('',#21867);
#5458=VERTEX_POINT('',#21870);
#5459=VERTEX_POINT('',#21883);
#5460=VERTEX_POINT('',#21884);
#5461=VERTEX_POINT('',#21934);
#5462=VERTEX_POINT('',#21935);
#5463=VERTEX_POINT('',#21985);
#5464=VERTEX_POINT('',#21986);
#5465=VERTEX_POINT('',#22033);
#5466=VERTEX_POINT('',#22034);
#5467=VERTEX_POINT('',#22084);
#5468=VERTEX_POINT('',#22085);
#5469=VERTEX_POINT('',#22135);
#5470=VERTEX_POINT('',#22136);
#5471=VERTEX_POINT('',#22183);
#5472=VERTEX_POINT('',#22184);
#5473=VERTEX_POINT('',#22234);
#5474=VERTEX_POINT('',#22235);
#5475=VERTEX_POINT('',#22237);
#5476=VERTEX_POINT('',#22251);
#5477=VERTEX_POINT('',#22273);
#5478=VERTEX_POINT('',#22274);
#5479=VERTEX_POINT('',#22276);
#5480=VERTEX_POINT('',#22285);
#5481=VERTEX_POINT('',#22297);
#5482=VERTEX_POINT('',#22298);
#5483=VERTEX_POINT('',#22321);
#5484=VERTEX_POINT('',#22322);
#5485=VERTEX_POINT('',#22346);
#5486=VERTEX_POINT('',#22347);
#5487=VERTEX_POINT('',#22371);
#5488=VERTEX_POINT('',#22372);
#5489=VERTEX_POINT('',#22395);
#5490=VERTEX_POINT('',#22396);
#5491=VERTEX_POINT('',#22420);
#5492=VERTEX_POINT('',#22421);
#5493=VERTEX_POINT('',#22445);
#5494=VERTEX_POINT('',#22446);
#5495=VERTEX_POINT('',#22469);
#5496=VERTEX_POINT('',#22470);
#5497=VERTEX_POINT('',#22472);
#5498=VERTEX_POINT('',#22478);
#5499=VERTEX_POINT('',#22486);
#5500=VERTEX_POINT('',#22487);
#5501=VERTEX_POINT('',#22489);
#5502=VERTEX_POINT('',#22494);
#5503=VERTEX_POINT('',#22496);
#5504=VERTEX_POINT('',#22499);
#5505=VERTEX_POINT('',#22512);
#5506=VERTEX_POINT('',#22513);
#5507=VERTEX_POINT('',#22563);
#5508=VERTEX_POINT('',#22564);
#5509=VERTEX_POINT('',#22614);
#5510=VERTEX_POINT('',#22615);
#5511=VERTEX_POINT('',#22662);
#5512=VERTEX_POINT('',#22663);
#5513=VERTEX_POINT('',#22713);
#5514=VERTEX_POINT('',#22714);
#5515=VERTEX_POINT('',#22764);
#5516=VERTEX_POINT('',#22765);
#5517=VERTEX_POINT('',#22812);
#5518=VERTEX_POINT('',#22813);
#5519=VERTEX_POINT('',#22863);
#5520=VERTEX_POINT('',#22864);
#5521=VERTEX_POINT('',#22866);
#5522=VERTEX_POINT('',#22880);
#5523=VERTEX_POINT('',#22902);
#5524=VERTEX_POINT('',#22903);
#5525=VERTEX_POINT('',#22905);
#5526=VERTEX_POINT('',#22914);
#5527=VERTEX_POINT('',#22926);
#5528=VERTEX_POINT('',#22927);
#5529=VERTEX_POINT('',#22950);
#5530=VERTEX_POINT('',#22951);
#5531=VERTEX_POINT('',#22975);
#5532=VERTEX_POINT('',#22976);
#5533=VERTEX_POINT('',#23000);
#5534=VERTEX_POINT('',#23001);
#5535=VERTEX_POINT('',#23024);
#5536=VERTEX_POINT('',#23025);
#5537=VERTEX_POINT('',#23049);
#5538=VERTEX_POINT('',#23050);
#5539=VERTEX_POINT('',#23074);
#5540=VERTEX_POINT('',#23075);
#5541=VERTEX_POINT('',#23098);
#5542=VERTEX_POINT('',#23099);
#5543=VERTEX_POINT('',#23101);
#5544=VERTEX_POINT('',#23107);
#5545=VERTEX_POINT('',#23115);
#5546=VERTEX_POINT('',#23116);
#5547=VERTEX_POINT('',#23118);
#5548=VERTEX_POINT('',#23123);
#5549=VERTEX_POINT('',#23125);
#5550=VERTEX_POINT('',#23128);
#5551=VERTEX_POINT('',#23141);
#5552=VERTEX_POINT('',#23142);
#5553=VERTEX_POINT('',#23192);
#5554=VERTEX_POINT('',#23193);
#5555=VERTEX_POINT('',#23243);
#5556=VERTEX_POINT('',#23244);
#5557=VERTEX_POINT('',#23291);
#5558=VERTEX_POINT('',#23292);
#5559=VERTEX_POINT('',#23342);
#5560=VERTEX_POINT('',#23343);
#5561=VERTEX_POINT('',#23393);
#5562=VERTEX_POINT('',#23394);
#5563=VERTEX_POINT('',#23441);
#5564=VERTEX_POINT('',#23442);
#5565=VERTEX_POINT('',#23492);
#5566=VERTEX_POINT('',#23493);
#5567=VERTEX_POINT('',#23495);
#5568=VERTEX_POINT('',#23509);
#5569=VERTEX_POINT('',#23531);
#5570=VERTEX_POINT('',#23532);
#5571=VERTEX_POINT('',#23534);
#5572=VERTEX_POINT('',#23543);
#5573=VERTEX_POINT('',#23555);
#5574=VERTEX_POINT('',#23556);
#5575=VERTEX_POINT('',#23579);
#5576=VERTEX_POINT('',#23580);
#5577=VERTEX_POINT('',#23604);
#5578=VERTEX_POINT('',#23605);
#5579=VERTEX_POINT('',#23629);
#5580=VERTEX_POINT('',#23630);
#5581=VERTEX_POINT('',#23653);
#5582=VERTEX_POINT('',#23654);
#5583=VERTEX_POINT('',#23678);
#5584=VERTEX_POINT('',#23679);
#5585=VERTEX_POINT('',#23703);
#5586=VERTEX_POINT('',#23704);
#5587=VERTEX_POINT('',#23727);
#5588=VERTEX_POINT('',#23728);
#5589=VERTEX_POINT('',#23730);
#5590=VERTEX_POINT('',#23736);
#5591=VERTEX_POINT('',#23744);
#5592=VERTEX_POINT('',#23746);
#5593=VERTEX_POINT('',#23750);
#5594=VERTEX_POINT('',#23753);
#5595=VERTEX_POINT('',#23755);
#5596=VERTEX_POINT('',#23759);
#5597=VERTEX_POINT('',#23762);
#5598=VERTEX_POINT('',#23764);
#5599=VERTEX_POINT('',#23768);
#5600=VERTEX_POINT('',#23771);
#5601=VERTEX_POINT('',#23773);
#5602=VERTEX_POINT('',#23777);
#5603=VERTEX_POINT('',#23780);
#5604=VERTEX_POINT('',#23784);
#5605=VERTEX_POINT('',#23788);
#5606=VERTEX_POINT('',#23792);
#5607=VERTEX_POINT('',#31292);
#5608=VERTEX_POINT('',#31293);
#5609=VERTEX_POINT('',#31295);
#5610=VERTEX_POINT('',#31297);
#5611=VERTEX_POINT('',#31301);
#5612=VERTEX_POINT('',#31302);
#5613=VERTEX_POINT('',#31305);
#5614=VERTEX_POINT('',#31307);
#5615=VERTEX_POINT('',#31309);
#5616=VERTEX_POINT('',#31311);
#5617=VERTEX_POINT('',#31313);
#5618=VERTEX_POINT('',#31315);
#5619=VERTEX_POINT('',#31317);
#5620=VERTEX_POINT('',#31319);
#5621=VERTEX_POINT('',#31323);
#5622=VERTEX_POINT('',#31324);
#5623=VERTEX_POINT('',#31331);
#5624=VERTEX_POINT('',#31332);
#5625=VERTEX_POINT('',#31334);
#5626=VERTEX_POINT('',#31336);
#5627=VERTEX_POINT('',#31338);
#5628=VERTEX_POINT('',#31340);
#5629=VERTEX_POINT('',#31342);
#5630=VERTEX_POINT('',#31344);
#5631=VERTEX_POINT('',#31346);
#5632=VERTEX_POINT('',#31348);
#5633=VERTEX_POINT('',#31350);
#5634=VERTEX_POINT('',#31352);
#5635=VERTEX_POINT('',#31356);
#5636=VERTEX_POINT('',#31357);
#5637=VERTEX_POINT('',#31362);
#5638=VERTEX_POINT('',#31363);
#5639=VERTEX_POINT('',#31370);
#5640=VERTEX_POINT('',#31372);
#5641=VERTEX_POINT('',#31374);
#5642=VERTEX_POINT('',#31376);
#5643=VERTEX_POINT('',#31380);
#5644=VERTEX_POINT('',#31384);
#5645=VERTEX_POINT('',#31386);
#5646=VERTEX_POINT('',#31388);
#5647=VERTEX_POINT('',#31390);
#5648=VERTEX_POINT('',#31392);
#5649=VERTEX_POINT('',#31394);
#5650=VERTEX_POINT('',#31396);
#5651=VERTEX_POINT('',#31400);
#5652=VERTEX_POINT('',#31402);
#5653=VERTEX_POINT('',#31404);
#5654=VERTEX_POINT('',#31406);
#5655=VERTEX_POINT('',#31408);
#5656=VERTEX_POINT('',#31410);
#5657=VERTEX_POINT('',#31412);
#5658=VERTEX_POINT('',#31416);
#5659=VERTEX_POINT('',#31422);
#5660=VERTEX_POINT('',#31424);
#5661=VERTEX_POINT('',#31426);
#5662=VERTEX_POINT('',#31428);
#5663=VERTEX_POINT('',#31432);
#5664=VERTEX_POINT('',#31436);
#5665=VERTEX_POINT('',#31440);
#5666=VERTEX_POINT('',#31444);
#5667=VERTEX_POINT('',#31446);
#5668=VERTEX_POINT('',#31448);
#5669=VERTEX_POINT('',#31450);
#5670=VERTEX_POINT('',#31452);
#5671=VERTEX_POINT('',#31454);
#5672=VERTEX_POINT('',#31458);
#5673=VERTEX_POINT('',#31462);
#5674=VERTEX_POINT('',#31466);
#5675=VERTEX_POINT('',#31468);
#5676=VERTEX_POINT('',#31476);
#5677=VERTEX_POINT('',#31478);
#5678=VERTEX_POINT('',#31480);
#5679=VERTEX_POINT('',#31482);
#5680=VERTEX_POINT('',#31486);
#5681=VERTEX_POINT('',#31488);
#5682=VERTEX_POINT('',#31490);
#5683=VERTEX_POINT('',#31493);
#5684=VERTEX_POINT('',#31505);
#5685=VERTEX_POINT('',#31512);
#5686=VERTEX_POINT('',#31514);
#5687=VERTEX_POINT('',#31518);
#5688=VERTEX_POINT('',#31520);
#5689=VERTEX_POINT('',#31522);
#5690=VERTEX_POINT('',#31526);
#5691=VERTEX_POINT('',#31528);
#5692=VERTEX_POINT('',#31530);
#5693=VERTEX_POINT('',#31532);
#5694=VERTEX_POINT('',#31534);
#5695=VERTEX_POINT('',#31536);
#5696=VERTEX_POINT('',#31543);
#5697=VERTEX_POINT('',#31545);
#5698=VERTEX_POINT('',#31549);
#5699=VERTEX_POINT('',#31551);
#5700=VERTEX_POINT('',#31553);
#5701=VERTEX_POINT('',#31555);
#5702=VERTEX_POINT('',#31557);
#5703=VERTEX_POINT('',#31559);
#5704=VERTEX_POINT('',#31561);
#5705=VERTEX_POINT('',#31563);
#5706=VERTEX_POINT('',#31565);
#5707=VERTEX_POINT('',#31569);
#5708=VERTEX_POINT('',#31570);
#5709=VERTEX_POINT('',#31580);
#5710=VERTEX_POINT('',#31586);
#5711=VERTEX_POINT('',#31591);
#5712=VERTEX_POINT('',#31598);
#5713=VERTEX_POINT('',#31615);
#5714=VERTEX_POINT('',#31620);
#5715=VERTEX_POINT('',#31632);
#5716=VERTEX_POINT('',#31634);
#6697=EDGE_CURVE('',#5223,#5224,#3527,.T.);
#6698=EDGE_CURVE('',#5224,#5225,#2347,.T.);
#6699=EDGE_CURVE('',#5225,#5226,#2151,.T.);
#6700=EDGE_CURVE('',#5226,#5227,#3528,.T.);
#6701=EDGE_CURVE('',#5227,#5227,#2152,.F.);
#6702=EDGE_CURVE('',#5226,#5228,#2153,.T.);
#6703=EDGE_CURVE('',#5228,#5223,#2348,.T.);
#6704=EDGE_CURVE('',#5229,#5230,#3529,.T.);
#6705=EDGE_CURVE('',#5230,#5224,#2349,.T.);
#6706=EDGE_CURVE('',#5223,#5229,#2350,.T.);
#6707=EDGE_CURVE('',#5231,#5232,#3530,.T.);
#6708=EDGE_CURVE('',#5232,#5230,#2351,.T.);
#6709=EDGE_CURVE('',#5229,#5231,#2352,.T.);
#6710=EDGE_CURVE('',#5233,#5234,#3531,.T.);
#6711=EDGE_CURVE('',#5234,#5232,#2353,.T.);
#6712=EDGE_CURVE('',#5231,#5233,#2354,.T.);
#6713=EDGE_CURVE('',#5235,#5236,#3532,.T.);
#6714=EDGE_CURVE('',#5236,#5234,#2355,.T.);
#6715=EDGE_CURVE('',#5233,#5235,#2356,.T.);
#6716=EDGE_CURVE('',#5237,#5238,#3533,.T.);
#6717=EDGE_CURVE('',#5238,#5236,#2357,.T.);
#6718=EDGE_CURVE('',#5235,#5237,#2358,.T.);
#6719=EDGE_CURVE('',#5239,#5240,#3534,.T.);
#6720=EDGE_CURVE('',#5240,#5238,#2359,.T.);
#6721=EDGE_CURVE('',#5237,#5239,#2360,.T.);
#6722=EDGE_CURVE('',#5241,#5242,#3535,.T.);
#6723=EDGE_CURVE('',#5242,#5240,#2361,.T.);
#6724=EDGE_CURVE('',#5239,#5241,#2362,.T.);
#6725=EDGE_CURVE('',#5243,#5244,#3536,.T.);
#6726=EDGE_CURVE('',#5243,#5245,#2363,.T.);
#6727=EDGE_CURVE('',#5246,#5245,#2154,.F.);
#6728=EDGE_CURVE('',#5246,#5244,#2364,.T.);
#6729=EDGE_CURVE('',#5247,#5248,#3537,.T.);
#6730=EDGE_CURVE('',#5248,#5249,#2365,.T.);
#6731=EDGE_CURVE('',#5250,#5249,#2155,.T.);
#6732=EDGE_CURVE('',#5247,#5250,#2366,.T.);
#6733=EDGE_CURVE('',#5251,#5252,#3538,.T.);
#6734=EDGE_CURVE('',#5252,#5248,#2367,.T.);
#6735=EDGE_CURVE('',#5251,#5247,#2368,.T.);
#6736=EDGE_CURVE('',#5253,#5254,#3539,.T.);
#6737=EDGE_CURVE('',#5254,#5252,#2369,.T.);
#6738=EDGE_CURVE('',#5253,#5251,#2370,.T.);
#6739=EDGE_CURVE('',#5255,#5256,#3540,.T.);
#6740=EDGE_CURVE('',#5256,#5254,#2371,.T.);
#6741=EDGE_CURVE('',#5255,#5253,#2372,.T.);
#6742=EDGE_CURVE('',#5257,#5258,#3541,.T.);
#6743=EDGE_CURVE('',#5258,#5256,#2373,.T.);
#6744=EDGE_CURVE('',#5257,#5255,#2374,.T.);
#6745=EDGE_CURVE('',#5259,#5260,#3542,.T.);
#6746=EDGE_CURVE('',#5260,#5258,#2375,.T.);
#6747=EDGE_CURVE('',#5259,#5257,#2376,.T.);
#6748=EDGE_CURVE('',#5261,#5262,#3543,.T.);
#6749=EDGE_CURVE('',#5262,#5260,#2377,.T.);
#6750=EDGE_CURVE('',#5261,#5259,#2378,.T.);
#6751=EDGE_CURVE('',#5263,#5264,#3544,.T.);
#6752=EDGE_CURVE('',#5264,#5262,#2379,.T.);
#6753=EDGE_CURVE('',#5263,#5261,#2380,.T.);
#6754=EDGE_CURVE('',#5265,#5266,#3545,.T.);
#6755=EDGE_CURVE('',#5267,#5265,#2381,.T.);
#6756=EDGE_CURVE('',#5268,#5267,#2156,.T.);
#6757=EDGE_CURVE('',#5268,#5266,#2382,.T.);
#6758=EDGE_CURVE('',#5269,#5270,#3546,.T.);
#6759=EDGE_CURVE('',#5270,#5271,#2383,.T.);
#6760=EDGE_CURVE('',#5271,#5272,#2157,.T.);
#6761=EDGE_CURVE('',#5272,#5273,#3547,.T.);
#6762=EDGE_CURVE('',#5273,#5273,#2158,.F.);
#6763=EDGE_CURVE('',#5272,#5274,#2159,.T.);
#6764=EDGE_CURVE('',#5274,#5269,#2384,.T.);
#6765=EDGE_CURVE('',#5275,#5276,#3548,.T.);
#6766=EDGE_CURVE('',#5276,#5270,#2385,.T.);
#6767=EDGE_CURVE('',#5269,#5275,#2386,.T.);
#6768=EDGE_CURVE('',#5277,#5278,#3549,.T.);
#6769=EDGE_CURVE('',#5278,#5276,#2387,.T.);
#6770=EDGE_CURVE('',#5275,#5277,#2388,.T.);
#6771=EDGE_CURVE('',#5279,#5280,#3550,.T.);
#6772=EDGE_CURVE('',#5280,#5278,#2389,.T.);
#6773=EDGE_CURVE('',#5277,#5279,#2390,.T.);
#6774=EDGE_CURVE('',#5281,#5282,#3551,.T.);
#6775=EDGE_CURVE('',#5282,#5280,#2391,.T.);
#6776=EDGE_CURVE('',#5279,#5281,#2392,.T.);
#6777=EDGE_CURVE('',#5283,#5284,#3552,.T.);
#6778=EDGE_CURVE('',#5284,#5282,#2393,.T.);
#6779=EDGE_CURVE('',#5281,#5283,#2394,.T.);
#6780=EDGE_CURVE('',#5285,#5286,#3553,.T.);
#6781=EDGE_CURVE('',#5286,#5284,#2395,.T.);
#6782=EDGE_CURVE('',#5283,#5285,#2396,.T.);
#6783=EDGE_CURVE('',#5287,#5288,#3554,.T.);
#6784=EDGE_CURVE('',#5288,#5286,#2397,.T.);
#6785=EDGE_CURVE('',#5285,#5287,#2398,.T.);
#6786=EDGE_CURVE('',#5289,#5290,#3555,.T.);
#6787=EDGE_CURVE('',#5289,#5291,#2399,.T.);
#6788=EDGE_CURVE('',#5292,#5291,#2160,.F.);
#6789=EDGE_CURVE('',#5292,#5290,#2400,.T.);
#6790=EDGE_CURVE('',#5293,#5294,#3556,.T.);
#6791=EDGE_CURVE('',#5294,#5295,#2401,.T.);
#6792=EDGE_CURVE('',#5296,#5295,#2161,.T.);
#6793=EDGE_CURVE('',#5293,#5296,#2402,.T.);
#6794=EDGE_CURVE('',#5297,#5298,#3557,.T.);
#6795=EDGE_CURVE('',#5298,#5294,#2403,.T.);
#6796=EDGE_CURVE('',#5297,#5293,#2404,.T.);
#6797=EDGE_CURVE('',#5299,#5300,#3558,.T.);
#6798=EDGE_CURVE('',#5300,#5298,#2405,.T.);
#6799=EDGE_CURVE('',#5299,#5297,#2406,.T.);
#6800=EDGE_CURVE('',#5301,#5302,#3559,.T.);
#6801=EDGE_CURVE('',#5302,#5300,#2407,.T.);
#6802=EDGE_CURVE('',#5301,#5299,#2408,.T.);
#6803=EDGE_CURVE('',#5303,#5304,#3560,.T.);
#6804=EDGE_CURVE('',#5304,#5302,#2409,.T.);
#6805=EDGE_CURVE('',#5303,#5301,#2410,.T.);
#6806=EDGE_CURVE('',#5305,#5306,#3561,.T.);
#6807=EDGE_CURVE('',#5306,#5304,#2411,.T.);
#6808=EDGE_CURVE('',#5305,#5303,#2412,.T.);
#6809=EDGE_CURVE('',#5307,#5308,#3562,.T.);
#6810=EDGE_CURVE('',#5308,#5306,#2413,.T.);
#6811=EDGE_CURVE('',#5307,#5305,#2414,.T.);
#6812=EDGE_CURVE('',#5309,#5310,#3563,.T.);
#6813=EDGE_CURVE('',#5310,#5308,#2415,.T.);
#6814=EDGE_CURVE('',#5309,#5307,#2416,.T.);
#6815=EDGE_CURVE('',#5311,#5312,#3564,.T.);
#6816=EDGE_CURVE('',#5313,#5311,#2417,.T.);
#6817=EDGE_CURVE('',#5314,#5313,#2162,.T.);
#6818=EDGE_CURVE('',#5314,#5312,#2418,.T.);
#6819=EDGE_CURVE('',#5315,#5316,#3565,.T.);
#6820=EDGE_CURVE('',#5316,#5317,#2419,.T.);
#6821=EDGE_CURVE('',#5317,#5318,#2163,.T.);
#6822=EDGE_CURVE('',#5318,#5319,#3566,.T.);
#6823=EDGE_CURVE('',#5319,#5319,#2164,.F.);
#6824=EDGE_CURVE('',#5318,#5320,#2165,.T.);
#6825=EDGE_CURVE('',#5320,#5315,#2420,.T.);
#6826=EDGE_CURVE('',#5321,#5322,#3567,.T.);
#6827=EDGE_CURVE('',#5322,#5316,#2421,.T.);
#6828=EDGE_CURVE('',#5315,#5321,#2422,.T.);
#6829=EDGE_CURVE('',#5323,#5324,#3568,.T.);
#6830=EDGE_CURVE('',#5324,#5322,#2423,.T.);
#6831=EDGE_CURVE('',#5321,#5323,#2424,.T.);
#6832=EDGE_CURVE('',#5325,#5326,#3569,.T.);
#6833=EDGE_CURVE('',#5326,#5324,#2425,.T.);
#6834=EDGE_CURVE('',#5323,#5325,#2426,.T.);
#6835=EDGE_CURVE('',#5327,#5328,#3570,.T.);
#6836=EDGE_CURVE('',#5328,#5326,#2427,.T.);
#6837=EDGE_CURVE('',#5325,#5327,#2428,.T.);
#6838=EDGE_CURVE('',#5329,#5330,#3571,.T.);
#6839=EDGE_CURVE('',#5330,#5328,#2429,.T.);
#6840=EDGE_CURVE('',#5327,#5329,#2430,.T.);
#6841=EDGE_CURVE('',#5331,#5332,#3572,.T.);
#6842=EDGE_CURVE('',#5332,#5330,#2431,.T.);
#6843=EDGE_CURVE('',#5329,#5331,#2432,.T.);
#6844=EDGE_CURVE('',#5333,#5334,#3573,.T.);
#6845=EDGE_CURVE('',#5334,#5332,#2433,.T.);
#6846=EDGE_CURVE('',#5331,#5333,#2434,.T.);
#6847=EDGE_CURVE('',#5335,#5336,#3574,.T.);
#6848=EDGE_CURVE('',#5335,#5337,#2435,.T.);
#6849=EDGE_CURVE('',#5338,#5337,#2166,.F.);
#6850=EDGE_CURVE('',#5338,#5336,#2436,.T.);
#6851=EDGE_CURVE('',#5339,#5340,#3575,.T.);
#6852=EDGE_CURVE('',#5340,#5341,#2437,.T.);
#6853=EDGE_CURVE('',#5342,#5341,#2167,.T.);
#6854=EDGE_CURVE('',#5339,#5342,#2438,.T.);
#6855=EDGE_CURVE('',#5343,#5344,#3576,.T.);
#6856=EDGE_CURVE('',#5344,#5340,#2439,.T.);
#6857=EDGE_CURVE('',#5343,#5339,#2440,.T.);
#6858=EDGE_CURVE('',#5345,#5346,#3577,.T.);
#6859=EDGE_CURVE('',#5346,#5344,#2441,.T.);
#6860=EDGE_CURVE('',#5345,#5343,#2442,.T.);
#6861=EDGE_CURVE('',#5347,#5348,#3578,.T.);
#6862=EDGE_CURVE('',#5348,#5346,#2443,.T.);
#6863=EDGE_CURVE('',#5347,#5345,#2444,.T.);
#6864=EDGE_CURVE('',#5349,#5350,#3579,.T.);
#6865=EDGE_CURVE('',#5350,#5348,#2445,.T.);
#6866=EDGE_CURVE('',#5349,#5347,#2446,.T.);
#6867=EDGE_CURVE('',#5351,#5352,#3580,.T.);
#6868=EDGE_CURVE('',#5352,#5350,#2447,.T.);
#6869=EDGE_CURVE('',#5351,#5349,#2448,.T.);
#6870=EDGE_CURVE('',#5353,#5354,#3581,.T.);
#6871=EDGE_CURVE('',#5354,#5352,#2449,.T.);
#6872=EDGE_CURVE('',#5353,#5351,#2450,.T.);
#6873=EDGE_CURVE('',#5355,#5356,#3582,.T.);
#6874=EDGE_CURVE('',#5356,#5354,#2451,.T.);
#6875=EDGE_CURVE('',#5355,#5353,#2452,.T.);
#6876=EDGE_CURVE('',#5357,#5358,#3583,.T.);
#6877=EDGE_CURVE('',#5359,#5357,#2453,.T.);
#6878=EDGE_CURVE('',#5360,#5359,#2168,.T.);
#6879=EDGE_CURVE('',#5360,#5358,#2454,.T.);
#6880=EDGE_CURVE('',#5361,#5362,#3584,.T.);
#6881=EDGE_CURVE('',#5362,#5363,#2455,.T.);
#6882=EDGE_CURVE('',#5363,#5364,#2169,.T.);
#6883=EDGE_CURVE('',#5364,#5365,#3585,.T.);
#6884=EDGE_CURVE('',#5365,#5365,#2170,.F.);
#6885=EDGE_CURVE('',#5364,#5366,#2171,.T.);
#6886=EDGE_CURVE('',#5366,#5361,#2456,.T.);
#6887=EDGE_CURVE('',#5367,#5368,#3586,.T.);
#6888=EDGE_CURVE('',#5368,#5362,#2457,.T.);
#6889=EDGE_CURVE('',#5361,#5367,#2458,.T.);
#6890=EDGE_CURVE('',#5369,#5370,#3587,.T.);
#6891=EDGE_CURVE('',#5370,#5368,#2459,.T.);
#6892=EDGE_CURVE('',#5367,#5369,#2460,.T.);
#6893=EDGE_CURVE('',#5371,#5372,#3588,.T.);
#6894=EDGE_CURVE('',#5372,#5370,#2461,.T.);
#6895=EDGE_CURVE('',#5369,#5371,#2462,.T.);
#6896=EDGE_CURVE('',#5373,#5374,#3589,.T.);
#6897=EDGE_CURVE('',#5374,#5372,#2463,.T.);
#6898=EDGE_CURVE('',#5371,#5373,#2464,.T.);
#6899=EDGE_CURVE('',#5375,#5376,#3590,.T.);
#6900=EDGE_CURVE('',#5376,#5374,#2465,.T.);
#6901=EDGE_CURVE('',#5373,#5375,#2466,.T.);
#6902=EDGE_CURVE('',#5377,#5378,#3591,.T.);
#6903=EDGE_CURVE('',#5378,#5376,#2467,.T.);
#6904=EDGE_CURVE('',#5375,#5377,#2468,.T.);
#6905=EDGE_CURVE('',#5379,#5380,#3592,.T.);
#6906=EDGE_CURVE('',#5380,#5378,#2469,.T.);
#6907=EDGE_CURVE('',#5377,#5379,#2470,.T.);
#6908=EDGE_CURVE('',#5381,#5382,#3593,.T.);
#6909=EDGE_CURVE('',#5381,#5383,#2471,.T.);
#6910=EDGE_CURVE('',#5384,#5383,#2172,.F.);
#6911=EDGE_CURVE('',#5384,#5382,#2472,.T.);
#6912=EDGE_CURVE('',#5385,#5386,#3594,.T.);
#6913=EDGE_CURVE('',#5386,#5387,#2473,.T.);
#6914=EDGE_CURVE('',#5388,#5387,#2173,.T.);
#6915=EDGE_CURVE('',#5385,#5388,#2474,.T.);
#6916=EDGE_CURVE('',#5389,#5390,#3595,.T.);
#6917=EDGE_CURVE('',#5390,#5386,#2475,.T.);
#6918=EDGE_CURVE('',#5389,#5385,#2476,.T.);
#6919=EDGE_CURVE('',#5391,#5392,#3596,.T.);
#6920=EDGE_CURVE('',#5392,#5390,#2477,.T.);
#6921=EDGE_CURVE('',#5391,#5389,#2478,.T.);
#6922=EDGE_CURVE('',#5393,#5394,#3597,.T.);
#6923=EDGE_CURVE('',#5394,#5392,#2479,.T.);
#6924=EDGE_CURVE('',#5393,#5391,#2480,.T.);
#6925=EDGE_CURVE('',#5395,#5396,#3598,.T.);
#6926=EDGE_CURVE('',#5396,#5394,#2481,.T.);
#6927=EDGE_CURVE('',#5395,#5393,#2482,.T.);
#6928=EDGE_CURVE('',#5397,#5398,#3599,.T.);
#6929=EDGE_CURVE('',#5398,#5396,#2483,.T.);
#6930=EDGE_CURVE('',#5397,#5395,#2484,.T.);
#6931=EDGE_CURVE('',#5399,#5400,#3600,.T.);
#6932=EDGE_CURVE('',#5400,#5398,#2485,.T.);
#6933=EDGE_CURVE('',#5399,#5397,#2486,.T.);
#6934=EDGE_CURVE('',#5401,#5402,#3601,.T.);
#6935=EDGE_CURVE('',#5402,#5400,#2487,.T.);
#6936=EDGE_CURVE('',#5401,#5399,#2488,.T.);
#6937=EDGE_CURVE('',#5403,#5404,#3602,.T.);
#6938=EDGE_CURVE('',#5405,#5403,#2489,.T.);
#6939=EDGE_CURVE('',#5406,#5405,#2174,.T.);
#6940=EDGE_CURVE('',#5406,#5404,#2490,.T.);
#6941=EDGE_CURVE('',#5407,#5408,#3603,.T.);
#6942=EDGE_CURVE('',#5408,#5409,#2491,.T.);
#6943=EDGE_CURVE('',#5409,#5410,#2175,.T.);
#6944=EDGE_CURVE('',#5410,#5411,#3604,.T.);
#6945=EDGE_CURVE('',#5411,#5411,#2176,.F.);
#6946=EDGE_CURVE('',#5410,#5412,#2177,.T.);
#6947=EDGE_CURVE('',#5412,#5407,#2492,.T.);
#6948=EDGE_CURVE('',#5413,#5414,#3605,.T.);
#6949=EDGE_CURVE('',#5414,#5408,#2493,.T.);
#6950=EDGE_CURVE('',#5407,#5413,#2494,.T.);
#6951=EDGE_CURVE('',#5415,#5416,#3606,.T.);
#6952=EDGE_CURVE('',#5416,#5414,#2495,.T.);
#6953=EDGE_CURVE('',#5413,#5415,#2496,.T.);
#6954=EDGE_CURVE('',#5417,#5418,#3607,.T.);
#6955=EDGE_CURVE('',#5418,#5416,#2497,.T.);
#6956=EDGE_CURVE('',#5415,#5417,#2498,.T.);
#6957=EDGE_CURVE('',#5419,#5420,#3608,.T.);
#6958=EDGE_CURVE('',#5420,#5418,#2499,.T.);
#6959=EDGE_CURVE('',#5417,#5419,#2500,.T.);
#6960=EDGE_CURVE('',#5421,#5422,#3609,.T.);
#6961=EDGE_CURVE('',#5422,#5420,#2501,.T.);
#6962=EDGE_CURVE('',#5419,#5421,#2502,.T.);
#6963=EDGE_CURVE('',#5423,#5424,#3610,.T.);
#6964=EDGE_CURVE('',#5424,#5422,#2503,.T.);
#6965=EDGE_CURVE('',#5421,#5423,#2504,.T.);
#6966=EDGE_CURVE('',#5425,#5426,#3611,.T.);
#6967=EDGE_CURVE('',#5426,#5424,#2505,.T.);
#6968=EDGE_CURVE('',#5423,#5425,#2506,.T.);
#6969=EDGE_CURVE('',#5427,#5428,#3612,.T.);
#6970=EDGE_CURVE('',#5427,#5429,#2507,.T.);
#6971=EDGE_CURVE('',#5430,#5429,#2178,.F.);
#6972=EDGE_CURVE('',#5430,#5428,#2508,.T.);
#6973=EDGE_CURVE('',#5431,#5432,#3613,.T.);
#6974=EDGE_CURVE('',#5432,#5433,#2509,.T.);
#6975=EDGE_CURVE('',#5434,#5433,#2179,.T.);
#6976=EDGE_CURVE('',#5431,#5434,#2510,.T.);
#6977=EDGE_CURVE('',#5435,#5436,#3614,.T.);
#6978=EDGE_CURVE('',#5436,#5432,#2511,.T.);
#6979=EDGE_CURVE('',#5435,#5431,#2512,.T.);
#6980=EDGE_CURVE('',#5437,#5438,#3615,.T.);
#6981=EDGE_CURVE('',#5438,#5436,#2513,.T.);
#6982=EDGE_CURVE('',#5437,#5435,#2514,.T.);
#6983=EDGE_CURVE('',#5439,#5440,#3616,.T.);
#6984=EDGE_CURVE('',#5440,#5438,#2515,.T.);
#6985=EDGE_CURVE('',#5439,#5437,#2516,.T.);
#6986=EDGE_CURVE('',#5441,#5442,#3617,.T.);
#6987=EDGE_CURVE('',#5442,#5440,#2517,.T.);
#6988=EDGE_CURVE('',#5441,#5439,#2518,.T.);
#6989=EDGE_CURVE('',#5443,#5444,#3618,.T.);
#6990=EDGE_CURVE('',#5444,#5442,#2519,.T.);
#6991=EDGE_CURVE('',#5443,#5441,#2520,.T.);
#6992=EDGE_CURVE('',#5445,#5446,#3619,.T.);
#6993=EDGE_CURVE('',#5446,#5444,#2521,.T.);
#6994=EDGE_CURVE('',#5445,#5443,#2522,.T.);
#6995=EDGE_CURVE('',#5447,#5448,#3620,.T.);
#6996=EDGE_CURVE('',#5448,#5446,#2523,.T.);
#6997=EDGE_CURVE('',#5447,#5445,#2524,.T.);
#6998=EDGE_CURVE('',#5449,#5450,#3621,.T.);
#6999=EDGE_CURVE('',#5451,#5449,#2525,.T.);
#7000=EDGE_CURVE('',#5452,#5451,#2180,.T.);
#7001=EDGE_CURVE('',#5452,#5450,#2526,.T.);
#7002=EDGE_CURVE('',#5453,#5454,#3622,.T.);
#7003=EDGE_CURVE('',#5454,#5455,#2527,.T.);
#7004=EDGE_CURVE('',#5455,#5456,#2181,.T.);
#7005=EDGE_CURVE('',#5456,#5457,#3623,.T.);
#7006=EDGE_CURVE('',#5457,#5457,#2182,.F.);
#7007=EDGE_CURVE('',#5456,#5458,#2183,.T.);
#7008=EDGE_CURVE('',#5458,#5453,#2528,.T.);
#7009=EDGE_CURVE('',#5459,#5460,#3624,.T.);
#7010=EDGE_CURVE('',#5460,#5454,#2529,.T.);
#7011=EDGE_CURVE('',#5453,#5459,#2530,.T.);
#7012=EDGE_CURVE('',#5461,#5462,#3625,.T.);
#7013=EDGE_CURVE('',#5462,#5460,#2531,.T.);
#7014=EDGE_CURVE('',#5459,#5461,#2532,.T.);
#7015=EDGE_CURVE('',#5463,#5464,#3626,.T.);
#7016=EDGE_CURVE('',#5464,#5462,#2533,.T.);
#7017=EDGE_CURVE('',#5461,#5463,#2534,.T.);
#7018=EDGE_CURVE('',#5465,#5466,#3627,.T.);
#7019=EDGE_CURVE('',#5466,#5464,#2535,.T.);
#7020=EDGE_CURVE('',#5463,#5465,#2536,.T.);
#7021=EDGE_CURVE('',#5467,#5468,#3628,.T.);
#7022=EDGE_CURVE('',#5468,#5466,#2537,.T.);
#7023=EDGE_CURVE('',#5465,#5467,#2538,.T.);
#7024=EDGE_CURVE('',#5469,#5470,#3629,.T.);
#7025=EDGE_CURVE('',#5470,#5468,#2539,.T.);
#7026=EDGE_CURVE('',#5467,#5469,#2540,.T.);
#7027=EDGE_CURVE('',#5471,#5472,#3630,.T.);
#7028=EDGE_CURVE('',#5472,#5470,#2541,.T.);
#7029=EDGE_CURVE('',#5469,#5471,#2542,.T.);
#7030=EDGE_CURVE('',#5473,#5474,#3631,.T.);
#7031=EDGE_CURVE('',#5473,#5475,#2543,.T.);
#7032=EDGE_CURVE('',#5476,#5475,#2184,.F.);
#7033=EDGE_CURVE('',#5476,#5474,#2544,.T.);
#7034=EDGE_CURVE('',#5477,#5478,#3632,.T.);
#7035=EDGE_CURVE('',#5478,#5479,#2545,.T.);
#7036=EDGE_CURVE('',#5480,#5479,#2185,.T.);
#7037=EDGE_CURVE('',#5477,#5480,#2546,.T.);
#7038=EDGE_CURVE('',#5481,#5482,#3633,.T.);
#7039=EDGE_CURVE('',#5482,#5478,#2547,.T.);
#7040=EDGE_CURVE('',#5481,#5477,#2548,.T.);
#7041=EDGE_CURVE('',#5483,#5484,#3634,.T.);
#7042=EDGE_CURVE('',#5484,#5482,#2549,.T.);
#7043=EDGE_CURVE('',#5483,#5481,#2550,.T.);
#7044=EDGE_CURVE('',#5485,#5486,#3635,.T.);
#7045=EDGE_CURVE('',#5486,#5484,#2551,.T.);
#7046=EDGE_CURVE('',#5485,#5483,#2552,.T.);
#7047=EDGE_CURVE('',#5487,#5488,#3636,.T.);
#7048=EDGE_CURVE('',#5488,#5486,#2553,.T.);
#7049=EDGE_CURVE('',#5487,#5485,#2554,.T.);
#7050=EDGE_CURVE('',#5489,#5490,#3637,.T.);
#7051=EDGE_CURVE('',#5490,#5488,#2555,.T.);
#7052=EDGE_CURVE('',#5489,#5487,#2556,.T.);
#7053=EDGE_CURVE('',#5491,#5492,#3638,.T.);
#7054=EDGE_CURVE('',#5492,#5490,#2557,.T.);
#7055=EDGE_CURVE('',#5491,#5489,#2558,.T.);
#7056=EDGE_CURVE('',#5493,#5494,#3639,.T.);
#7057=EDGE_CURVE('',#5494,#5492,#2559,.T.);
#7058=EDGE_CURVE('',#5493,#5491,#2560,.T.);
#7059=EDGE_CURVE('',#5495,#5496,#3640,.T.);
#7060=EDGE_CURVE('',#5497,#5495,#2561,.T.);
#7061=EDGE_CURVE('',#5498,#5497,#2186,.T.);
#7062=EDGE_CURVE('',#5498,#5496,#2562,.T.);
#7063=EDGE_CURVE('',#5499,#5500,#3641,.T.);
#7064=EDGE_CURVE('',#5500,#5501,#2563,.T.);
#7065=EDGE_CURVE('',#5501,#5502,#2187,.T.);
#7066=EDGE_CURVE('',#5502,#5503,#3642,.T.);
#7067=EDGE_CURVE('',#5503,#5503,#2188,.F.);
#7068=EDGE_CURVE('',#5502,#5504,#2189,.T.);
#7069=EDGE_CURVE('',#5504,#5499,#2564,.T.);
#7070=EDGE_CURVE('',#5505,#5506,#3643,.T.);
#7071=EDGE_CURVE('',#5506,#5500,#2565,.T.);
#7072=EDGE_CURVE('',#5499,#5505,#2566,.T.);
#7073=EDGE_CURVE('',#5507,#5508,#3644,.T.);
#7074=EDGE_CURVE('',#5508,#5506,#2567,.T.);
#7075=EDGE_CURVE('',#5505,#5507,#2568,.T.);
#7076=EDGE_CURVE('',#5509,#5510,#3645,.T.);
#7077=EDGE_CURVE('',#5510,#5508,#2569,.T.);
#7078=EDGE_CURVE('',#5507,#5509,#2570,.T.);
#7079=EDGE_CURVE('',#5511,#5512,#3646,.T.);
#7080=EDGE_CURVE('',#5512,#5510,#2571,.T.);
#7081=EDGE_CURVE('',#5509,#5511,#2572,.T.);
#7082=EDGE_CURVE('',#5513,#5514,#3647,.T.);
#7083=EDGE_CURVE('',#5514,#5512,#2573,.T.);
#7084=EDGE_CURVE('',#5511,#5513,#2574,.T.);
#7085=EDGE_CURVE('',#5515,#5516,#3648,.T.);
#7086=EDGE_CURVE('',#5516,#5514,#2575,.T.);
#7087=EDGE_CURVE('',#5513,#5515,#2576,.T.);
#7088=EDGE_CURVE('',#5517,#5518,#3649,.T.);
#7089=EDGE_CURVE('',#5518,#5516,#2577,.T.);
#7090=EDGE_CURVE('',#5515,#5517,#2578,.T.);
#7091=EDGE_CURVE('',#5519,#5520,#3650,.T.);
#7092=EDGE_CURVE('',#5519,#5521,#2579,.T.);
#7093=EDGE_CURVE('',#5522,#5521,#2190,.F.);
#7094=EDGE_CURVE('',#5522,#5520,#2580,.T.);
#7095=EDGE_CURVE('',#5523,#5524,#3651,.T.);
#7096=EDGE_CURVE('',#5524,#5525,#2581,.T.);
#7097=EDGE_CURVE('',#5526,#5525,#2191,.T.);
#7098=EDGE_CURVE('',#5523,#5526,#2582,.T.);
#7099=EDGE_CURVE('',#5527,#5528,#3652,.T.);
#7100=EDGE_CURVE('',#5528,#5524,#2583,.T.);
#7101=EDGE_CURVE('',#5527,#5523,#2584,.T.);
#7102=EDGE_CURVE('',#5529,#5530,#3653,.T.);
#7103=EDGE_CURVE('',#5530,#5528,#2585,.T.);
#7104=EDGE_CURVE('',#5529,#5527,#2586,.T.);
#7105=EDGE_CURVE('',#5531,#5532,#3654,.T.);
#7106=EDGE_CURVE('',#5532,#5530,#2587,.T.);
#7107=EDGE_CURVE('',#5531,#5529,#2588,.T.);
#7108=EDGE_CURVE('',#5533,#5534,#3655,.T.);
#7109=EDGE_CURVE('',#5534,#5532,#2589,.T.);
#7110=EDGE_CURVE('',#5533,#5531,#2590,.T.);
#7111=EDGE_CURVE('',#5535,#5536,#3656,.T.);
#7112=EDGE_CURVE('',#5536,#5534,#2591,.T.);
#7113=EDGE_CURVE('',#5535,#5533,#2592,.T.);
#7114=EDGE_CURVE('',#5537,#5538,#3657,.T.);
#7115=EDGE_CURVE('',#5538,#5536,#2593,.T.);
#7116=EDGE_CURVE('',#5537,#5535,#2594,.T.);
#7117=EDGE_CURVE('',#5539,#5540,#3658,.T.);
#7118=EDGE_CURVE('',#5540,#5538,#2595,.T.);
#7119=EDGE_CURVE('',#5539,#5537,#2596,.T.);
#7120=EDGE_CURVE('',#5541,#5542,#3659,.T.);
#7121=EDGE_CURVE('',#5543,#5541,#2597,.T.);
#7122=EDGE_CURVE('',#5544,#5543,#2192,.T.);
#7123=EDGE_CURVE('',#5544,#5542,#2598,.T.);
#7124=EDGE_CURVE('',#5545,#5546,#3660,.T.);
#7125=EDGE_CURVE('',#5546,#5547,#2599,.T.);
#7126=EDGE_CURVE('',#5547,#5548,#2193,.T.);
#7127=EDGE_CURVE('',#5548,#5549,#3661,.T.);
#7128=EDGE_CURVE('',#5549,#5549,#2194,.F.);
#7129=EDGE_CURVE('',#5548,#5550,#2195,.T.);
#7130=EDGE_CURVE('',#5550,#5545,#2600,.T.);
#7131=EDGE_CURVE('',#5551,#5552,#3662,.T.);
#7132=EDGE_CURVE('',#5552,#5546,#2601,.T.);
#7133=EDGE_CURVE('',#5545,#5551,#2602,.T.);
#7134=EDGE_CURVE('',#5553,#5554,#3663,.T.);
#7135=EDGE_CURVE('',#5554,#5552,#2603,.T.);
#7136=EDGE_CURVE('',#5551,#5553,#2604,.T.);
#7137=EDGE_CURVE('',#5555,#5556,#3664,.T.);
#7138=EDGE_CURVE('',#5556,#5554,#2605,.T.);
#7139=EDGE_CURVE('',#5553,#5555,#2606,.T.);
#7140=EDGE_CURVE('',#5557,#5558,#3665,.T.);
#7141=EDGE_CURVE('',#5558,#5556,#2607,.T.);
#7142=EDGE_CURVE('',#5555,#5557,#2608,.T.);
#7143=EDGE_CURVE('',#5559,#5560,#3666,.T.);
#7144=EDGE_CURVE('',#5560,#5558,#2609,.T.);
#7145=EDGE_CURVE('',#5557,#5559,#2610,.T.);
#7146=EDGE_CURVE('',#5561,#5562,#3667,.T.);
#7147=EDGE_CURVE('',#5562,#5560,#2611,.T.);
#7148=EDGE_CURVE('',#5559,#5561,#2612,.T.);
#7149=EDGE_CURVE('',#5563,#5564,#3668,.T.);
#7150=EDGE_CURVE('',#5564,#5562,#2613,.T.);
#7151=EDGE_CURVE('',#5561,#5563,#2614,.T.);
#7152=EDGE_CURVE('',#5565,#5566,#3669,.T.);
#7153=EDGE_CURVE('',#5565,#5567,#2615,.T.);
#7154=EDGE_CURVE('',#5568,#5567,#2196,.F.);
#7155=EDGE_CURVE('',#5568,#5566,#2616,.T.);
#7156=EDGE_CURVE('',#5569,#5570,#3670,.T.);
#7157=EDGE_CURVE('',#5570,#5571,#2617,.T.);
#7158=EDGE_CURVE('',#5572,#5571,#2197,.T.);
#7159=EDGE_CURVE('',#5569,#5572,#2618,.T.);
#7160=EDGE_CURVE('',#5573,#5574,#3671,.T.);
#7161=EDGE_CURVE('',#5574,#5570,#2619,.T.);
#7162=EDGE_CURVE('',#5573,#5569,#2620,.T.);
#7163=EDGE_CURVE('',#5575,#5576,#3672,.T.);
#7164=EDGE_CURVE('',#5576,#5574,#2621,.T.);
#7165=EDGE_CURVE('',#5575,#5573,#2622,.T.);
#7166=EDGE_CURVE('',#5577,#5578,#3673,.T.);
#7167=EDGE_CURVE('',#5578,#5576,#2623,.T.);
#7168=EDGE_CURVE('',#5577,#5575,#2624,.T.);
#7169=EDGE_CURVE('',#5579,#5580,#3674,.T.);
#7170=EDGE_CURVE('',#5580,#5578,#2625,.T.);
#7171=EDGE_CURVE('',#5579,#5577,#2626,.T.);
#7172=EDGE_CURVE('',#5581,#5582,#3675,.T.);
#7173=EDGE_CURVE('',#5582,#5580,#2627,.T.);
#7174=EDGE_CURVE('',#5581,#5579,#2628,.T.);
#7175=EDGE_CURVE('',#5583,#5584,#3676,.T.);
#7176=EDGE_CURVE('',#5584,#5582,#2629,.T.);
#7177=EDGE_CURVE('',#5583,#5581,#2630,.T.);
#7178=EDGE_CURVE('',#5585,#5586,#3677,.T.);
#7179=EDGE_CURVE('',#5586,#5584,#2631,.T.);
#7180=EDGE_CURVE('',#5585,#5583,#2632,.T.);
#7181=EDGE_CURVE('',#5587,#5588,#3678,.T.);
#7182=EDGE_CURVE('',#5589,#5587,#2633,.T.);
#7183=EDGE_CURVE('',#5590,#5589,#2198,.T.);
#7184=EDGE_CURVE('',#5590,#5588,#2634,.T.);
#7185=EDGE_CURVE('',#5591,#5591,#2199,.T.);
#7186=EDGE_CURVE('',#5591,#5592,#3679,.T.);
#7187=EDGE_CURVE('',#5592,#5592,#2200,.T.);
#7188=EDGE_CURVE('',#5593,#5593,#2201,.T.);
#7189=EDGE_CURVE('',#5594,#5594,#2202,.T.);
#7190=EDGE_CURVE('',#5594,#5595,#3680,.T.);
#7191=EDGE_CURVE('',#5595,#5595,#2203,.T.);
#7192=EDGE_CURVE('',#5596,#5596,#2204,.T.);
#7193=EDGE_CURVE('',#5597,#5597,#2205,.T.);
#7194=EDGE_CURVE('',#5597,#5598,#3681,.T.);
#7195=EDGE_CURVE('',#5598,#5598,#2206,.T.);
#7196=EDGE_CURVE('',#5599,#5599,#2207,.T.);
#7197=EDGE_CURVE('',#5600,#5600,#2208,.T.);
#7198=EDGE_CURVE('',#5600,#5601,#3682,.T.);
#7199=EDGE_CURVE('',#5601,#5601,#2209,.T.);
#7200=EDGE_CURVE('',#5602,#5602,#2210,.T.);
#7201=EDGE_CURVE('',#5593,#5603,#3683,.T.);
#7202=EDGE_CURVE('',#5603,#5603,#2211,.T.);
#7203=EDGE_CURVE('',#5596,#5604,#3684,.T.);
#7204=EDGE_CURVE('',#5604,#5604,#2212,.T.);
#7205=EDGE_CURVE('',#5599,#5605,#3685,.T.);
#7206=EDGE_CURVE('',#5605,#5605,#2213,.T.);
#7207=EDGE_CURVE('',#5602,#5606,#3686,.T.);
#7208=EDGE_CURVE('',#5606,#5606,#2214,.T.);
#7209=EDGE_CURVE('',#5547,#5572,#2635,.T.);
#7210=EDGE_CURVE('',#5571,#5550,#2636,.T.);
#7211=EDGE_CURVE('',#5588,#5586,#2637,.T.);
#7212=EDGE_CURVE('',#5587,#5585,#2638,.T.);
#7213=EDGE_CURVE('',#5567,#5590,#2639,.T.);
#7214=EDGE_CURVE('',#5563,#5565,#2640,.T.);
#7215=EDGE_CURVE('',#5566,#5564,#2641,.T.);
#7216=EDGE_CURVE('',#5589,#5568,#2642,.T.);
#7217=EDGE_CURVE('',#5501,#5526,#2643,.T.);
#7218=EDGE_CURVE('',#5525,#5504,#2644,.T.);
#7219=EDGE_CURVE('',#5542,#5540,#2645,.T.);
#7220=EDGE_CURVE('',#5541,#5539,#2646,.T.);
#7221=EDGE_CURVE('',#5521,#5544,#2647,.T.);
#7222=EDGE_CURVE('',#5517,#5519,#2648,.T.);
#7223=EDGE_CURVE('',#5520,#5518,#2649,.T.);
#7224=EDGE_CURVE('',#5543,#5522,#2650,.T.);
#7225=EDGE_CURVE('',#5455,#5480,#2651,.T.);
#7226=EDGE_CURVE('',#5479,#5458,#2652,.T.);
#7227=EDGE_CURVE('',#5496,#5494,#2653,.T.);
#7228=EDGE_CURVE('',#5495,#5493,#2654,.T.);
#7229=EDGE_CURVE('',#5475,#5498,#2655,.T.);
#7230=EDGE_CURVE('',#5471,#5473,#2656,.T.);
#7231=EDGE_CURVE('',#5474,#5472,#2657,.T.);
#7232=EDGE_CURVE('',#5497,#5476,#2658,.T.);
#7233=EDGE_CURVE('',#5409,#5434,#2659,.T.);
#7234=EDGE_CURVE('',#5433,#5412,#2660,.T.);
#7235=EDGE_CURVE('',#5450,#5448,#2661,.T.);
#7236=EDGE_CURVE('',#5449,#5447,#2662,.T.);
#7237=EDGE_CURVE('',#5429,#5452,#2663,.T.);
#7238=EDGE_CURVE('',#5425,#5427,#2664,.T.);
#7239=EDGE_CURVE('',#5428,#5426,#2665,.T.);
#7240=EDGE_CURVE('',#5451,#5430,#2666,.T.);
#7241=EDGE_CURVE('',#5363,#5388,#2667,.T.);
#7242=EDGE_CURVE('',#5387,#5366,#2668,.T.);
#7243=EDGE_CURVE('',#5404,#5402,#2669,.T.);
#7244=EDGE_CURVE('',#5403,#5401,#2670,.T.);
#7245=EDGE_CURVE('',#5383,#5406,#2671,.T.);
#7246=EDGE_CURVE('',#5379,#5381,#2672,.T.);
#7247=EDGE_CURVE('',#5382,#5380,#2673,.T.);
#7248=EDGE_CURVE('',#5405,#5384,#2674,.T.);
#7249=EDGE_CURVE('',#5317,#5342,#2675,.T.);
#7250=EDGE_CURVE('',#5341,#5320,#2676,.T.);
#7251=EDGE_CURVE('',#5358,#5356,#2677,.T.);
#7252=EDGE_CURVE('',#5357,#5355,#2678,.T.);
#7253=EDGE_CURVE('',#5337,#5360,#2679,.T.);
#7254=EDGE_CURVE('',#5333,#5335,#2680,.T.);
#7255=EDGE_CURVE('',#5336,#5334,#2681,.T.);
#7256=EDGE_CURVE('',#5359,#5338,#2682,.T.);
#7257=EDGE_CURVE('',#5271,#5296,#2683,.T.);
#7258=EDGE_CURVE('',#5295,#5274,#2684,.T.);
#7259=EDGE_CURVE('',#5312,#5310,#2685,.T.);
#7260=EDGE_CURVE('',#5311,#5309,#2686,.T.);
#7261=EDGE_CURVE('',#5291,#5314,#2687,.T.);
#7262=EDGE_CURVE('',#5287,#5289,#2688,.T.);
#7263=EDGE_CURVE('',#5290,#5288,#2689,.T.);
#7264=EDGE_CURVE('',#5313,#5292,#2690,.T.);
#7265=EDGE_CURVE('',#5225,#5250,#2691,.T.);
#7266=EDGE_CURVE('',#5249,#5228,#2692,.T.);
#7267=EDGE_CURVE('',#5266,#5264,#2693,.T.);
#7268=EDGE_CURVE('',#5265,#5263,#2694,.T.);
#7269=EDGE_CURVE('',#5245,#5268,#2695,.T.);
#7270=EDGE_CURVE('',#5241,#5243,#2696,.T.);
#7271=EDGE_CURVE('',#5244,#5242,#2697,.T.);
#7272=EDGE_CURVE('',#5267,#5246,#2698,.T.);
#7273=EDGE_CURVE('',#5607,#5608,#3687,.T.);
#7274=EDGE_CURVE('',#5607,#5609,#3688,.T.);
#7275=EDGE_CURVE('',#5610,#5609,#3689,.T.);
#7276=EDGE_CURVE('',#5608,#5610,#3690,.T.);
#7277=EDGE_CURVE('',#5611,#5612,#3691,.T.);
#7278=EDGE_CURVE('',#5610,#5611,#3692,.T.);
#7279=EDGE_CURVE('',#5609,#5613,#3693,.T.);
#7280=EDGE_CURVE('',#5614,#5613,#3694,.T.);
#7281=EDGE_CURVE('',#5615,#5614,#3695,.T.);
#7282=EDGE_CURVE('',#5616,#5615,#3696,.T.);
#7283=EDGE_CURVE('',#5617,#5616,#3697,.T.);
#7284=EDGE_CURVE('',#5618,#5617,#3698,.T.);
#7285=EDGE_CURVE('',#5619,#5618,#3699,.T.);
#7286=EDGE_CURVE('',#5620,#5619,#3700,.T.);
#7287=EDGE_CURVE('',#5612,#5620,#3701,.T.);
#7288=EDGE_CURVE('',#5621,#5622,#3702,.T.);
#7289=EDGE_CURVE('',#5614,#5621,#3703,.T.);
#7290=EDGE_CURVE('',#5613,#5622,#3704,.T.);
#7291=EDGE_CURVE('',#5622,#5607,#2215,.T.);
#7292=EDGE_CURVE('',#5623,#5624,#3705,.T.);
#7293=EDGE_CURVE('',#5625,#5623,#3706,.T.);
#7294=EDGE_CURVE('',#5625,#5626,#3707,.T.);
#7295=EDGE_CURVE('',#5626,#5627,#3708,.T.);
#7296=EDGE_CURVE('',#5628,#5627,#3709,.T.);
#7297=EDGE_CURVE('',#5629,#5628,#3710,.T.);
#7298=EDGE_CURVE('',#5630,#5629,#3711,.T.);
#7299=EDGE_CURVE('',#5631,#5630,#3712,.T.);
#7300=EDGE_CURVE('',#5632,#5631,#3713,.T.);
#7301=EDGE_CURVE('',#5633,#5632,#3714,.T.);
#7302=EDGE_CURVE('',#5634,#5633,#3715,.T.);
#7303=EDGE_CURVE('',#5624,#5634,#3716,.T.);
#7304=EDGE_CURVE('',#5635,#5636,#3717,.T.);
#7305=EDGE_CURVE('',#5635,#5626,#3718,.T.);
#7306=EDGE_CURVE('',#5636,#5625,#3719,.T.);
#7307=EDGE_CURVE('',#5637,#5638,#3720,.T.);
#7308=EDGE_CURVE('',#5628,#5637,#3721,.T.);
#7309=EDGE_CURVE('',#5627,#5638,#3722,.T.);
#7310=EDGE_CURVE('',#5638,#5635,#2216,.T.);
#7311=EDGE_CURVE('',#5639,#5618,#3723,.T.);
#7312=EDGE_CURVE('',#5640,#5639,#3724,.T.);
#7313=EDGE_CURVE('',#5641,#5640,#2217,.T.);
#7314=EDGE_CURVE('',#5642,#5641,#3725,.T.);
#7315=EDGE_CURVE('',#5619,#5642,#3726,.T.);
#7316=EDGE_CURVE('',#5617,#5643,#3727,.T.);
#7317=EDGE_CURVE('',#5643,#5639,#3728,.T.);
#7318=EDGE_CURVE('',#5621,#5644,#2218,.T.);
#7319=EDGE_CURVE('',#5644,#5645,#3729,.T.);
#7320=EDGE_CURVE('',#5645,#5646,#3730,.T.);
#7321=EDGE_CURVE('',#5646,#5647,#3731,.T.);
#7322=EDGE_CURVE('',#5647,#5648,#3732,.T.);
#7323=EDGE_CURVE('',#5648,#5649,#2219,.T.);
#7324=EDGE_CURVE('',#5649,#5650,#3733,.T.);
#7325=EDGE_CURVE('',#5650,#5615,#3734,.T.);
#7326=EDGE_CURVE('',#5611,#5651,#3735,.T.);
#7327=EDGE_CURVE('',#5651,#5652,#3736,.T.);
#7328=EDGE_CURVE('',#5652,#5653,#2220,.T.);
#7329=EDGE_CURVE('',#5653,#5654,#3737,.T.);
#7330=EDGE_CURVE('',#5654,#5655,#3738,.T.);
#7331=EDGE_CURVE('',#5655,#5656,#3739,.T.);
#7332=EDGE_CURVE('',#5656,#5657,#3740,.T.);
#7333=EDGE_CURVE('',#5657,#5608,#2221,.T.);
#7334=EDGE_CURVE('',#5658,#5616,#3741,.T.);
#7335=EDGE_CURVE('',#5643,#5658,#3742,.T.);
#7336=EDGE_CURVE('',#5650,#5658,#3743,.T.);
#7337=EDGE_CURVE('',#5659,#5632,#3744,.T.);
#7338=EDGE_CURVE('',#5660,#5659,#3745,.T.);
#7339=EDGE_CURVE('',#5661,#5660,#2222,.T.);
#7340=EDGE_CURVE('',#5662,#5661,#3746,.T.);
#7341=EDGE_CURVE('',#5633,#5662,#3747,.T.);
#7342=EDGE_CURVE('',#5631,#5663,#3748,.T.);
#7343=EDGE_CURVE('',#5663,#5659,#3749,.T.);
#7344=EDGE_CURVE('',#5664,#5630,#3750,.T.);
#7345=EDGE_CURVE('',#5663,#5664,#3751,.T.);
#7346=EDGE_CURVE('',#5665,#5629,#3752,.T.);
#7347=EDGE_CURVE('',#5665,#5664,#3753,.T.);
#7348=EDGE_CURVE('',#5637,#5666,#2223,.T.);
#7349=EDGE_CURVE('',#5666,#5667,#3754,.T.);
#7350=EDGE_CURVE('',#5667,#5668,#3755,.T.);
#7351=EDGE_CURVE('',#5668,#5669,#3756,.T.);
#7352=EDGE_CURVE('',#5669,#5670,#3757,.T.);
#7353=EDGE_CURVE('',#5670,#5671,#2224,.T.);
#7354=EDGE_CURVE('',#5671,#5665,#3758,.T.);
#7355=EDGE_CURVE('',#5672,#5642,#3759,.T.);
#7356=EDGE_CURVE('',#5672,#5620,#3760,.T.);
#7357=EDGE_CURVE('',#5673,#5672,#3761,.T.);
#7358=EDGE_CURVE('',#5612,#5673,#3762,.T.);
#7359=EDGE_CURVE('',#5674,#5634,#3763,.T.);
#7360=EDGE_CURVE('',#5675,#5674,#3764,.T.);
#7361=EDGE_CURVE('',#5624,#5675,#3765,.T.);
#7362=EDGE_CURVE('',#5674,#5662,#3766,.T.);
#7363=EDGE_CURVE('',#5652,#5641,#3767,.T.);
#7364=EDGE_CURVE('',#5640,#5649,#3768,.T.);
#7365=EDGE_CURVE('',#5648,#5676,#3769,.T.);
#7366=EDGE_CURVE('',#5676,#5677,#2225,.T.);
#7367=EDGE_CURVE('',#5677,#5678,#3770,.T.);
#7368=EDGE_CURVE('',#5679,#5678,#2226,.T.);
#7369=EDGE_CURVE('',#5679,#5661,#3771,.T.);
#7370=EDGE_CURVE('',#5660,#5671,#3772,.T.);
#7371=EDGE_CURVE('',#5670,#5680,#3773,.T.);
#7372=EDGE_CURVE('',#5680,#5681,#2227,.T.);
#7373=EDGE_CURVE('',#5681,#5682,#3774,.T.);
#7374=EDGE_CURVE('',#5682,#5682,#2228,.T.);
#7375=EDGE_CURVE('',#5681,#5683,#2229,.T.);
#7376=EDGE_CURVE('',#5683,#5653,#3775,.T.);
#7377=EDGE_CURVE('',#5651,#5673,#3776,.T.);
#7378=EDGE_CURVE('',#5672,#5642,#3777,.T.);
#7379=EDGE_CURVE('',#5643,#5639,#3778,.T.);
#7380=EDGE_CURVE('',#5663,#5659,#3779,.T.);
#7381=EDGE_CURVE('',#5684,#5679,#3780,.T.);
#7382=EDGE_CURVE('',#5684,#5675,#3781,.T.);
#7383=EDGE_CURVE('',#5674,#5662,#3782,.T.);
#7384=EDGE_CURVE('',#5623,#5684,#3783,.T.);
#7385=EDGE_CURVE('',#5657,#5685,#3784,.T.);
#7386=EDGE_CURVE('',#5656,#5686,#3785,.T.);
#7387=EDGE_CURVE('',#5686,#5685,#3786,.T.);
#7388=EDGE_CURVE('',#5685,#5687,#2230,.T.);
#7389=EDGE_CURVE('',#5688,#5686,#3787,.T.);
#7390=EDGE_CURVE('',#5689,#5688,#3788,.T.);
#7391=EDGE_CURVE('',#5687,#5689,#2231,.T.);
#7392=EDGE_CURVE('',#5690,#5655,#3789,.T.);
#7393=EDGE_CURVE('',#5691,#5690,#3790,.T.);
#7394=EDGE_CURVE('',#5692,#5691,#3791,.T.);
#7395=EDGE_CURVE('',#5693,#5692,#3792,.T.);
#7396=EDGE_CURVE('',#5694,#5693,#3793,.T.);
#7397=EDGE_CURVE('',#5695,#5694,#3794,.T.);
#7398=EDGE_CURVE('',#5668,#5695,#3795,.T.);
#7399=EDGE_CURVE('',#5667,#5688,#3796,.T.);
#7400=EDGE_CURVE('',#5689,#5666,#3797,.T.);
#7401=EDGE_CURVE('',#5696,#5644,#3798,.T.);
#7402=EDGE_CURVE('',#5696,#5697,#3799,.T.);
#7403=EDGE_CURVE('',#5645,#5697,#3800,.T.);
#7404=EDGE_CURVE('',#5646,#5698,#3801,.T.);
#7405=EDGE_CURVE('',#5697,#5699,#3802,.T.);
#7406=EDGE_CURVE('',#5700,#5699,#3803,.T.);
#7407=EDGE_CURVE('',#5701,#5700,#3804,.T.);
#7408=EDGE_CURVE('',#5702,#5701,#3805,.T.);
#7409=EDGE_CURVE('',#5703,#5702,#3806,.T.);
#7410=EDGE_CURVE('',#5704,#5703,#3807,.T.);
#7411=EDGE_CURVE('',#5705,#5704,#3808,.T.);
#7412=EDGE_CURVE('',#5706,#5705,#3809,.T.);
#7413=EDGE_CURVE('',#5698,#5706,#3810,.T.);
#7414=EDGE_CURVE('',#5707,#5708,#3811,.T.);
#7415=EDGE_CURVE('',#5700,#5707,#3812,.T.);
#7416=EDGE_CURVE('',#5699,#5708,#3813,.T.);
#7417=EDGE_CURVE('',#5708,#5696,#2232,.T.);
#7418=EDGE_CURVE('',#5691,#5672,#3814,.T.);
#7419=EDGE_CURVE('',#5642,#5692,#3815,.T.);
#7420=EDGE_CURVE('',#5709,#5690,#3816,.T.);
#7421=EDGE_CURVE('',#5672,#5709,#3817,.T.);
#7422=EDGE_CURVE('',#5654,#5709,#3818,.T.);
#7423=EDGE_CURVE('',#5687,#5710,#3819,.T.);
#7424=EDGE_CURVE('',#5710,#5710,#2233,.T.);
#7425=EDGE_CURVE('',#5707,#5636,#2234,.T.);
#7426=EDGE_CURVE('',#5698,#5711,#3820,.T.);
#7427=EDGE_CURVE('',#5647,#5711,#3821,.T.);
#7428=EDGE_CURVE('',#5643,#5706,#3822,.T.);
#7429=EDGE_CURVE('',#5711,#5643,#3823,.T.);
#7430=EDGE_CURVE('',#5678,#5712,#3824,.T.);
#7431=EDGE_CURVE('',#5712,#5701,#3825,.T.);
#7432=EDGE_CURVE('',#5705,#5639,#3826,.T.);
#7433=EDGE_CURVE('',#5662,#5704,#3827,.T.);
#7434=EDGE_CURVE('',#5677,#5662,#3828,.T.);
#7435=EDGE_CURVE('',#5639,#5676,#3829,.T.);
#7436=EDGE_CURVE('',#5703,#5674,#3830,.T.);
#7437=EDGE_CURVE('',#5683,#5642,#3831,.T.);
#7438=EDGE_CURVE('',#5659,#5680,#3832,.T.);
#7439=EDGE_CURVE('',#5693,#5659,#3833,.T.);
#7440=EDGE_CURVE('',#5663,#5694,#3834,.T.);
#7441=EDGE_CURVE('',#5713,#5663,#3835,.T.);
#7442=EDGE_CURVE('',#5695,#5713,#3836,.T.);
#7443=EDGE_CURVE('',#5714,#5702,#3837,.T.);
#7444=EDGE_CURVE('',#5674,#5714,#3838,.T.);
#7445=EDGE_CURVE('',#5669,#5713,#3839,.T.);
#7446=EDGE_CURVE('',#5712,#5714,#3840,.T.);
#7447=EDGE_CURVE('',#5715,#5715,#2235,.T.);
#7448=EDGE_CURVE('',#5715,#5716,#3841,.T.);
#7449=EDGE_CURVE('',#5716,#5716,#2236,.T.);
#8921=ORIENTED_EDGE('',*,*,#6697,.T.);
#8922=ORIENTED_EDGE('',*,*,#6698,.T.);
#8923=ORIENTED_EDGE('',*,*,#6699,.T.);
#8924=ORIENTED_EDGE('',*,*,#6700,.T.);
#8925=ORIENTED_EDGE('',*,*,#6701,.F.);
#8926=ORIENTED_EDGE('',*,*,#6700,.F.);
#8927=ORIENTED_EDGE('',*,*,#6702,.T.);
#8928=ORIENTED_EDGE('',*,*,#6703,.T.);
#8929=ORIENTED_EDGE('',*,*,#6704,.T.);
#8930=ORIENTED_EDGE('',*,*,#6705,.T.);
#8931=ORIENTED_EDGE('',*,*,#6697,.F.);
#8932=ORIENTED_EDGE('',*,*,#6706,.T.);
#8933=ORIENTED_EDGE('',*,*,#6707,.T.);
#8934=ORIENTED_EDGE('',*,*,#6708,.T.);
#8935=ORIENTED_EDGE('',*,*,#6704,.F.);
#8936=ORIENTED_EDGE('',*,*,#6709,.T.);
#8937=ORIENTED_EDGE('',*,*,#6710,.T.);
#8938=ORIENTED_EDGE('',*,*,#6711,.T.);
#8939=ORIENTED_EDGE('',*,*,#6707,.F.);
#8940=ORIENTED_EDGE('',*,*,#6712,.T.);
#8941=ORIENTED_EDGE('',*,*,#6713,.T.);
#8942=ORIENTED_EDGE('',*,*,#6714,.T.);
#8943=ORIENTED_EDGE('',*,*,#6710,.F.);
#8944=ORIENTED_EDGE('',*,*,#6715,.T.);
#8945=ORIENTED_EDGE('',*,*,#6716,.T.);
#8946=ORIENTED_EDGE('',*,*,#6717,.T.);
#8947=ORIENTED_EDGE('',*,*,#6713,.F.);
#8948=ORIENTED_EDGE('',*,*,#6718,.T.);
#8949=ORIENTED_EDGE('',*,*,#6719,.T.);
#8950=ORIENTED_EDGE('',*,*,#6720,.T.);
#8951=ORIENTED_EDGE('',*,*,#6716,.F.);
#8952=ORIENTED_EDGE('',*,*,#6721,.T.);
#8953=ORIENTED_EDGE('',*,*,#6722,.T.);
#8954=ORIENTED_EDGE('',*,*,#6723,.T.);
#8955=ORIENTED_EDGE('',*,*,#6719,.F.);
#8956=ORIENTED_EDGE('',*,*,#6724,.T.);
#8957=ORIENTED_EDGE('',*,*,#6725,.F.);
#8958=ORIENTED_EDGE('',*,*,#6726,.T.);
#8959=ORIENTED_EDGE('',*,*,#6727,.F.);
#8960=ORIENTED_EDGE('',*,*,#6728,.T.);
#8961=ORIENTED_EDGE('',*,*,#6729,.T.);
#8962=ORIENTED_EDGE('',*,*,#6730,.T.);
#8963=ORIENTED_EDGE('',*,*,#6731,.F.);
#8964=ORIENTED_EDGE('',*,*,#6732,.F.);
#8965=ORIENTED_EDGE('',*,*,#6733,.T.);
#8966=ORIENTED_EDGE('',*,*,#6734,.T.);
#8967=ORIENTED_EDGE('',*,*,#6729,.F.);
#8968=ORIENTED_EDGE('',*,*,#6735,.F.);
#8969=ORIENTED_EDGE('',*,*,#6736,.T.);
#8970=ORIENTED_EDGE('',*,*,#6737,.T.);
#8971=ORIENTED_EDGE('',*,*,#6733,.F.);
#8972=ORIENTED_EDGE('',*,*,#6738,.F.);
#8973=ORIENTED_EDGE('',*,*,#6739,.T.);
#8974=ORIENTED_EDGE('',*,*,#6740,.T.);
#8975=ORIENTED_EDGE('',*,*,#6736,.F.);
#8976=ORIENTED_EDGE('',*,*,#6741,.F.);
#8977=ORIENTED_EDGE('',*,*,#6742,.T.);
#8978=ORIENTED_EDGE('',*,*,#6743,.T.);
#8979=ORIENTED_EDGE('',*,*,#6739,.F.);
#8980=ORIENTED_EDGE('',*,*,#6744,.F.);
#8981=ORIENTED_EDGE('',*,*,#6745,.T.);
#8982=ORIENTED_EDGE('',*,*,#6746,.T.);
#8983=ORIENTED_EDGE('',*,*,#6742,.F.);
#8984=ORIENTED_EDGE('',*,*,#6747,.F.);
#8985=ORIENTED_EDGE('',*,*,#6748,.T.);
#8986=ORIENTED_EDGE('',*,*,#6749,.T.);
#8987=ORIENTED_EDGE('',*,*,#6745,.F.);
#8988=ORIENTED_EDGE('',*,*,#6750,.F.);
#8989=ORIENTED_EDGE('',*,*,#6751,.T.);
#8990=ORIENTED_EDGE('',*,*,#6752,.T.);
#8991=ORIENTED_EDGE('',*,*,#6748,.F.);
#8992=ORIENTED_EDGE('',*,*,#6753,.F.);
#8993=ORIENTED_EDGE('',*,*,#6754,.F.);
#8994=ORIENTED_EDGE('',*,*,#6755,.F.);
#8995=ORIENTED_EDGE('',*,*,#6756,.F.);
#8996=ORIENTED_EDGE('',*,*,#6757,.T.);
#8997=ORIENTED_EDGE('',*,*,#6758,.T.);
#8998=ORIENTED_EDGE('',*,*,#6759,.T.);
#8999=ORIENTED_EDGE('',*,*,#6760,.T.);
#9000=ORIENTED_EDGE('',*,*,#6761,.T.);
#9001=ORIENTED_EDGE('',*,*,#6762,.F.);
#9002=ORIENTED_EDGE('',*,*,#6761,.F.);
#9003=ORIENTED_EDGE('',*,*,#6763,.T.);
#9004=ORIENTED_EDGE('',*,*,#6764,.T.);
#9005=ORIENTED_EDGE('',*,*,#6765,.T.);
#9006=ORIENTED_EDGE('',*,*,#6766,.T.);
#9007=ORIENTED_EDGE('',*,*,#6758,.F.);
#9008=ORIENTED_EDGE('',*,*,#6767,.T.);
#9009=ORIENTED_EDGE('',*,*,#6768,.T.);
#9010=ORIENTED_EDGE('',*,*,#6769,.T.);
#9011=ORIENTED_EDGE('',*,*,#6765,.F.);
#9012=ORIENTED_EDGE('',*,*,#6770,.T.);
#9013=ORIENTED_EDGE('',*,*,#6771,.T.);
#9014=ORIENTED_EDGE('',*,*,#6772,.T.);
#9015=ORIENTED_EDGE('',*,*,#6768,.F.);
#9016=ORIENTED_EDGE('',*,*,#6773,.T.);
#9017=ORIENTED_EDGE('',*,*,#6774,.T.);
#9018=ORIENTED_EDGE('',*,*,#6775,.T.);
#9019=ORIENTED_EDGE('',*,*,#6771,.F.);
#9020=ORIENTED_EDGE('',*,*,#6776,.T.);
#9021=ORIENTED_EDGE('',*,*,#6777,.T.);
#9022=ORIENTED_EDGE('',*,*,#6778,.T.);
#9023=ORIENTED_EDGE('',*,*,#6774,.F.);
#9024=ORIENTED_EDGE('',*,*,#6779,.T.);
#9025=ORIENTED_EDGE('',*,*,#6780,.T.);
#9026=ORIENTED_EDGE('',*,*,#6781,.T.);
#9027=ORIENTED_EDGE('',*,*,#6777,.F.);
#9028=ORIENTED_EDGE('',*,*,#6782,.T.);
#9029=ORIENTED_EDGE('',*,*,#6783,.T.);
#9030=ORIENTED_EDGE('',*,*,#6784,.T.);
#9031=ORIENTED_EDGE('',*,*,#6780,.F.);
#9032=ORIENTED_EDGE('',*,*,#6785,.T.);
#9033=ORIENTED_EDGE('',*,*,#6786,.F.);
#9034=ORIENTED_EDGE('',*,*,#6787,.T.);
#9035=ORIENTED_EDGE('',*,*,#6788,.F.);
#9036=ORIENTED_EDGE('',*,*,#6789,.T.);
#9037=ORIENTED_EDGE('',*,*,#6790,.T.);
#9038=ORIENTED_EDGE('',*,*,#6791,.T.);
#9039=ORIENTED_EDGE('',*,*,#6792,.F.);
#9040=ORIENTED_EDGE('',*,*,#6793,.F.);
#9041=ORIENTED_EDGE('',*,*,#6794,.T.);
#9042=ORIENTED_EDGE('',*,*,#6795,.T.);
#9043=ORIENTED_EDGE('',*,*,#6790,.F.);
#9044=ORIENTED_EDGE('',*,*,#6796,.F.);
#9045=ORIENTED_EDGE('',*,*,#6797,.T.);
#9046=ORIENTED_EDGE('',*,*,#6798,.T.);
#9047=ORIENTED_EDGE('',*,*,#6794,.F.);
#9048=ORIENTED_EDGE('',*,*,#6799,.F.);
#9049=ORIENTED_EDGE('',*,*,#6800,.T.);
#9050=ORIENTED_EDGE('',*,*,#6801,.T.);
#9051=ORIENTED_EDGE('',*,*,#6797,.F.);
#9052=ORIENTED_EDGE('',*,*,#6802,.F.);
#9053=ORIENTED_EDGE('',*,*,#6803,.T.);
#9054=ORIENTED_EDGE('',*,*,#6804,.T.);
#9055=ORIENTED_EDGE('',*,*,#6800,.F.);
#9056=ORIENTED_EDGE('',*,*,#6805,.F.);
#9057=ORIENTED_EDGE('',*,*,#6806,.T.);
#9058=ORIENTED_EDGE('',*,*,#6807,.T.);
#9059=ORIENTED_EDGE('',*,*,#6803,.F.);
#9060=ORIENTED_EDGE('',*,*,#6808,.F.);
#9061=ORIENTED_EDGE('',*,*,#6809,.T.);
#9062=ORIENTED_EDGE('',*,*,#6810,.T.);
#9063=ORIENTED_EDGE('',*,*,#6806,.F.);
#9064=ORIENTED_EDGE('',*,*,#6811,.F.);
#9065=ORIENTED_EDGE('',*,*,#6812,.T.);
#9066=ORIENTED_EDGE('',*,*,#6813,.T.);
#9067=ORIENTED_EDGE('',*,*,#6809,.F.);
#9068=ORIENTED_EDGE('',*,*,#6814,.F.);
#9069=ORIENTED_EDGE('',*,*,#6815,.F.);
#9070=ORIENTED_EDGE('',*,*,#6816,.F.);
#9071=ORIENTED_EDGE('',*,*,#6817,.F.);
#9072=ORIENTED_EDGE('',*,*,#6818,.T.);
#9073=ORIENTED_EDGE('',*,*,#6819,.T.);
#9074=ORIENTED_EDGE('',*,*,#6820,.T.);
#9075=ORIENTED_EDGE('',*,*,#6821,.T.);
#9076=ORIENTED_EDGE('',*,*,#6822,.T.);
#9077=ORIENTED_EDGE('',*,*,#6823,.F.);
#9078=ORIENTED_EDGE('',*,*,#6822,.F.);
#9079=ORIENTED_EDGE('',*,*,#6824,.T.);
#9080=ORIENTED_EDGE('',*,*,#6825,.T.);
#9081=ORIENTED_EDGE('',*,*,#6826,.T.);
#9082=ORIENTED_EDGE('',*,*,#6827,.T.);
#9083=ORIENTED_EDGE('',*,*,#6819,.F.);
#9084=ORIENTED_EDGE('',*,*,#6828,.T.);
#9085=ORIENTED_EDGE('',*,*,#6829,.T.);
#9086=ORIENTED_EDGE('',*,*,#6830,.T.);
#9087=ORIENTED_EDGE('',*,*,#6826,.F.);
#9088=ORIENTED_EDGE('',*,*,#6831,.T.);
#9089=ORIENTED_EDGE('',*,*,#6832,.T.);
#9090=ORIENTED_EDGE('',*,*,#6833,.T.);
#9091=ORIENTED_EDGE('',*,*,#6829,.F.);
#9092=ORIENTED_EDGE('',*,*,#6834,.T.);
#9093=ORIENTED_EDGE('',*,*,#6835,.T.);
#9094=ORIENTED_EDGE('',*,*,#6836,.T.);
#9095=ORIENTED_EDGE('',*,*,#6832,.F.);
#9096=ORIENTED_EDGE('',*,*,#6837,.T.);
#9097=ORIENTED_EDGE('',*,*,#6838,.T.);
#9098=ORIENTED_EDGE('',*,*,#6839,.T.);
#9099=ORIENTED_EDGE('',*,*,#6835,.F.);
#9100=ORIENTED_EDGE('',*,*,#6840,.T.);
#9101=ORIENTED_EDGE('',*,*,#6841,.T.);
#9102=ORIENTED_EDGE('',*,*,#6842,.T.);
#9103=ORIENTED_EDGE('',*,*,#6838,.F.);
#9104=ORIENTED_EDGE('',*,*,#6843,.T.);
#9105=ORIENTED_EDGE('',*,*,#6844,.T.);
#9106=ORIENTED_EDGE('',*,*,#6845,.T.);
#9107=ORIENTED_EDGE('',*,*,#6841,.F.);
#9108=ORIENTED_EDGE('',*,*,#6846,.T.);
#9109=ORIENTED_EDGE('',*,*,#6847,.F.);
#9110=ORIENTED_EDGE('',*,*,#6848,.T.);
#9111=ORIENTED_EDGE('',*,*,#6849,.F.);
#9112=ORIENTED_EDGE('',*,*,#6850,.T.);
#9113=ORIENTED_EDGE('',*,*,#6851,.T.);
#9114=ORIENTED_EDGE('',*,*,#6852,.T.);
#9115=ORIENTED_EDGE('',*,*,#6853,.F.);
#9116=ORIENTED_EDGE('',*,*,#6854,.F.);
#9117=ORIENTED_EDGE('',*,*,#6855,.T.);
#9118=ORIENTED_EDGE('',*,*,#6856,.T.);
#9119=ORIENTED_EDGE('',*,*,#6851,.F.);
#9120=ORIENTED_EDGE('',*,*,#6857,.F.);
#9121=ORIENTED_EDGE('',*,*,#6858,.T.);
#9122=ORIENTED_EDGE('',*,*,#6859,.T.);
#9123=ORIENTED_EDGE('',*,*,#6855,.F.);
#9124=ORIENTED_EDGE('',*,*,#6860,.F.);
#9125=ORIENTED_EDGE('',*,*,#6861,.T.);
#9126=ORIENTED_EDGE('',*,*,#6862,.T.);
#9127=ORIENTED_EDGE('',*,*,#6858,.F.);
#9128=ORIENTED_EDGE('',*,*,#6863,.F.);
#9129=ORIENTED_EDGE('',*,*,#6864,.T.);
#9130=ORIENTED_EDGE('',*,*,#6865,.T.);
#9131=ORIENTED_EDGE('',*,*,#6861,.F.);
#9132=ORIENTED_EDGE('',*,*,#6866,.F.);
#9133=ORIENTED_EDGE('',*,*,#6867,.T.);
#9134=ORIENTED_EDGE('',*,*,#6868,.T.);
#9135=ORIENTED_EDGE('',*,*,#6864,.F.);
#9136=ORIENTED_EDGE('',*,*,#6869,.F.);
#9137=ORIENTED_EDGE('',*,*,#6870,.T.);
#9138=ORIENTED_EDGE('',*,*,#6871,.T.);
#9139=ORIENTED_EDGE('',*,*,#6867,.F.);
#9140=ORIENTED_EDGE('',*,*,#6872,.F.);
#9141=ORIENTED_EDGE('',*,*,#6873,.T.);
#9142=ORIENTED_EDGE('',*,*,#6874,.T.);
#9143=ORIENTED_EDGE('',*,*,#6870,.F.);
#9144=ORIENTED_EDGE('',*,*,#6875,.F.);
#9145=ORIENTED_EDGE('',*,*,#6876,.F.);
#9146=ORIENTED_EDGE('',*,*,#6877,.F.);
#9147=ORIENTED_EDGE('',*,*,#6878,.F.);
#9148=ORIENTED_EDGE('',*,*,#6879,.T.);
#9149=ORIENTED_EDGE('',*,*,#6880,.T.);
#9150=ORIENTED_EDGE('',*,*,#6881,.T.);
#9151=ORIENTED_EDGE('',*,*,#6882,.T.);
#9152=ORIENTED_EDGE('',*,*,#6883,.T.);
#9153=ORIENTED_EDGE('',*,*,#6884,.F.);
#9154=ORIENTED_EDGE('',*,*,#6883,.F.);
#9155=ORIENTED_EDGE('',*,*,#6885,.T.);
#9156=ORIENTED_EDGE('',*,*,#6886,.T.);
#9157=ORIENTED_EDGE('',*,*,#6887,.T.);
#9158=ORIENTED_EDGE('',*,*,#6888,.T.);
#9159=ORIENTED_EDGE('',*,*,#6880,.F.);
#9160=ORIENTED_EDGE('',*,*,#6889,.T.);
#9161=ORIENTED_EDGE('',*,*,#6890,.T.);
#9162=ORIENTED_EDGE('',*,*,#6891,.T.);
#9163=ORIENTED_EDGE('',*,*,#6887,.F.);
#9164=ORIENTED_EDGE('',*,*,#6892,.T.);
#9165=ORIENTED_EDGE('',*,*,#6893,.T.);
#9166=ORIENTED_EDGE('',*,*,#6894,.T.);
#9167=ORIENTED_EDGE('',*,*,#6890,.F.);
#9168=ORIENTED_EDGE('',*,*,#6895,.T.);
#9169=ORIENTED_EDGE('',*,*,#6896,.T.);
#9170=ORIENTED_EDGE('',*,*,#6897,.T.);
#9171=ORIENTED_EDGE('',*,*,#6893,.F.);
#9172=ORIENTED_EDGE('',*,*,#6898,.T.);
#9173=ORIENTED_EDGE('',*,*,#6899,.T.);
#9174=ORIENTED_EDGE('',*,*,#6900,.T.);
#9175=ORIENTED_EDGE('',*,*,#6896,.F.);
#9176=ORIENTED_EDGE('',*,*,#6901,.T.);
#9177=ORIENTED_EDGE('',*,*,#6902,.T.);
#9178=ORIENTED_EDGE('',*,*,#6903,.T.);
#9179=ORIENTED_EDGE('',*,*,#6899,.F.);
#9180=ORIENTED_EDGE('',*,*,#6904,.T.);
#9181=ORIENTED_EDGE('',*,*,#6905,.T.);
#9182=ORIENTED_EDGE('',*,*,#6906,.T.);
#9183=ORIENTED_EDGE('',*,*,#6902,.F.);
#9184=ORIENTED_EDGE('',*,*,#6907,.T.);
#9185=ORIENTED_EDGE('',*,*,#6908,.F.);
#9186=ORIENTED_EDGE('',*,*,#6909,.T.);
#9187=ORIENTED_EDGE('',*,*,#6910,.F.);
#9188=ORIENTED_EDGE('',*,*,#6911,.T.);
#9189=ORIENTED_EDGE('',*,*,#6912,.T.);
#9190=ORIENTED_EDGE('',*,*,#6913,.T.);
#9191=ORIENTED_EDGE('',*,*,#6914,.F.);
#9192=ORIENTED_EDGE('',*,*,#6915,.F.);
#9193=ORIENTED_EDGE('',*,*,#6916,.T.);
#9194=ORIENTED_EDGE('',*,*,#6917,.T.);
#9195=ORIENTED_EDGE('',*,*,#6912,.F.);
#9196=ORIENTED_EDGE('',*,*,#6918,.F.);
#9197=ORIENTED_EDGE('',*,*,#6919,.T.);
#9198=ORIENTED_EDGE('',*,*,#6920,.T.);
#9199=ORIENTED_EDGE('',*,*,#6916,.F.);
#9200=ORIENTED_EDGE('',*,*,#6921,.F.);
#9201=ORIENTED_EDGE('',*,*,#6922,.T.);
#9202=ORIENTED_EDGE('',*,*,#6923,.T.);
#9203=ORIENTED_EDGE('',*,*,#6919,.F.);
#9204=ORIENTED_EDGE('',*,*,#6924,.F.);
#9205=ORIENTED_EDGE('',*,*,#6925,.T.);
#9206=ORIENTED_EDGE('',*,*,#6926,.T.);
#9207=ORIENTED_EDGE('',*,*,#6922,.F.);
#9208=ORIENTED_EDGE('',*,*,#6927,.F.);
#9209=ORIENTED_EDGE('',*,*,#6928,.T.);
#9210=ORIENTED_EDGE('',*,*,#6929,.T.);
#9211=ORIENTED_EDGE('',*,*,#6925,.F.);
#9212=ORIENTED_EDGE('',*,*,#6930,.F.);
#9213=ORIENTED_EDGE('',*,*,#6931,.T.);
#9214=ORIENTED_EDGE('',*,*,#6932,.T.);
#9215=ORIENTED_EDGE('',*,*,#6928,.F.);
#9216=ORIENTED_EDGE('',*,*,#6933,.F.);
#9217=ORIENTED_EDGE('',*,*,#6934,.T.);
#9218=ORIENTED_EDGE('',*,*,#6935,.T.);
#9219=ORIENTED_EDGE('',*,*,#6931,.F.);
#9220=ORIENTED_EDGE('',*,*,#6936,.F.);
#9221=ORIENTED_EDGE('',*,*,#6937,.F.);
#9222=ORIENTED_EDGE('',*,*,#6938,.F.);
#9223=ORIENTED_EDGE('',*,*,#6939,.F.);
#9224=ORIENTED_EDGE('',*,*,#6940,.T.);
#9225=ORIENTED_EDGE('',*,*,#6941,.T.);
#9226=ORIENTED_EDGE('',*,*,#6942,.T.);
#9227=ORIENTED_EDGE('',*,*,#6943,.T.);
#9228=ORIENTED_EDGE('',*,*,#6944,.T.);
#9229=ORIENTED_EDGE('',*,*,#6945,.F.);
#9230=ORIENTED_EDGE('',*,*,#6944,.F.);
#9231=ORIENTED_EDGE('',*,*,#6946,.T.);
#9232=ORIENTED_EDGE('',*,*,#6947,.T.);
#9233=ORIENTED_EDGE('',*,*,#6948,.T.);
#9234=ORIENTED_EDGE('',*,*,#6949,.T.);
#9235=ORIENTED_EDGE('',*,*,#6941,.F.);
#9236=ORIENTED_EDGE('',*,*,#6950,.T.);
#9237=ORIENTED_EDGE('',*,*,#6951,.T.);
#9238=ORIENTED_EDGE('',*,*,#6952,.T.);
#9239=ORIENTED_EDGE('',*,*,#6948,.F.);
#9240=ORIENTED_EDGE('',*,*,#6953,.T.);
#9241=ORIENTED_EDGE('',*,*,#6954,.T.);
#9242=ORIENTED_EDGE('',*,*,#6955,.T.);
#9243=ORIENTED_EDGE('',*,*,#6951,.F.);
#9244=ORIENTED_EDGE('',*,*,#6956,.T.);
#9245=ORIENTED_EDGE('',*,*,#6957,.T.);
#9246=ORIENTED_EDGE('',*,*,#6958,.T.);
#9247=ORIENTED_EDGE('',*,*,#6954,.F.);
#9248=ORIENTED_EDGE('',*,*,#6959,.T.);
#9249=ORIENTED_EDGE('',*,*,#6960,.T.);
#9250=ORIENTED_EDGE('',*,*,#6961,.T.);
#9251=ORIENTED_EDGE('',*,*,#6957,.F.);
#9252=ORIENTED_EDGE('',*,*,#6962,.T.);
#9253=ORIENTED_EDGE('',*,*,#6963,.T.);
#9254=ORIENTED_EDGE('',*,*,#6964,.T.);
#9255=ORIENTED_EDGE('',*,*,#6960,.F.);
#9256=ORIENTED_EDGE('',*,*,#6965,.T.);
#9257=ORIENTED_EDGE('',*,*,#6966,.T.);
#9258=ORIENTED_EDGE('',*,*,#6967,.T.);
#9259=ORIENTED_EDGE('',*,*,#6963,.F.);
#9260=ORIENTED_EDGE('',*,*,#6968,.T.);
#9261=ORIENTED_EDGE('',*,*,#6969,.F.);
#9262=ORIENTED_EDGE('',*,*,#6970,.T.);
#9263=ORIENTED_EDGE('',*,*,#6971,.F.);
#9264=ORIENTED_EDGE('',*,*,#6972,.T.);
#9265=ORIENTED_EDGE('',*,*,#6973,.T.);
#9266=ORIENTED_EDGE('',*,*,#6974,.T.);
#9267=ORIENTED_EDGE('',*,*,#6975,.F.);
#9268=ORIENTED_EDGE('',*,*,#6976,.F.);
#9269=ORIENTED_EDGE('',*,*,#6977,.T.);
#9270=ORIENTED_EDGE('',*,*,#6978,.T.);
#9271=ORIENTED_EDGE('',*,*,#6973,.F.);
#9272=ORIENTED_EDGE('',*,*,#6979,.F.);
#9273=ORIENTED_EDGE('',*,*,#6980,.T.);
#9274=ORIENTED_EDGE('',*,*,#6981,.T.);
#9275=ORIENTED_EDGE('',*,*,#6977,.F.);
#9276=ORIENTED_EDGE('',*,*,#6982,.F.);
#9277=ORIENTED_EDGE('',*,*,#6983,.T.);
#9278=ORIENTED_EDGE('',*,*,#6984,.T.);
#9279=ORIENTED_EDGE('',*,*,#6980,.F.);
#9280=ORIENTED_EDGE('',*,*,#6985,.F.);
#9281=ORIENTED_EDGE('',*,*,#6986,.T.);
#9282=ORIENTED_EDGE('',*,*,#6987,.T.);
#9283=ORIENTED_EDGE('',*,*,#6983,.F.);
#9284=ORIENTED_EDGE('',*,*,#6988,.F.);
#9285=ORIENTED_EDGE('',*,*,#6989,.T.);
#9286=ORIENTED_EDGE('',*,*,#6990,.T.);
#9287=ORIENTED_EDGE('',*,*,#6986,.F.);
#9288=ORIENTED_EDGE('',*,*,#6991,.F.);
#9289=ORIENTED_EDGE('',*,*,#6992,.T.);
#9290=ORIENTED_EDGE('',*,*,#6993,.T.);
#9291=ORIENTED_EDGE('',*,*,#6989,.F.);
#9292=ORIENTED_EDGE('',*,*,#6994,.F.);
#9293=ORIENTED_EDGE('',*,*,#6995,.T.);
#9294=ORIENTED_EDGE('',*,*,#6996,.T.);
#9295=ORIENTED_EDGE('',*,*,#6992,.F.);
#9296=ORIENTED_EDGE('',*,*,#6997,.F.);
#9297=ORIENTED_EDGE('',*,*,#6998,.F.);
#9298=ORIENTED_EDGE('',*,*,#6999,.F.);
#9299=ORIENTED_EDGE('',*,*,#7000,.F.);
#9300=ORIENTED_EDGE('',*,*,#7001,.T.);
#9301=ORIENTED_EDGE('',*,*,#7002,.T.);
#9302=ORIENTED_EDGE('',*,*,#7003,.T.);
#9303=ORIENTED_EDGE('',*,*,#7004,.T.);
#9304=ORIENTED_EDGE('',*,*,#7005,.T.);
#9305=ORIENTED_EDGE('',*,*,#7006,.F.);
#9306=ORIENTED_EDGE('',*,*,#7005,.F.);
#9307=ORIENTED_EDGE('',*,*,#7007,.T.);
#9308=ORIENTED_EDGE('',*,*,#7008,.T.);
#9309=ORIENTED_EDGE('',*,*,#7009,.T.);
#9310=ORIENTED_EDGE('',*,*,#7010,.T.);
#9311=ORIENTED_EDGE('',*,*,#7002,.F.);
#9312=ORIENTED_EDGE('',*,*,#7011,.T.);
#9313=ORIENTED_EDGE('',*,*,#7012,.T.);
#9314=ORIENTED_EDGE('',*,*,#7013,.T.);
#9315=ORIENTED_EDGE('',*,*,#7009,.F.);
#9316=ORIENTED_EDGE('',*,*,#7014,.T.);
#9317=ORIENTED_EDGE('',*,*,#7015,.T.);
#9318=ORIENTED_EDGE('',*,*,#7016,.T.);
#9319=ORIENTED_EDGE('',*,*,#7012,.F.);
#9320=ORIENTED_EDGE('',*,*,#7017,.T.);
#9321=ORIENTED_EDGE('',*,*,#7018,.T.);
#9322=ORIENTED_EDGE('',*,*,#7019,.T.);
#9323=ORIENTED_EDGE('',*,*,#7015,.F.);
#9324=ORIENTED_EDGE('',*,*,#7020,.T.);
#9325=ORIENTED_EDGE('',*,*,#7021,.T.);
#9326=ORIENTED_EDGE('',*,*,#7022,.T.);
#9327=ORIENTED_EDGE('',*,*,#7018,.F.);
#9328=ORIENTED_EDGE('',*,*,#7023,.T.);
#9329=ORIENTED_EDGE('',*,*,#7024,.T.);
#9330=ORIENTED_EDGE('',*,*,#7025,.T.);
#9331=ORIENTED_EDGE('',*,*,#7021,.F.);
#9332=ORIENTED_EDGE('',*,*,#7026,.T.);
#9333=ORIENTED_EDGE('',*,*,#7027,.T.);
#9334=ORIENTED_EDGE('',*,*,#7028,.T.);
#9335=ORIENTED_EDGE('',*,*,#7024,.F.);
#9336=ORIENTED_EDGE('',*,*,#7029,.T.);
#9337=ORIENTED_EDGE('',*,*,#7030,.F.);
#9338=ORIENTED_EDGE('',*,*,#7031,.T.);
#9339=ORIENTED_EDGE('',*,*,#7032,.F.);
#9340=ORIENTED_EDGE('',*,*,#7033,.T.);
#9341=ORIENTED_EDGE('',*,*,#7034,.T.);
#9342=ORIENTED_EDGE('',*,*,#7035,.T.);
#9343=ORIENTED_EDGE('',*,*,#7036,.F.);
#9344=ORIENTED_EDGE('',*,*,#7037,.F.);
#9345=ORIENTED_EDGE('',*,*,#7038,.T.);
#9346=ORIENTED_EDGE('',*,*,#7039,.T.);
#9347=ORIENTED_EDGE('',*,*,#7034,.F.);
#9348=ORIENTED_EDGE('',*,*,#7040,.F.);
#9349=ORIENTED_EDGE('',*,*,#7041,.T.);
#9350=ORIENTED_EDGE('',*,*,#7042,.T.);
#9351=ORIENTED_EDGE('',*,*,#7038,.F.);
#9352=ORIENTED_EDGE('',*,*,#7043,.F.);
#9353=ORIENTED_EDGE('',*,*,#7044,.T.);
#9354=ORIENTED_EDGE('',*,*,#7045,.T.);
#9355=ORIENTED_EDGE('',*,*,#7041,.F.);
#9356=ORIENTED_EDGE('',*,*,#7046,.F.);
#9357=ORIENTED_EDGE('',*,*,#7047,.T.);
#9358=ORIENTED_EDGE('',*,*,#7048,.T.);
#9359=ORIENTED_EDGE('',*,*,#7044,.F.);
#9360=ORIENTED_EDGE('',*,*,#7049,.F.);
#9361=ORIENTED_EDGE('',*,*,#7050,.T.);
#9362=ORIENTED_EDGE('',*,*,#7051,.T.);
#9363=ORIENTED_EDGE('',*,*,#7047,.F.);
#9364=ORIENTED_EDGE('',*,*,#7052,.F.);
#9365=ORIENTED_EDGE('',*,*,#7053,.T.);
#9366=ORIENTED_EDGE('',*,*,#7054,.T.);
#9367=ORIENTED_EDGE('',*,*,#7050,.F.);
#9368=ORIENTED_EDGE('',*,*,#7055,.F.);
#9369=ORIENTED_EDGE('',*,*,#7056,.T.);
#9370=ORIENTED_EDGE('',*,*,#7057,.T.);
#9371=ORIENTED_EDGE('',*,*,#7053,.F.);
#9372=ORIENTED_EDGE('',*,*,#7058,.F.);
#9373=ORIENTED_EDGE('',*,*,#7059,.F.);
#9374=ORIENTED_EDGE('',*,*,#7060,.F.);
#9375=ORIENTED_EDGE('',*,*,#7061,.F.);
#9376=ORIENTED_EDGE('',*,*,#7062,.T.);
#9377=ORIENTED_EDGE('',*,*,#7063,.T.);
#9378=ORIENTED_EDGE('',*,*,#7064,.T.);
#9379=ORIENTED_EDGE('',*,*,#7065,.T.);
#9380=ORIENTED_EDGE('',*,*,#7066,.T.);
#9381=ORIENTED_EDGE('',*,*,#7067,.F.);
#9382=ORIENTED_EDGE('',*,*,#7066,.F.);
#9383=ORIENTED_EDGE('',*,*,#7068,.T.);
#9384=ORIENTED_EDGE('',*,*,#7069,.T.);
#9385=ORIENTED_EDGE('',*,*,#7070,.T.);
#9386=ORIENTED_EDGE('',*,*,#7071,.T.);
#9387=ORIENTED_EDGE('',*,*,#7063,.F.);
#9388=ORIENTED_EDGE('',*,*,#7072,.T.);
#9389=ORIENTED_EDGE('',*,*,#7073,.T.);
#9390=ORIENTED_EDGE('',*,*,#7074,.T.);
#9391=ORIENTED_EDGE('',*,*,#7070,.F.);
#9392=ORIENTED_EDGE('',*,*,#7075,.T.);
#9393=ORIENTED_EDGE('',*,*,#7076,.T.);
#9394=ORIENTED_EDGE('',*,*,#7077,.T.);
#9395=ORIENTED_EDGE('',*,*,#7073,.F.);
#9396=ORIENTED_EDGE('',*,*,#7078,.T.);
#9397=ORIENTED_EDGE('',*,*,#7079,.T.);
#9398=ORIENTED_EDGE('',*,*,#7080,.T.);
#9399=ORIENTED_EDGE('',*,*,#7076,.F.);
#9400=ORIENTED_EDGE('',*,*,#7081,.T.);
#9401=ORIENTED_EDGE('',*,*,#7082,.T.);
#9402=ORIENTED_EDGE('',*,*,#7083,.T.);
#9403=ORIENTED_EDGE('',*,*,#7079,.F.);
#9404=ORIENTED_EDGE('',*,*,#7084,.T.);
#9405=ORIENTED_EDGE('',*,*,#7085,.T.);
#9406=ORIENTED_EDGE('',*,*,#7086,.T.);
#9407=ORIENTED_EDGE('',*,*,#7082,.F.);
#9408=ORIENTED_EDGE('',*,*,#7087,.T.);
#9409=ORIENTED_EDGE('',*,*,#7088,.T.);
#9410=ORIENTED_EDGE('',*,*,#7089,.T.);
#9411=ORIENTED_EDGE('',*,*,#7085,.F.);
#9412=ORIENTED_EDGE('',*,*,#7090,.T.);
#9413=ORIENTED_EDGE('',*,*,#7091,.F.);
#9414=ORIENTED_EDGE('',*,*,#7092,.T.);
#9415=ORIENTED_EDGE('',*,*,#7093,.F.);
#9416=ORIENTED_EDGE('',*,*,#7094,.T.);
#9417=ORIENTED_EDGE('',*,*,#7095,.T.);
#9418=ORIENTED_EDGE('',*,*,#7096,.T.);
#9419=ORIENTED_EDGE('',*,*,#7097,.F.);
#9420=ORIENTED_EDGE('',*,*,#7098,.F.);
#9421=ORIENTED_EDGE('',*,*,#7099,.T.);
#9422=ORIENTED_EDGE('',*,*,#7100,.T.);
#9423=ORIENTED_EDGE('',*,*,#7095,.F.);
#9424=ORIENTED_EDGE('',*,*,#7101,.F.);
#9425=ORIENTED_EDGE('',*,*,#7102,.T.);
#9426=ORIENTED_EDGE('',*,*,#7103,.T.);
#9427=ORIENTED_EDGE('',*,*,#7099,.F.);
#9428=ORIENTED_EDGE('',*,*,#7104,.F.);
#9429=ORIENTED_EDGE('',*,*,#7105,.T.);
#9430=ORIENTED_EDGE('',*,*,#7106,.T.);
#9431=ORIENTED_EDGE('',*,*,#7102,.F.);
#9432=ORIENTED_EDGE('',*,*,#7107,.F.);
#9433=ORIENTED_EDGE('',*,*,#7108,.T.);
#9434=ORIENTED_EDGE('',*,*,#7109,.T.);
#9435=ORIENTED_EDGE('',*,*,#7105,.F.);
#9436=ORIENTED_EDGE('',*,*,#7110,.F.);
#9437=ORIENTED_EDGE('',*,*,#7111,.T.);
#9438=ORIENTED_EDGE('',*,*,#7112,.T.);
#9439=ORIENTED_EDGE('',*,*,#7108,.F.);
#9440=ORIENTED_EDGE('',*,*,#7113,.F.);
#9441=ORIENTED_EDGE('',*,*,#7114,.T.);
#9442=ORIENTED_EDGE('',*,*,#7115,.T.);
#9443=ORIENTED_EDGE('',*,*,#7111,.F.);
#9444=ORIENTED_EDGE('',*,*,#7116,.F.);
#9445=ORIENTED_EDGE('',*,*,#7117,.T.);
#9446=ORIENTED_EDGE('',*,*,#7118,.T.);
#9447=ORIENTED_EDGE('',*,*,#7114,.F.);
#9448=ORIENTED_EDGE('',*,*,#7119,.F.);
#9449=ORIENTED_EDGE('',*,*,#7120,.F.);
#9450=ORIENTED_EDGE('',*,*,#7121,.F.);
#9451=ORIENTED_EDGE('',*,*,#7122,.F.);
#9452=ORIENTED_EDGE('',*,*,#7123,.T.);
#9453=ORIENTED_EDGE('',*,*,#7124,.T.);
#9454=ORIENTED_EDGE('',*,*,#7125,.T.);
#9455=ORIENTED_EDGE('',*,*,#7126,.T.);
#9456=ORIENTED_EDGE('',*,*,#7127,.T.);
#9457=ORIENTED_EDGE('',*,*,#7128,.F.);
#9458=ORIENTED_EDGE('',*,*,#7127,.F.);
#9459=ORIENTED_EDGE('',*,*,#7129,.T.);
#9460=ORIENTED_EDGE('',*,*,#7130,.T.);
#9461=ORIENTED_EDGE('',*,*,#7131,.T.);
#9462=ORIENTED_EDGE('',*,*,#7132,.T.);
#9463=ORIENTED_EDGE('',*,*,#7124,.F.);
#9464=ORIENTED_EDGE('',*,*,#7133,.T.);
#9465=ORIENTED_EDGE('',*,*,#7134,.T.);
#9466=ORIENTED_EDGE('',*,*,#7135,.T.);
#9467=ORIENTED_EDGE('',*,*,#7131,.F.);
#9468=ORIENTED_EDGE('',*,*,#7136,.T.);
#9469=ORIENTED_EDGE('',*,*,#7137,.T.);
#9470=ORIENTED_EDGE('',*,*,#7138,.T.);
#9471=ORIENTED_EDGE('',*,*,#7134,.F.);
#9472=ORIENTED_EDGE('',*,*,#7139,.T.);
#9473=ORIENTED_EDGE('',*,*,#7140,.T.);
#9474=ORIENTED_EDGE('',*,*,#7141,.T.);
#9475=ORIENTED_EDGE('',*,*,#7137,.F.);
#9476=ORIENTED_EDGE('',*,*,#7142,.T.);
#9477=ORIENTED_EDGE('',*,*,#7143,.T.);
#9478=ORIENTED_EDGE('',*,*,#7144,.T.);
#9479=ORIENTED_EDGE('',*,*,#7140,.F.);
#9480=ORIENTED_EDGE('',*,*,#7145,.T.);
#9481=ORIENTED_EDGE('',*,*,#7146,.T.);
#9482=ORIENTED_EDGE('',*,*,#7147,.T.);
#9483=ORIENTED_EDGE('',*,*,#7143,.F.);
#9484=ORIENTED_EDGE('',*,*,#7148,.T.);
#9485=ORIENTED_EDGE('',*,*,#7149,.T.);
#9486=ORIENTED_EDGE('',*,*,#7150,.T.);
#9487=ORIENTED_EDGE('',*,*,#7146,.F.);
#9488=ORIENTED_EDGE('',*,*,#7151,.T.);
#9489=ORIENTED_EDGE('',*,*,#7152,.F.);
#9490=ORIENTED_EDGE('',*,*,#7153,.T.);
#9491=ORIENTED_EDGE('',*,*,#7154,.F.);
#9492=ORIENTED_EDGE('',*,*,#7155,.T.);
#9493=ORIENTED_EDGE('',*,*,#7156,.T.);
#9494=ORIENTED_EDGE('',*,*,#7157,.T.);
#9495=ORIENTED_EDGE('',*,*,#7158,.F.);
#9496=ORIENTED_EDGE('',*,*,#7159,.F.);
#9497=ORIENTED_EDGE('',*,*,#7160,.T.);
#9498=ORIENTED_EDGE('',*,*,#7161,.T.);
#9499=ORIENTED_EDGE('',*,*,#7156,.F.);
#9500=ORIENTED_EDGE('',*,*,#7162,.F.);
#9501=ORIENTED_EDGE('',*,*,#7163,.T.);
#9502=ORIENTED_EDGE('',*,*,#7164,.T.);
#9503=ORIENTED_EDGE('',*,*,#7160,.F.);
#9504=ORIENTED_EDGE('',*,*,#7165,.F.);
#9505=ORIENTED_EDGE('',*,*,#7166,.T.);
#9506=ORIENTED_EDGE('',*,*,#7167,.T.);
#9507=ORIENTED_EDGE('',*,*,#7163,.F.);
#9508=ORIENTED_EDGE('',*,*,#7168,.F.);
#9509=ORIENTED_EDGE('',*,*,#7169,.T.);
#9510=ORIENTED_EDGE('',*,*,#7170,.T.);
#9511=ORIENTED_EDGE('',*,*,#7166,.F.);
#9512=ORIENTED_EDGE('',*,*,#7171,.F.);
#9513=ORIENTED_EDGE('',*,*,#7172,.T.);
#9514=ORIENTED_EDGE('',*,*,#7173,.T.);
#9515=ORIENTED_EDGE('',*,*,#7169,.F.);
#9516=ORIENTED_EDGE('',*,*,#7174,.F.);
#9517=ORIENTED_EDGE('',*,*,#7175,.T.);
#9518=ORIENTED_EDGE('',*,*,#7176,.T.);
#9519=ORIENTED_EDGE('',*,*,#7172,.F.);
#9520=ORIENTED_EDGE('',*,*,#7177,.F.);
#9521=ORIENTED_EDGE('',*,*,#7178,.T.);
#9522=ORIENTED_EDGE('',*,*,#7179,.T.);
#9523=ORIENTED_EDGE('',*,*,#7175,.F.);
#9524=ORIENTED_EDGE('',*,*,#7180,.F.);
#9525=ORIENTED_EDGE('',*,*,#7181,.F.);
#9526=ORIENTED_EDGE('',*,*,#7182,.F.);
#9527=ORIENTED_EDGE('',*,*,#7183,.F.);
#9528=ORIENTED_EDGE('',*,*,#7184,.T.);
#9529=ORIENTED_EDGE('',*,*,#7185,.F.);
#9530=ORIENTED_EDGE('',*,*,#7186,.T.);
#9531=ORIENTED_EDGE('',*,*,#7187,.T.);
#9532=ORIENTED_EDGE('',*,*,#7186,.F.);
#9533=ORIENTED_EDGE('',*,*,#7187,.F.);
#9534=ORIENTED_EDGE('',*,*,#7188,.F.);
#9535=ORIENTED_EDGE('',*,*,#7189,.F.);
#9536=ORIENTED_EDGE('',*,*,#7190,.T.);
#9537=ORIENTED_EDGE('',*,*,#7191,.T.);
#9538=ORIENTED_EDGE('',*,*,#7190,.F.);
#9539=ORIENTED_EDGE('',*,*,#7191,.F.);
#9540=ORIENTED_EDGE('',*,*,#7192,.F.);
#9541=ORIENTED_EDGE('',*,*,#7193,.F.);
#9542=ORIENTED_EDGE('',*,*,#7194,.T.);
#9543=ORIENTED_EDGE('',*,*,#7195,.T.);
#9544=ORIENTED_EDGE('',*,*,#7194,.F.);
#9545=ORIENTED_EDGE('',*,*,#7195,.F.);
#9546=ORIENTED_EDGE('',*,*,#7196,.F.);
#9547=ORIENTED_EDGE('',*,*,#7197,.F.);
#9548=ORIENTED_EDGE('',*,*,#7198,.T.);
#9549=ORIENTED_EDGE('',*,*,#7199,.T.);
#9550=ORIENTED_EDGE('',*,*,#7198,.F.);
#9551=ORIENTED_EDGE('',*,*,#7199,.F.);
#9552=ORIENTED_EDGE('',*,*,#7200,.F.);
#9553=ORIENTED_EDGE('',*,*,#7188,.T.);
#9554=ORIENTED_EDGE('',*,*,#7201,.T.);
#9555=ORIENTED_EDGE('',*,*,#7202,.F.);
#9556=ORIENTED_EDGE('',*,*,#7201,.F.);
#9557=ORIENTED_EDGE('',*,*,#7192,.T.);
#9558=ORIENTED_EDGE('',*,*,#7203,.T.);
#9559=ORIENTED_EDGE('',*,*,#7204,.F.);
#9560=ORIENTED_EDGE('',*,*,#7203,.F.);
#9561=ORIENTED_EDGE('',*,*,#7196,.T.);
#9562=ORIENTED_EDGE('',*,*,#7205,.T.);
#9563=ORIENTED_EDGE('',*,*,#7206,.F.);
#9564=ORIENTED_EDGE('',*,*,#7205,.F.);
#9565=ORIENTED_EDGE('',*,*,#7200,.T.);
#9566=ORIENTED_EDGE('',*,*,#7207,.T.);
#9567=ORIENTED_EDGE('',*,*,#7208,.F.);
#9568=ORIENTED_EDGE('',*,*,#7207,.F.);
#9569=ORIENTED_EDGE('',*,*,#7126,.F.);
#9570=ORIENTED_EDGE('',*,*,#7209,.T.);
#9571=ORIENTED_EDGE('',*,*,#7158,.T.);
#9572=ORIENTED_EDGE('',*,*,#7210,.T.);
#9573=ORIENTED_EDGE('',*,*,#7129,.F.);
#9574=ORIENTED_EDGE('',*,*,#7181,.T.);
#9575=ORIENTED_EDGE('',*,*,#7211,.T.);
#9576=ORIENTED_EDGE('',*,*,#7178,.F.);
#9577=ORIENTED_EDGE('',*,*,#7212,.F.);
#9578=ORIENTED_EDGE('',*,*,#7210,.F.);
#9579=ORIENTED_EDGE('',*,*,#7157,.F.);
#9580=ORIENTED_EDGE('',*,*,#7161,.F.);
#9581=ORIENTED_EDGE('',*,*,#7164,.F.);
#9582=ORIENTED_EDGE('',*,*,#7167,.F.);
#9583=ORIENTED_EDGE('',*,*,#7170,.F.);
#9584=ORIENTED_EDGE('',*,*,#7173,.F.);
#9585=ORIENTED_EDGE('',*,*,#7176,.F.);
#9586=ORIENTED_EDGE('',*,*,#7179,.F.);
#9587=ORIENTED_EDGE('',*,*,#7211,.F.);
#9588=ORIENTED_EDGE('',*,*,#7184,.F.);
#9589=ORIENTED_EDGE('',*,*,#7213,.F.);
#9590=ORIENTED_EDGE('',*,*,#7153,.F.);
#9591=ORIENTED_EDGE('',*,*,#7214,.F.);
#9592=ORIENTED_EDGE('',*,*,#7151,.F.);
#9593=ORIENTED_EDGE('',*,*,#7148,.F.);
#9594=ORIENTED_EDGE('',*,*,#7145,.F.);
#9595=ORIENTED_EDGE('',*,*,#7142,.F.);
#9596=ORIENTED_EDGE('',*,*,#7139,.F.);
#9597=ORIENTED_EDGE('',*,*,#7136,.F.);
#9598=ORIENTED_EDGE('',*,*,#7133,.F.);
#9599=ORIENTED_EDGE('',*,*,#7130,.F.);
#9600=ORIENTED_EDGE('',*,*,#7209,.F.);
#9601=ORIENTED_EDGE('',*,*,#7125,.F.);
#9602=ORIENTED_EDGE('',*,*,#7132,.F.);
#9603=ORIENTED_EDGE('',*,*,#7135,.F.);
#9604=ORIENTED_EDGE('',*,*,#7138,.F.);
#9605=ORIENTED_EDGE('',*,*,#7141,.F.);
#9606=ORIENTED_EDGE('',*,*,#7144,.F.);
#9607=ORIENTED_EDGE('',*,*,#7147,.F.);
#9608=ORIENTED_EDGE('',*,*,#7150,.F.);
#9609=ORIENTED_EDGE('',*,*,#7215,.F.);
#9610=ORIENTED_EDGE('',*,*,#7155,.F.);
#9611=ORIENTED_EDGE('',*,*,#7216,.F.);
#9612=ORIENTED_EDGE('',*,*,#7182,.T.);
#9613=ORIENTED_EDGE('',*,*,#7212,.T.);
#9614=ORIENTED_EDGE('',*,*,#7180,.T.);
#9615=ORIENTED_EDGE('',*,*,#7177,.T.);
#9616=ORIENTED_EDGE('',*,*,#7174,.T.);
#9617=ORIENTED_EDGE('',*,*,#7171,.T.);
#9618=ORIENTED_EDGE('',*,*,#7168,.T.);
#9619=ORIENTED_EDGE('',*,*,#7165,.T.);
#9620=ORIENTED_EDGE('',*,*,#7162,.T.);
#9621=ORIENTED_EDGE('',*,*,#7159,.T.);
#9622=ORIENTED_EDGE('',*,*,#7152,.T.);
#9623=ORIENTED_EDGE('',*,*,#7215,.T.);
#9624=ORIENTED_EDGE('',*,*,#7149,.F.);
#9625=ORIENTED_EDGE('',*,*,#7214,.T.);
#9626=ORIENTED_EDGE('',*,*,#7065,.F.);
#9627=ORIENTED_EDGE('',*,*,#7217,.T.);
#9628=ORIENTED_EDGE('',*,*,#7097,.T.);
#9629=ORIENTED_EDGE('',*,*,#7218,.T.);
#9630=ORIENTED_EDGE('',*,*,#7068,.F.);
#9631=ORIENTED_EDGE('',*,*,#7120,.T.);
#9632=ORIENTED_EDGE('',*,*,#7219,.T.);
#9633=ORIENTED_EDGE('',*,*,#7117,.F.);
#9634=ORIENTED_EDGE('',*,*,#7220,.F.);
#9635=ORIENTED_EDGE('',*,*,#7218,.F.);
#9636=ORIENTED_EDGE('',*,*,#7096,.F.);
#9637=ORIENTED_EDGE('',*,*,#7100,.F.);
#9638=ORIENTED_EDGE('',*,*,#7103,.F.);
#9639=ORIENTED_EDGE('',*,*,#7106,.F.);
#9640=ORIENTED_EDGE('',*,*,#7109,.F.);
#9641=ORIENTED_EDGE('',*,*,#7112,.F.);
#9642=ORIENTED_EDGE('',*,*,#7115,.F.);
#9643=ORIENTED_EDGE('',*,*,#7118,.F.);
#9644=ORIENTED_EDGE('',*,*,#7219,.F.);
#9645=ORIENTED_EDGE('',*,*,#7123,.F.);
#9646=ORIENTED_EDGE('',*,*,#7221,.F.);
#9647=ORIENTED_EDGE('',*,*,#7092,.F.);
#9648=ORIENTED_EDGE('',*,*,#7222,.F.);
#9649=ORIENTED_EDGE('',*,*,#7090,.F.);
#9650=ORIENTED_EDGE('',*,*,#7087,.F.);
#9651=ORIENTED_EDGE('',*,*,#7084,.F.);
#9652=ORIENTED_EDGE('',*,*,#7081,.F.);
#9653=ORIENTED_EDGE('',*,*,#7078,.F.);
#9654=ORIENTED_EDGE('',*,*,#7075,.F.);
#9655=ORIENTED_EDGE('',*,*,#7072,.F.);
#9656=ORIENTED_EDGE('',*,*,#7069,.F.);
#9657=ORIENTED_EDGE('',*,*,#7217,.F.);
#9658=ORIENTED_EDGE('',*,*,#7064,.F.);
#9659=ORIENTED_EDGE('',*,*,#7071,.F.);
#9660=ORIENTED_EDGE('',*,*,#7074,.F.);
#9661=ORIENTED_EDGE('',*,*,#7077,.F.);
#9662=ORIENTED_EDGE('',*,*,#7080,.F.);
#9663=ORIENTED_EDGE('',*,*,#7083,.F.);
#9664=ORIENTED_EDGE('',*,*,#7086,.F.);
#9665=ORIENTED_EDGE('',*,*,#7089,.F.);
#9666=ORIENTED_EDGE('',*,*,#7223,.F.);
#9667=ORIENTED_EDGE('',*,*,#7094,.F.);
#9668=ORIENTED_EDGE('',*,*,#7224,.F.);
#9669=ORIENTED_EDGE('',*,*,#7121,.T.);
#9670=ORIENTED_EDGE('',*,*,#7220,.T.);
#9671=ORIENTED_EDGE('',*,*,#7119,.T.);
#9672=ORIENTED_EDGE('',*,*,#7116,.T.);
#9673=ORIENTED_EDGE('',*,*,#7113,.T.);
#9674=ORIENTED_EDGE('',*,*,#7110,.T.);
#9675=ORIENTED_EDGE('',*,*,#7107,.T.);
#9676=ORIENTED_EDGE('',*,*,#7104,.T.);
#9677=ORIENTED_EDGE('',*,*,#7101,.T.);
#9678=ORIENTED_EDGE('',*,*,#7098,.T.);
#9679=ORIENTED_EDGE('',*,*,#7091,.T.);
#9680=ORIENTED_EDGE('',*,*,#7223,.T.);
#9681=ORIENTED_EDGE('',*,*,#7088,.F.);
#9682=ORIENTED_EDGE('',*,*,#7222,.T.);
#9683=ORIENTED_EDGE('',*,*,#7004,.F.);
#9684=ORIENTED_EDGE('',*,*,#7225,.T.);
#9685=ORIENTED_EDGE('',*,*,#7036,.T.);
#9686=ORIENTED_EDGE('',*,*,#7226,.T.);
#9687=ORIENTED_EDGE('',*,*,#7007,.F.);
#9688=ORIENTED_EDGE('',*,*,#7059,.T.);
#9689=ORIENTED_EDGE('',*,*,#7227,.T.);
#9690=ORIENTED_EDGE('',*,*,#7056,.F.);
#9691=ORIENTED_EDGE('',*,*,#7228,.F.);
#9692=ORIENTED_EDGE('',*,*,#7226,.F.);
#9693=ORIENTED_EDGE('',*,*,#7035,.F.);
#9694=ORIENTED_EDGE('',*,*,#7039,.F.);
#9695=ORIENTED_EDGE('',*,*,#7042,.F.);
#9696=ORIENTED_EDGE('',*,*,#7045,.F.);
#9697=ORIENTED_EDGE('',*,*,#7048,.F.);
#9698=ORIENTED_EDGE('',*,*,#7051,.F.);
#9699=ORIENTED_EDGE('',*,*,#7054,.F.);
#9700=ORIENTED_EDGE('',*,*,#7057,.F.);
#9701=ORIENTED_EDGE('',*,*,#7227,.F.);
#9702=ORIENTED_EDGE('',*,*,#7062,.F.);
#9703=ORIENTED_EDGE('',*,*,#7229,.F.);
#9704=ORIENTED_EDGE('',*,*,#7031,.F.);
#9705=ORIENTED_EDGE('',*,*,#7230,.F.);
#9706=ORIENTED_EDGE('',*,*,#7029,.F.);
#9707=ORIENTED_EDGE('',*,*,#7026,.F.);
#9708=ORIENTED_EDGE('',*,*,#7023,.F.);
#9709=ORIENTED_EDGE('',*,*,#7020,.F.);
#9710=ORIENTED_EDGE('',*,*,#7017,.F.);
#9711=ORIENTED_EDGE('',*,*,#7014,.F.);
#9712=ORIENTED_EDGE('',*,*,#7011,.F.);
#9713=ORIENTED_EDGE('',*,*,#7008,.F.);
#9714=ORIENTED_EDGE('',*,*,#7225,.F.);
#9715=ORIENTED_EDGE('',*,*,#7003,.F.);
#9716=ORIENTED_EDGE('',*,*,#7010,.F.);
#9717=ORIENTED_EDGE('',*,*,#7013,.F.);
#9718=ORIENTED_EDGE('',*,*,#7016,.F.);
#9719=ORIENTED_EDGE('',*,*,#7019,.F.);
#9720=ORIENTED_EDGE('',*,*,#7022,.F.);
#9721=ORIENTED_EDGE('',*,*,#7025,.F.);
#9722=ORIENTED_EDGE('',*,*,#7028,.F.);
#9723=ORIENTED_EDGE('',*,*,#7231,.F.);
#9724=ORIENTED_EDGE('',*,*,#7033,.F.);
#9725=ORIENTED_EDGE('',*,*,#7232,.F.);
#9726=ORIENTED_EDGE('',*,*,#7060,.T.);
#9727=ORIENTED_EDGE('',*,*,#7228,.T.);
#9728=ORIENTED_EDGE('',*,*,#7058,.T.);
#9729=ORIENTED_EDGE('',*,*,#7055,.T.);
#9730=ORIENTED_EDGE('',*,*,#7052,.T.);
#9731=ORIENTED_EDGE('',*,*,#7049,.T.);
#9732=ORIENTED_EDGE('',*,*,#7046,.T.);
#9733=ORIENTED_EDGE('',*,*,#7043,.T.);
#9734=ORIENTED_EDGE('',*,*,#7040,.T.);
#9735=ORIENTED_EDGE('',*,*,#7037,.T.);
#9736=ORIENTED_EDGE('',*,*,#7030,.T.);
#9737=ORIENTED_EDGE('',*,*,#7231,.T.);
#9738=ORIENTED_EDGE('',*,*,#7027,.F.);
#9739=ORIENTED_EDGE('',*,*,#7230,.T.);
#9740=ORIENTED_EDGE('',*,*,#6943,.F.);
#9741=ORIENTED_EDGE('',*,*,#7233,.T.);
#9742=ORIENTED_EDGE('',*,*,#6975,.T.);
#9743=ORIENTED_EDGE('',*,*,#7234,.T.);
#9744=ORIENTED_EDGE('',*,*,#6946,.F.);
#9745=ORIENTED_EDGE('',*,*,#6998,.T.);
#9746=ORIENTED_EDGE('',*,*,#7235,.T.);
#9747=ORIENTED_EDGE('',*,*,#6995,.F.);
#9748=ORIENTED_EDGE('',*,*,#7236,.F.);
#9749=ORIENTED_EDGE('',*,*,#7234,.F.);
#9750=ORIENTED_EDGE('',*,*,#6974,.F.);
#9751=ORIENTED_EDGE('',*,*,#6978,.F.);
#9752=ORIENTED_EDGE('',*,*,#6981,.F.);
#9753=ORIENTED_EDGE('',*,*,#6984,.F.);
#9754=ORIENTED_EDGE('',*,*,#6987,.F.);
#9755=ORIENTED_EDGE('',*,*,#6990,.F.);
#9756=ORIENTED_EDGE('',*,*,#6993,.F.);
#9757=ORIENTED_EDGE('',*,*,#6996,.F.);
#9758=ORIENTED_EDGE('',*,*,#7235,.F.);
#9759=ORIENTED_EDGE('',*,*,#7001,.F.);
#9760=ORIENTED_EDGE('',*,*,#7237,.F.);
#9761=ORIENTED_EDGE('',*,*,#6970,.F.);
#9762=ORIENTED_EDGE('',*,*,#7238,.F.);
#9763=ORIENTED_EDGE('',*,*,#6968,.F.);
#9764=ORIENTED_EDGE('',*,*,#6965,.F.);
#9765=ORIENTED_EDGE('',*,*,#6962,.F.);
#9766=ORIENTED_EDGE('',*,*,#6959,.F.);
#9767=ORIENTED_EDGE('',*,*,#6956,.F.);
#9768=ORIENTED_EDGE('',*,*,#6953,.F.);
#9769=ORIENTED_EDGE('',*,*,#6950,.F.);
#9770=ORIENTED_EDGE('',*,*,#6947,.F.);
#9771=ORIENTED_EDGE('',*,*,#7233,.F.);
#9772=ORIENTED_EDGE('',*,*,#6942,.F.);
#9773=ORIENTED_EDGE('',*,*,#6949,.F.);
#9774=ORIENTED_EDGE('',*,*,#6952,.F.);
#9775=ORIENTED_EDGE('',*,*,#6955,.F.);
#9776=ORIENTED_EDGE('',*,*,#6958,.F.);
#9777=ORIENTED_EDGE('',*,*,#6961,.F.);
#9778=ORIENTED_EDGE('',*,*,#6964,.F.);
#9779=ORIENTED_EDGE('',*,*,#6967,.F.);
#9780=ORIENTED_EDGE('',*,*,#7239,.F.);
#9781=ORIENTED_EDGE('',*,*,#6972,.F.);
#9782=ORIENTED_EDGE('',*,*,#7240,.F.);
#9783=ORIENTED_EDGE('',*,*,#6999,.T.);
#9784=ORIENTED_EDGE('',*,*,#7236,.T.);
#9785=ORIENTED_EDGE('',*,*,#6997,.T.);
#9786=ORIENTED_EDGE('',*,*,#6994,.T.);
#9787=ORIENTED_EDGE('',*,*,#6991,.T.);
#9788=ORIENTED_EDGE('',*,*,#6988,.T.);
#9789=ORIENTED_EDGE('',*,*,#6985,.T.);
#9790=ORIENTED_EDGE('',*,*,#6982,.T.);
#9791=ORIENTED_EDGE('',*,*,#6979,.T.);
#9792=ORIENTED_EDGE('',*,*,#6976,.T.);
#9793=ORIENTED_EDGE('',*,*,#6969,.T.);
#9794=ORIENTED_EDGE('',*,*,#7239,.T.);
#9795=ORIENTED_EDGE('',*,*,#6966,.F.);
#9796=ORIENTED_EDGE('',*,*,#7238,.T.);
#9797=ORIENTED_EDGE('',*,*,#6882,.F.);
#9798=ORIENTED_EDGE('',*,*,#7241,.T.);
#9799=ORIENTED_EDGE('',*,*,#6914,.T.);
#9800=ORIENTED_EDGE('',*,*,#7242,.T.);
#9801=ORIENTED_EDGE('',*,*,#6885,.F.);
#9802=ORIENTED_EDGE('',*,*,#6937,.T.);
#9803=ORIENTED_EDGE('',*,*,#7243,.T.);
#9804=ORIENTED_EDGE('',*,*,#6934,.F.);
#9805=ORIENTED_EDGE('',*,*,#7244,.F.);
#9806=ORIENTED_EDGE('',*,*,#7242,.F.);
#9807=ORIENTED_EDGE('',*,*,#6913,.F.);
#9808=ORIENTED_EDGE('',*,*,#6917,.F.);
#9809=ORIENTED_EDGE('',*,*,#6920,.F.);
#9810=ORIENTED_EDGE('',*,*,#6923,.F.);
#9811=ORIENTED_EDGE('',*,*,#6926,.F.);
#9812=ORIENTED_EDGE('',*,*,#6929,.F.);
#9813=ORIENTED_EDGE('',*,*,#6932,.F.);
#9814=ORIENTED_EDGE('',*,*,#6935,.F.);
#9815=ORIENTED_EDGE('',*,*,#7243,.F.);
#9816=ORIENTED_EDGE('',*,*,#6940,.F.);
#9817=ORIENTED_EDGE('',*,*,#7245,.F.);
#9818=ORIENTED_EDGE('',*,*,#6909,.F.);
#9819=ORIENTED_EDGE('',*,*,#7246,.F.);
#9820=ORIENTED_EDGE('',*,*,#6907,.F.);
#9821=ORIENTED_EDGE('',*,*,#6904,.F.);
#9822=ORIENTED_EDGE('',*,*,#6901,.F.);
#9823=ORIENTED_EDGE('',*,*,#6898,.F.);
#9824=ORIENTED_EDGE('',*,*,#6895,.F.);
#9825=ORIENTED_EDGE('',*,*,#6892,.F.);
#9826=ORIENTED_EDGE('',*,*,#6889,.F.);
#9827=ORIENTED_EDGE('',*,*,#6886,.F.);
#9828=ORIENTED_EDGE('',*,*,#7241,.F.);
#9829=ORIENTED_EDGE('',*,*,#6881,.F.);
#9830=ORIENTED_EDGE('',*,*,#6888,.F.);
#9831=ORIENTED_EDGE('',*,*,#6891,.F.);
#9832=ORIENTED_EDGE('',*,*,#6894,.F.);
#9833=ORIENTED_EDGE('',*,*,#6897,.F.);
#9834=ORIENTED_EDGE('',*,*,#6900,.F.);
#9835=ORIENTED_EDGE('',*,*,#6903,.F.);
#9836=ORIENTED_EDGE('',*,*,#6906,.F.);
#9837=ORIENTED_EDGE('',*,*,#7247,.F.);
#9838=ORIENTED_EDGE('',*,*,#6911,.F.);
#9839=ORIENTED_EDGE('',*,*,#7248,.F.);
#9840=ORIENTED_EDGE('',*,*,#6938,.T.);
#9841=ORIENTED_EDGE('',*,*,#7244,.T.);
#9842=ORIENTED_EDGE('',*,*,#6936,.T.);
#9843=ORIENTED_EDGE('',*,*,#6933,.T.);
#9844=ORIENTED_EDGE('',*,*,#6930,.T.);
#9845=ORIENTED_EDGE('',*,*,#6927,.T.);
#9846=ORIENTED_EDGE('',*,*,#6924,.T.);
#9847=ORIENTED_EDGE('',*,*,#6921,.T.);
#9848=ORIENTED_EDGE('',*,*,#6918,.T.);
#9849=ORIENTED_EDGE('',*,*,#6915,.T.);
#9850=ORIENTED_EDGE('',*,*,#6908,.T.);
#9851=ORIENTED_EDGE('',*,*,#7247,.T.);
#9852=ORIENTED_EDGE('',*,*,#6905,.F.);
#9853=ORIENTED_EDGE('',*,*,#7246,.T.);
#9854=ORIENTED_EDGE('',*,*,#6821,.F.);
#9855=ORIENTED_EDGE('',*,*,#7249,.T.);
#9856=ORIENTED_EDGE('',*,*,#6853,.T.);
#9857=ORIENTED_EDGE('',*,*,#7250,.T.);
#9858=ORIENTED_EDGE('',*,*,#6824,.F.);
#9859=ORIENTED_EDGE('',*,*,#6876,.T.);
#9860=ORIENTED_EDGE('',*,*,#7251,.T.);
#9861=ORIENTED_EDGE('',*,*,#6873,.F.);
#9862=ORIENTED_EDGE('',*,*,#7252,.F.);
#9863=ORIENTED_EDGE('',*,*,#7250,.F.);
#9864=ORIENTED_EDGE('',*,*,#6852,.F.);
#9865=ORIENTED_EDGE('',*,*,#6856,.F.);
#9866=ORIENTED_EDGE('',*,*,#6859,.F.);
#9867=ORIENTED_EDGE('',*,*,#6862,.F.);
#9868=ORIENTED_EDGE('',*,*,#6865,.F.);
#9869=ORIENTED_EDGE('',*,*,#6868,.F.);
#9870=ORIENTED_EDGE('',*,*,#6871,.F.);
#9871=ORIENTED_EDGE('',*,*,#6874,.F.);
#9872=ORIENTED_EDGE('',*,*,#7251,.F.);
#9873=ORIENTED_EDGE('',*,*,#6879,.F.);
#9874=ORIENTED_EDGE('',*,*,#7253,.F.);
#9875=ORIENTED_EDGE('',*,*,#6848,.F.);
#9876=ORIENTED_EDGE('',*,*,#7254,.F.);
#9877=ORIENTED_EDGE('',*,*,#6846,.F.);
#9878=ORIENTED_EDGE('',*,*,#6843,.F.);
#9879=ORIENTED_EDGE('',*,*,#6840,.F.);
#9880=ORIENTED_EDGE('',*,*,#6837,.F.);
#9881=ORIENTED_EDGE('',*,*,#6834,.F.);
#9882=ORIENTED_EDGE('',*,*,#6831,.F.);
#9883=ORIENTED_EDGE('',*,*,#6828,.F.);
#9884=ORIENTED_EDGE('',*,*,#6825,.F.);
#9885=ORIENTED_EDGE('',*,*,#7249,.F.);
#9886=ORIENTED_EDGE('',*,*,#6820,.F.);
#9887=ORIENTED_EDGE('',*,*,#6827,.F.);
#9888=ORIENTED_EDGE('',*,*,#6830,.F.);
#9889=ORIENTED_EDGE('',*,*,#6833,.F.);
#9890=ORIENTED_EDGE('',*,*,#6836,.F.);
#9891=ORIENTED_EDGE('',*,*,#6839,.F.);
#9892=ORIENTED_EDGE('',*,*,#6842,.F.);
#9893=ORIENTED_EDGE('',*,*,#6845,.F.);
#9894=ORIENTED_EDGE('',*,*,#7255,.F.);
#9895=ORIENTED_EDGE('',*,*,#6850,.F.);
#9896=ORIENTED_EDGE('',*,*,#7256,.F.);
#9897=ORIENTED_EDGE('',*,*,#6877,.T.);
#9898=ORIENTED_EDGE('',*,*,#7252,.T.);
#9899=ORIENTED_EDGE('',*,*,#6875,.T.);
#9900=ORIENTED_EDGE('',*,*,#6872,.T.);
#9901=ORIENTED_EDGE('',*,*,#6869,.T.);
#9902=ORIENTED_EDGE('',*,*,#6866,.T.);
#9903=ORIENTED_EDGE('',*,*,#6863,.T.);
#9904=ORIENTED_EDGE('',*,*,#6860,.T.);
#9905=ORIENTED_EDGE('',*,*,#6857,.T.);
#9906=ORIENTED_EDGE('',*,*,#6854,.T.);
#9907=ORIENTED_EDGE('',*,*,#6847,.T.);
#9908=ORIENTED_EDGE('',*,*,#7255,.T.);
#9909=ORIENTED_EDGE('',*,*,#6844,.F.);
#9910=ORIENTED_EDGE('',*,*,#7254,.T.);
#9911=ORIENTED_EDGE('',*,*,#6760,.F.);
#9912=ORIENTED_EDGE('',*,*,#7257,.T.);
#9913=ORIENTED_EDGE('',*,*,#6792,.T.);
#9914=ORIENTED_EDGE('',*,*,#7258,.T.);
#9915=ORIENTED_EDGE('',*,*,#6763,.F.);
#9916=ORIENTED_EDGE('',*,*,#6815,.T.);
#9917=ORIENTED_EDGE('',*,*,#7259,.T.);
#9918=ORIENTED_EDGE('',*,*,#6812,.F.);
#9919=ORIENTED_EDGE('',*,*,#7260,.F.);
#9920=ORIENTED_EDGE('',*,*,#7258,.F.);
#9921=ORIENTED_EDGE('',*,*,#6791,.F.);
#9922=ORIENTED_EDGE('',*,*,#6795,.F.);
#9923=ORIENTED_EDGE('',*,*,#6798,.F.);
#9924=ORIENTED_EDGE('',*,*,#6801,.F.);
#9925=ORIENTED_EDGE('',*,*,#6804,.F.);
#9926=ORIENTED_EDGE('',*,*,#6807,.F.);
#9927=ORIENTED_EDGE('',*,*,#6810,.F.);
#9928=ORIENTED_EDGE('',*,*,#6813,.F.);
#9929=ORIENTED_EDGE('',*,*,#7259,.F.);
#9930=ORIENTED_EDGE('',*,*,#6818,.F.);
#9931=ORIENTED_EDGE('',*,*,#7261,.F.);
#9932=ORIENTED_EDGE('',*,*,#6787,.F.);
#9933=ORIENTED_EDGE('',*,*,#7262,.F.);
#9934=ORIENTED_EDGE('',*,*,#6785,.F.);
#9935=ORIENTED_EDGE('',*,*,#6782,.F.);
#9936=ORIENTED_EDGE('',*,*,#6779,.F.);
#9937=ORIENTED_EDGE('',*,*,#6776,.F.);
#9938=ORIENTED_EDGE('',*,*,#6773,.F.);
#9939=ORIENTED_EDGE('',*,*,#6770,.F.);
#9940=ORIENTED_EDGE('',*,*,#6767,.F.);
#9941=ORIENTED_EDGE('',*,*,#6764,.F.);
#9942=ORIENTED_EDGE('',*,*,#7257,.F.);
#9943=ORIENTED_EDGE('',*,*,#6759,.F.);
#9944=ORIENTED_EDGE('',*,*,#6766,.F.);
#9945=ORIENTED_EDGE('',*,*,#6769,.F.);
#9946=ORIENTED_EDGE('',*,*,#6772,.F.);
#9947=ORIENTED_EDGE('',*,*,#6775,.F.);
#9948=ORIENTED_EDGE('',*,*,#6778,.F.);
#9949=ORIENTED_EDGE('',*,*,#6781,.F.);
#9950=ORIENTED_EDGE('',*,*,#6784,.F.);
#9951=ORIENTED_EDGE('',*,*,#7263,.F.);
#9952=ORIENTED_EDGE('',*,*,#6789,.F.);
#9953=ORIENTED_EDGE('',*,*,#7264,.F.);
#9954=ORIENTED_EDGE('',*,*,#6816,.T.);
#9955=ORIENTED_EDGE('',*,*,#7260,.T.);
#9956=ORIENTED_EDGE('',*,*,#6814,.T.);
#9957=ORIENTED_EDGE('',*,*,#6811,.T.);
#9958=ORIENTED_EDGE('',*,*,#6808,.T.);
#9959=ORIENTED_EDGE('',*,*,#6805,.T.);
#9960=ORIENTED_EDGE('',*,*,#6802,.T.);
#9961=ORIENTED_EDGE('',*,*,#6799,.T.);
#9962=ORIENTED_EDGE('',*,*,#6796,.T.);
#9963=ORIENTED_EDGE('',*,*,#6793,.T.);
#9964=ORIENTED_EDGE('',*,*,#6786,.T.);
#9965=ORIENTED_EDGE('',*,*,#7263,.T.);
#9966=ORIENTED_EDGE('',*,*,#6783,.F.);
#9967=ORIENTED_EDGE('',*,*,#7262,.T.);
#9968=ORIENTED_EDGE('',*,*,#6699,.F.);
#9969=ORIENTED_EDGE('',*,*,#7265,.T.);
#9970=ORIENTED_EDGE('',*,*,#6731,.T.);
#9971=ORIENTED_EDGE('',*,*,#7266,.T.);
#9972=ORIENTED_EDGE('',*,*,#6702,.F.);
#9973=ORIENTED_EDGE('',*,*,#6754,.T.);
#9974=ORIENTED_EDGE('',*,*,#7267,.T.);
#9975=ORIENTED_EDGE('',*,*,#6751,.F.);
#9976=ORIENTED_EDGE('',*,*,#7268,.F.);
#9977=ORIENTED_EDGE('',*,*,#7266,.F.);
#9978=ORIENTED_EDGE('',*,*,#6730,.F.);
#9979=ORIENTED_EDGE('',*,*,#6734,.F.);
#9980=ORIENTED_EDGE('',*,*,#6737,.F.);
#9981=ORIENTED_EDGE('',*,*,#6740,.F.);
#9982=ORIENTED_EDGE('',*,*,#6743,.F.);
#9983=ORIENTED_EDGE('',*,*,#6746,.F.);
#9984=ORIENTED_EDGE('',*,*,#6749,.F.);
#9985=ORIENTED_EDGE('',*,*,#6752,.F.);
#9986=ORIENTED_EDGE('',*,*,#7267,.F.);
#9987=ORIENTED_EDGE('',*,*,#6757,.F.);
#9988=ORIENTED_EDGE('',*,*,#7269,.F.);
#9989=ORIENTED_EDGE('',*,*,#6726,.F.);
#9990=ORIENTED_EDGE('',*,*,#7270,.F.);
#9991=ORIENTED_EDGE('',*,*,#6724,.F.);
#9992=ORIENTED_EDGE('',*,*,#6721,.F.);
#9993=ORIENTED_EDGE('',*,*,#6718,.F.);
#9994=ORIENTED_EDGE('',*,*,#6715,.F.);
#9995=ORIENTED_EDGE('',*,*,#6712,.F.);
#9996=ORIENTED_EDGE('',*,*,#6709,.F.);
#9997=ORIENTED_EDGE('',*,*,#6706,.F.);
#9998=ORIENTED_EDGE('',*,*,#6703,.F.);
#9999=ORIENTED_EDGE('',*,*,#7265,.F.);
#10000=ORIENTED_EDGE('',*,*,#6698,.F.);
#10001=ORIENTED_EDGE('',*,*,#6705,.F.);
#10002=ORIENTED_EDGE('',*,*,#6708,.F.);
#10003=ORIENTED_EDGE('',*,*,#6711,.F.);
#10004=ORIENTED_EDGE('',*,*,#6714,.F.);
#10005=ORIENTED_EDGE('',*,*,#6717,.F.);
#10006=ORIENTED_EDGE('',*,*,#6720,.F.);
#10007=ORIENTED_EDGE('',*,*,#6723,.F.);
#10008=ORIENTED_EDGE('',*,*,#7271,.F.);
#10009=ORIENTED_EDGE('',*,*,#6728,.F.);
#10010=ORIENTED_EDGE('',*,*,#7272,.F.);
#10011=ORIENTED_EDGE('',*,*,#6755,.T.);
#10012=ORIENTED_EDGE('',*,*,#7268,.T.);
#10013=ORIENTED_EDGE('',*,*,#6753,.T.);
#10014=ORIENTED_EDGE('',*,*,#6750,.T.);
#10015=ORIENTED_EDGE('',*,*,#6747,.T.);
#10016=ORIENTED_EDGE('',*,*,#6744,.T.);
#10017=ORIENTED_EDGE('',*,*,#6741,.T.);
#10018=ORIENTED_EDGE('',*,*,#6738,.T.);
#10019=ORIENTED_EDGE('',*,*,#6735,.T.);
#10020=ORIENTED_EDGE('',*,*,#6732,.T.);
#10021=ORIENTED_EDGE('',*,*,#6725,.T.);
#10022=ORIENTED_EDGE('',*,*,#7271,.T.);
#10023=ORIENTED_EDGE('',*,*,#6722,.F.);
#10024=ORIENTED_EDGE('',*,*,#7270,.T.);
#10025=ORIENTED_EDGE('',*,*,#7273,.F.);
#10026=ORIENTED_EDGE('',*,*,#7274,.T.);
#10027=ORIENTED_EDGE('',*,*,#7275,.F.);
#10028=ORIENTED_EDGE('',*,*,#7276,.F.);
#10029=ORIENTED_EDGE('',*,*,#7277,.F.);
#10030=ORIENTED_EDGE('',*,*,#7278,.F.);
#10031=ORIENTED_EDGE('',*,*,#7275,.T.);
#10032=ORIENTED_EDGE('',*,*,#7279,.T.);
#10033=ORIENTED_EDGE('',*,*,#7280,.F.);
#10034=ORIENTED_EDGE('',*,*,#7281,.F.);
#10035=ORIENTED_EDGE('',*,*,#7282,.F.);
#10036=ORIENTED_EDGE('',*,*,#7283,.F.);
#10037=ORIENTED_EDGE('',*,*,#7284,.F.);
#10038=ORIENTED_EDGE('',*,*,#7285,.F.);
#10039=ORIENTED_EDGE('',*,*,#7286,.F.);
#10040=ORIENTED_EDGE('',*,*,#7287,.F.);
#10041=ORIENTED_EDGE('',*,*,#7288,.F.);
#10042=ORIENTED_EDGE('',*,*,#7289,.F.);
#10043=ORIENTED_EDGE('',*,*,#7280,.T.);
#10044=ORIENTED_EDGE('',*,*,#7290,.T.);
#10045=ORIENTED_EDGE('',*,*,#7291,.F.);
#10046=ORIENTED_EDGE('',*,*,#7290,.F.);
#10047=ORIENTED_EDGE('',*,*,#7279,.F.);
#10048=ORIENTED_EDGE('',*,*,#7274,.F.);
#10049=ORIENTED_EDGE('',*,*,#7224,.T.);
#10050=ORIENTED_EDGE('',*,*,#7093,.T.);
#10051=ORIENTED_EDGE('',*,*,#7221,.T.);
#10052=ORIENTED_EDGE('',*,*,#7122,.T.);
#10053=ORIENTED_EDGE('',*,*,#7248,.T.);
#10054=ORIENTED_EDGE('',*,*,#6910,.T.);
#10055=ORIENTED_EDGE('',*,*,#7245,.T.);
#10056=ORIENTED_EDGE('',*,*,#6939,.T.);
#10057=ORIENTED_EDGE('',*,*,#7292,.F.);
#10058=ORIENTED_EDGE('',*,*,#7293,.F.);
#10059=ORIENTED_EDGE('',*,*,#7294,.T.);
#10060=ORIENTED_EDGE('',*,*,#7295,.T.);
#10061=ORIENTED_EDGE('',*,*,#7296,.F.);
#10062=ORIENTED_EDGE('',*,*,#7297,.F.);
#10063=ORIENTED_EDGE('',*,*,#7298,.F.);
#10064=ORIENTED_EDGE('',*,*,#7299,.F.);
#10065=ORIENTED_EDGE('',*,*,#7300,.F.);
#10066=ORIENTED_EDGE('',*,*,#7301,.F.);
#10067=ORIENTED_EDGE('',*,*,#7302,.F.);
#10068=ORIENTED_EDGE('',*,*,#7303,.F.);
#10069=ORIENTED_EDGE('',*,*,#7304,.F.);
#10070=ORIENTED_EDGE('',*,*,#7305,.T.);
#10071=ORIENTED_EDGE('',*,*,#7294,.F.);
#10072=ORIENTED_EDGE('',*,*,#7306,.F.);
#10073=ORIENTED_EDGE('',*,*,#7307,.F.);
#10074=ORIENTED_EDGE('',*,*,#7308,.F.);
#10075=ORIENTED_EDGE('',*,*,#7296,.T.);
#10076=ORIENTED_EDGE('',*,*,#7309,.T.);
#10077=ORIENTED_EDGE('',*,*,#7310,.F.);
#10078=ORIENTED_EDGE('',*,*,#7309,.F.);
#10079=ORIENTED_EDGE('',*,*,#7295,.F.);
#10080=ORIENTED_EDGE('',*,*,#7305,.F.);
#10081=ORIENTED_EDGE('',*,*,#7232,.T.);
#10082=ORIENTED_EDGE('',*,*,#7032,.T.);
#10083=ORIENTED_EDGE('',*,*,#7229,.T.);
#10084=ORIENTED_EDGE('',*,*,#7061,.T.);
#10085=ORIENTED_EDGE('',*,*,#7256,.T.);
#10086=ORIENTED_EDGE('',*,*,#6849,.T.);
#10087=ORIENTED_EDGE('',*,*,#7253,.T.);
#10088=ORIENTED_EDGE('',*,*,#6878,.T.);
#10089=ORIENTED_EDGE('',*,*,#7285,.T.);
#10090=ORIENTED_EDGE('',*,*,#7311,.F.);
#10091=ORIENTED_EDGE('',*,*,#7312,.F.);
#10092=ORIENTED_EDGE('',*,*,#7313,.F.);
#10093=ORIENTED_EDGE('',*,*,#7314,.F.);
#10094=ORIENTED_EDGE('',*,*,#7315,.F.);
#10095=ORIENTED_EDGE('',*,*,#7284,.T.);
#10096=ORIENTED_EDGE('',*,*,#7316,.T.);
#10097=ORIENTED_EDGE('',*,*,#7317,.T.);
#10098=ORIENTED_EDGE('',*,*,#7311,.T.);
#10099=ORIENTED_EDGE('',*,*,#7289,.T.);
#10100=ORIENTED_EDGE('',*,*,#7318,.T.);
#10101=ORIENTED_EDGE('',*,*,#7319,.T.);
#10102=ORIENTED_EDGE('',*,*,#7320,.T.);
#10103=ORIENTED_EDGE('',*,*,#7321,.T.);
#10104=ORIENTED_EDGE('',*,*,#7322,.T.);
#10105=ORIENTED_EDGE('',*,*,#7323,.T.);
#10106=ORIENTED_EDGE('',*,*,#7324,.T.);
#10107=ORIENTED_EDGE('',*,*,#7325,.T.);
#10108=ORIENTED_EDGE('',*,*,#7281,.T.);
#10109=ORIENTED_EDGE('',*,*,#7185,.T.);
#10110=ORIENTED_EDGE('',*,*,#7276,.T.);
#10111=ORIENTED_EDGE('',*,*,#7278,.T.);
#10112=ORIENTED_EDGE('',*,*,#7326,.T.);
#10113=ORIENTED_EDGE('',*,*,#7327,.T.);
#10114=ORIENTED_EDGE('',*,*,#7328,.T.);
#10115=ORIENTED_EDGE('',*,*,#7329,.T.);
#10116=ORIENTED_EDGE('',*,*,#7330,.T.);
#10117=ORIENTED_EDGE('',*,*,#7331,.T.);
#10118=ORIENTED_EDGE('',*,*,#7332,.T.);
#10119=ORIENTED_EDGE('',*,*,#7333,.T.);
#10120=ORIENTED_EDGE('',*,*,#7189,.T.);
#10121=ORIENTED_EDGE('',*,*,#7283,.T.);
#10122=ORIENTED_EDGE('',*,*,#7334,.F.);
#10123=ORIENTED_EDGE('',*,*,#7335,.F.);
#10124=ORIENTED_EDGE('',*,*,#7316,.F.);
#10125=ORIENTED_EDGE('',*,*,#7282,.T.);
#10126=ORIENTED_EDGE('',*,*,#7325,.F.);
#10127=ORIENTED_EDGE('',*,*,#7336,.T.);
#10128=ORIENTED_EDGE('',*,*,#7334,.T.);
#10129=ORIENTED_EDGE('',*,*,#7301,.T.);
#10130=ORIENTED_EDGE('',*,*,#7337,.F.);
#10131=ORIENTED_EDGE('',*,*,#7338,.F.);
#10132=ORIENTED_EDGE('',*,*,#7339,.F.);
#10133=ORIENTED_EDGE('',*,*,#7340,.F.);
#10134=ORIENTED_EDGE('',*,*,#7341,.F.);
#10135=ORIENTED_EDGE('',*,*,#7300,.T.);
#10136=ORIENTED_EDGE('',*,*,#7342,.T.);
#10137=ORIENTED_EDGE('',*,*,#7343,.T.);
#10138=ORIENTED_EDGE('',*,*,#7337,.T.);
#10139=ORIENTED_EDGE('',*,*,#7299,.T.);
#10140=ORIENTED_EDGE('',*,*,#7344,.F.);
#10141=ORIENTED_EDGE('',*,*,#7345,.F.);
#10142=ORIENTED_EDGE('',*,*,#7342,.F.);
#10143=ORIENTED_EDGE('',*,*,#7298,.T.);
#10144=ORIENTED_EDGE('',*,*,#7346,.F.);
#10145=ORIENTED_EDGE('',*,*,#7347,.T.);
#10146=ORIENTED_EDGE('',*,*,#7344,.T.);
#10147=ORIENTED_EDGE('',*,*,#7297,.T.);
#10148=ORIENTED_EDGE('',*,*,#7308,.T.);
#10149=ORIENTED_EDGE('',*,*,#7348,.T.);
#10150=ORIENTED_EDGE('',*,*,#7349,.T.);
#10151=ORIENTED_EDGE('',*,*,#7350,.T.);
#10152=ORIENTED_EDGE('',*,*,#7351,.T.);
#10153=ORIENTED_EDGE('',*,*,#7352,.T.);
#10154=ORIENTED_EDGE('',*,*,#7353,.T.);
#10155=ORIENTED_EDGE('',*,*,#7354,.T.);
#10156=ORIENTED_EDGE('',*,*,#7346,.T.);
#10157=ORIENTED_EDGE('',*,*,#7193,.T.);
#10158=ORIENTED_EDGE('',*,*,#7286,.T.);
#10159=ORIENTED_EDGE('',*,*,#7315,.T.);
#10160=ORIENTED_EDGE('',*,*,#7355,.F.);
#10161=ORIENTED_EDGE('',*,*,#7356,.T.);
#10162=ORIENTED_EDGE('',*,*,#7287,.T.);
#10163=ORIENTED_EDGE('',*,*,#7356,.F.);
#10164=ORIENTED_EDGE('',*,*,#7357,.F.);
#10165=ORIENTED_EDGE('',*,*,#7358,.F.);
#10166=ORIENTED_EDGE('',*,*,#7303,.T.);
#10167=ORIENTED_EDGE('',*,*,#7359,.F.);
#10168=ORIENTED_EDGE('',*,*,#7360,.F.);
#10169=ORIENTED_EDGE('',*,*,#7361,.F.);
#10170=ORIENTED_EDGE('',*,*,#7302,.T.);
#10171=ORIENTED_EDGE('',*,*,#7341,.T.);
#10172=ORIENTED_EDGE('',*,*,#7362,.F.);
#10173=ORIENTED_EDGE('',*,*,#7359,.T.);
#10174=ORIENTED_EDGE('',*,*,#7363,.T.);
#10175=ORIENTED_EDGE('',*,*,#7313,.T.);
#10176=ORIENTED_EDGE('',*,*,#7364,.T.);
#10177=ORIENTED_EDGE('',*,*,#7323,.F.);
#10178=ORIENTED_EDGE('',*,*,#7365,.T.);
#10179=ORIENTED_EDGE('',*,*,#7366,.T.);
#10180=ORIENTED_EDGE('',*,*,#7367,.T.);
#10181=ORIENTED_EDGE('',*,*,#7368,.F.);
#10182=ORIENTED_EDGE('',*,*,#7369,.T.);
#10183=ORIENTED_EDGE('',*,*,#7339,.T.);
#10184=ORIENTED_EDGE('',*,*,#7370,.T.);
#10185=ORIENTED_EDGE('',*,*,#7353,.F.);
#10186=ORIENTED_EDGE('',*,*,#7371,.T.);
#10187=ORIENTED_EDGE('',*,*,#7372,.T.);
#10188=ORIENTED_EDGE('',*,*,#7373,.T.);
#10189=ORIENTED_EDGE('',*,*,#7374,.T.);
#10190=ORIENTED_EDGE('',*,*,#7373,.F.);
#10191=ORIENTED_EDGE('',*,*,#7375,.T.);
#10192=ORIENTED_EDGE('',*,*,#7376,.T.);
#10193=ORIENTED_EDGE('',*,*,#7328,.F.);
#10194=ORIENTED_EDGE('',*,*,#7363,.F.);
#10195=ORIENTED_EDGE('',*,*,#7327,.F.);
#10196=ORIENTED_EDGE('',*,*,#7377,.T.);
#10197=ORIENTED_EDGE('',*,*,#7357,.T.);
#10198=ORIENTED_EDGE('',*,*,#7378,.T.);
#10199=ORIENTED_EDGE('',*,*,#7314,.T.);
#10200=ORIENTED_EDGE('',*,*,#7364,.F.);
#10201=ORIENTED_EDGE('',*,*,#7312,.T.);
#10202=ORIENTED_EDGE('',*,*,#7379,.F.);
#10203=ORIENTED_EDGE('',*,*,#7335,.T.);
#10204=ORIENTED_EDGE('',*,*,#7336,.F.);
#10205=ORIENTED_EDGE('',*,*,#7324,.F.);
#10206=ORIENTED_EDGE('',*,*,#7277,.T.);
#10207=ORIENTED_EDGE('',*,*,#7358,.T.);
#10208=ORIENTED_EDGE('',*,*,#7377,.F.);
#10209=ORIENTED_EDGE('',*,*,#7326,.F.);
#10210=ORIENTED_EDGE('',*,*,#7370,.F.);
#10211=ORIENTED_EDGE('',*,*,#7338,.T.);
#10212=ORIENTED_EDGE('',*,*,#7380,.F.);
#10213=ORIENTED_EDGE('',*,*,#7345,.T.);
#10214=ORIENTED_EDGE('',*,*,#7347,.F.);
#10215=ORIENTED_EDGE('',*,*,#7354,.F.);
#10216=ORIENTED_EDGE('',*,*,#7369,.F.);
#10217=ORIENTED_EDGE('',*,*,#7381,.F.);
#10218=ORIENTED_EDGE('',*,*,#7382,.T.);
#10219=ORIENTED_EDGE('',*,*,#7360,.T.);
#10220=ORIENTED_EDGE('',*,*,#7383,.T.);
#10221=ORIENTED_EDGE('',*,*,#7340,.T.);
#10222=ORIENTED_EDGE('',*,*,#7292,.T.);
#10223=ORIENTED_EDGE('',*,*,#7361,.T.);
#10224=ORIENTED_EDGE('',*,*,#7382,.F.);
#10225=ORIENTED_EDGE('',*,*,#7384,.F.);
#10226=ORIENTED_EDGE('',*,*,#7385,.F.);
#10227=ORIENTED_EDGE('',*,*,#7332,.F.);
#10228=ORIENTED_EDGE('',*,*,#7386,.T.);
#10229=ORIENTED_EDGE('',*,*,#7387,.T.);
#10230=ORIENTED_EDGE('',*,*,#7388,.F.);
#10231=ORIENTED_EDGE('',*,*,#7387,.F.);
#10232=ORIENTED_EDGE('',*,*,#7389,.F.);
#10233=ORIENTED_EDGE('',*,*,#7390,.F.);
#10234=ORIENTED_EDGE('',*,*,#7391,.F.);
#10235=ORIENTED_EDGE('',*,*,#7216,.T.);
#10236=ORIENTED_EDGE('',*,*,#7154,.T.);
#10237=ORIENTED_EDGE('',*,*,#7213,.T.);
#10238=ORIENTED_EDGE('',*,*,#7183,.T.);
#10239=ORIENTED_EDGE('',*,*,#7272,.T.);
#10240=ORIENTED_EDGE('',*,*,#6727,.T.);
#10241=ORIENTED_EDGE('',*,*,#7269,.T.);
#10242=ORIENTED_EDGE('',*,*,#6756,.T.);
#10243=ORIENTED_EDGE('',*,*,#7392,.F.);
#10244=ORIENTED_EDGE('',*,*,#7393,.F.);
#10245=ORIENTED_EDGE('',*,*,#7394,.F.);
#10246=ORIENTED_EDGE('',*,*,#7395,.F.);
#10247=ORIENTED_EDGE('',*,*,#7396,.F.);
#10248=ORIENTED_EDGE('',*,*,#7397,.F.);
#10249=ORIENTED_EDGE('',*,*,#7398,.F.);
#10250=ORIENTED_EDGE('',*,*,#7350,.F.);
#10251=ORIENTED_EDGE('',*,*,#7399,.T.);
#10252=ORIENTED_EDGE('',*,*,#7389,.T.);
#10253=ORIENTED_EDGE('',*,*,#7386,.F.);
#10254=ORIENTED_EDGE('',*,*,#7331,.F.);
#10255=ORIENTED_EDGE('',*,*,#7400,.F.);
#10256=ORIENTED_EDGE('',*,*,#7390,.T.);
#10257=ORIENTED_EDGE('',*,*,#7399,.F.);
#10258=ORIENTED_EDGE('',*,*,#7349,.F.);
#10259=ORIENTED_EDGE('',*,*,#7401,.F.);
#10260=ORIENTED_EDGE('',*,*,#7402,.T.);
#10261=ORIENTED_EDGE('',*,*,#7403,.F.);
#10262=ORIENTED_EDGE('',*,*,#7319,.F.);
#10263=ORIENTED_EDGE('',*,*,#7404,.F.);
#10264=ORIENTED_EDGE('',*,*,#7320,.F.);
#10265=ORIENTED_EDGE('',*,*,#7403,.T.);
#10266=ORIENTED_EDGE('',*,*,#7405,.T.);
#10267=ORIENTED_EDGE('',*,*,#7406,.F.);
#10268=ORIENTED_EDGE('',*,*,#7407,.F.);
#10269=ORIENTED_EDGE('',*,*,#7408,.F.);
#10270=ORIENTED_EDGE('',*,*,#7409,.F.);
#10271=ORIENTED_EDGE('',*,*,#7410,.F.);
#10272=ORIENTED_EDGE('',*,*,#7411,.F.);
#10273=ORIENTED_EDGE('',*,*,#7412,.F.);
#10274=ORIENTED_EDGE('',*,*,#7413,.F.);
#10275=ORIENTED_EDGE('',*,*,#7414,.F.);
#10276=ORIENTED_EDGE('',*,*,#7415,.F.);
#10277=ORIENTED_EDGE('',*,*,#7406,.T.);
#10278=ORIENTED_EDGE('',*,*,#7416,.T.);
#10279=ORIENTED_EDGE('',*,*,#7417,.F.);
#10280=ORIENTED_EDGE('',*,*,#7416,.F.);
#10281=ORIENTED_EDGE('',*,*,#7405,.F.);
#10282=ORIENTED_EDGE('',*,*,#7402,.F.);
#10283=ORIENTED_EDGE('',*,*,#7240,.T.);
#10284=ORIENTED_EDGE('',*,*,#6971,.T.);
#10285=ORIENTED_EDGE('',*,*,#7237,.T.);
#10286=ORIENTED_EDGE('',*,*,#7000,.T.);
#10287=ORIENTED_EDGE('',*,*,#7264,.T.);
#10288=ORIENTED_EDGE('',*,*,#6788,.T.);
#10289=ORIENTED_EDGE('',*,*,#7261,.T.);
#10290=ORIENTED_EDGE('',*,*,#6817,.T.);
#10291=ORIENTED_EDGE('',*,*,#7394,.T.);
#10292=ORIENTED_EDGE('',*,*,#7418,.T.);
#10293=ORIENTED_EDGE('',*,*,#7355,.T.);
#10294=ORIENTED_EDGE('',*,*,#7419,.T.);
#10295=ORIENTED_EDGE('',*,*,#7393,.T.);
#10296=ORIENTED_EDGE('',*,*,#7420,.F.);
#10297=ORIENTED_EDGE('',*,*,#7421,.F.);
#10298=ORIENTED_EDGE('',*,*,#7418,.F.);
#10299=ORIENTED_EDGE('',*,*,#7392,.T.);
#10300=ORIENTED_EDGE('',*,*,#7330,.F.);
#10301=ORIENTED_EDGE('',*,*,#7422,.T.);
#10302=ORIENTED_EDGE('',*,*,#7420,.T.);
#10303=ORIENTED_EDGE('',*,*,#7273,.T.);
#10304=ORIENTED_EDGE('',*,*,#7333,.F.);
#10305=ORIENTED_EDGE('',*,*,#7385,.T.);
#10306=ORIENTED_EDGE('',*,*,#7388,.T.);
#10307=ORIENTED_EDGE('',*,*,#7423,.T.);
#10308=ORIENTED_EDGE('',*,*,#7424,.T.);
#10309=ORIENTED_EDGE('',*,*,#7423,.F.);
#10310=ORIENTED_EDGE('',*,*,#7391,.T.);
#10311=ORIENTED_EDGE('',*,*,#7400,.T.);
#10312=ORIENTED_EDGE('',*,*,#7348,.F.);
#10313=ORIENTED_EDGE('',*,*,#7307,.T.);
#10314=ORIENTED_EDGE('',*,*,#7310,.T.);
#10315=ORIENTED_EDGE('',*,*,#7304,.T.);
#10316=ORIENTED_EDGE('',*,*,#7425,.F.);
#10317=ORIENTED_EDGE('',*,*,#7414,.T.);
#10318=ORIENTED_EDGE('',*,*,#7417,.T.);
#10319=ORIENTED_EDGE('',*,*,#7401,.T.);
#10320=ORIENTED_EDGE('',*,*,#7318,.F.);
#10321=ORIENTED_EDGE('',*,*,#7288,.T.);
#10322=ORIENTED_EDGE('',*,*,#7291,.T.);
#10323=ORIENTED_EDGE('',*,*,#7404,.T.);
#10324=ORIENTED_EDGE('',*,*,#7426,.T.);
#10325=ORIENTED_EDGE('',*,*,#7427,.F.);
#10326=ORIENTED_EDGE('',*,*,#7321,.F.);
#10327=ORIENTED_EDGE('',*,*,#7413,.T.);
#10328=ORIENTED_EDGE('',*,*,#7428,.F.);
#10329=ORIENTED_EDGE('',*,*,#7429,.F.);
#10330=ORIENTED_EDGE('',*,*,#7426,.F.);
#10331=ORIENTED_EDGE('',*,*,#7293,.T.);
#10332=ORIENTED_EDGE('',*,*,#7384,.T.);
#10333=ORIENTED_EDGE('',*,*,#7381,.T.);
#10334=ORIENTED_EDGE('',*,*,#7368,.T.);
#10335=ORIENTED_EDGE('',*,*,#7430,.T.);
#10336=ORIENTED_EDGE('',*,*,#7431,.T.);
#10337=ORIENTED_EDGE('',*,*,#7407,.T.);
#10338=ORIENTED_EDGE('',*,*,#7415,.T.);
#10339=ORIENTED_EDGE('',*,*,#7425,.T.);
#10340=ORIENTED_EDGE('',*,*,#7306,.T.);
#10341=ORIENTED_EDGE('',*,*,#7197,.T.);
#10342=ORIENTED_EDGE('',*,*,#7412,.T.);
#10343=ORIENTED_EDGE('',*,*,#7432,.T.);
#10344=ORIENTED_EDGE('',*,*,#7317,.F.);
#10345=ORIENTED_EDGE('',*,*,#7428,.T.);
#10346=ORIENTED_EDGE('',*,*,#7411,.T.);
#10347=ORIENTED_EDGE('',*,*,#7433,.F.);
#10348=ORIENTED_EDGE('',*,*,#7434,.F.);
#10349=ORIENTED_EDGE('',*,*,#7366,.F.);
#10350=ORIENTED_EDGE('',*,*,#7435,.F.);
#10351=ORIENTED_EDGE('',*,*,#7432,.F.);
#10352=ORIENTED_EDGE('',*,*,#7410,.T.);
#10353=ORIENTED_EDGE('',*,*,#7436,.T.);
#10354=ORIENTED_EDGE('',*,*,#7362,.T.);
#10355=ORIENTED_EDGE('',*,*,#7433,.T.);
#10356=ORIENTED_EDGE('',*,*,#7395,.T.);
#10357=ORIENTED_EDGE('',*,*,#7419,.F.);
#10358=ORIENTED_EDGE('',*,*,#7437,.F.);
#10359=ORIENTED_EDGE('',*,*,#7375,.F.);
#10360=ORIENTED_EDGE('',*,*,#7372,.F.);
#10361=ORIENTED_EDGE('',*,*,#7438,.F.);
#10362=ORIENTED_EDGE('',*,*,#7439,.F.);
#10363=ORIENTED_EDGE('',*,*,#7397,.T.);
#10364=ORIENTED_EDGE('',*,*,#7440,.F.);
#10365=ORIENTED_EDGE('',*,*,#7441,.F.);
#10366=ORIENTED_EDGE('',*,*,#7442,.F.);
#10367=ORIENTED_EDGE('',*,*,#7396,.T.);
#10368=ORIENTED_EDGE('',*,*,#7439,.T.);
#10369=ORIENTED_EDGE('',*,*,#7343,.F.);
#10370=ORIENTED_EDGE('',*,*,#7440,.T.);
#10371=ORIENTED_EDGE('',*,*,#7409,.T.);
#10372=ORIENTED_EDGE('',*,*,#7443,.F.);
#10373=ORIENTED_EDGE('',*,*,#7444,.F.);
#10374=ORIENTED_EDGE('',*,*,#7436,.F.);
#10375=ORIENTED_EDGE('',*,*,#7376,.F.);
#10376=ORIENTED_EDGE('',*,*,#7437,.T.);
#10377=ORIENTED_EDGE('',*,*,#7378,.F.);
#10378=ORIENTED_EDGE('',*,*,#7421,.T.);
#10379=ORIENTED_EDGE('',*,*,#7422,.F.);
#10380=ORIENTED_EDGE('',*,*,#7329,.F.);
#10381=ORIENTED_EDGE('',*,*,#7371,.F.);
#10382=ORIENTED_EDGE('',*,*,#7352,.F.);
#10383=ORIENTED_EDGE('',*,*,#7445,.T.);
#10384=ORIENTED_EDGE('',*,*,#7441,.T.);
#10385=ORIENTED_EDGE('',*,*,#7380,.T.);
#10386=ORIENTED_EDGE('',*,*,#7438,.T.);
#10387=ORIENTED_EDGE('',*,*,#7398,.T.);
#10388=ORIENTED_EDGE('',*,*,#7442,.T.);
#10389=ORIENTED_EDGE('',*,*,#7445,.F.);
#10390=ORIENTED_EDGE('',*,*,#7351,.F.);
#10391=ORIENTED_EDGE('',*,*,#7365,.F.);
#10392=ORIENTED_EDGE('',*,*,#7322,.F.);
#10393=ORIENTED_EDGE('',*,*,#7427,.T.);
#10394=ORIENTED_EDGE('',*,*,#7429,.T.);
#10395=ORIENTED_EDGE('',*,*,#7379,.T.);
#10396=ORIENTED_EDGE('',*,*,#7435,.T.);
#10397=ORIENTED_EDGE('',*,*,#7408,.T.);
#10398=ORIENTED_EDGE('',*,*,#7431,.F.);
#10399=ORIENTED_EDGE('',*,*,#7446,.T.);
#10400=ORIENTED_EDGE('',*,*,#7443,.T.);
#10401=ORIENTED_EDGE('',*,*,#7367,.F.);
#10402=ORIENTED_EDGE('',*,*,#7434,.T.);
#10403=ORIENTED_EDGE('',*,*,#7383,.F.);
#10404=ORIENTED_EDGE('',*,*,#7444,.T.);
#10405=ORIENTED_EDGE('',*,*,#7446,.F.);
#10406=ORIENTED_EDGE('',*,*,#7430,.F.);
#10407=ORIENTED_EDGE('',*,*,#7447,.F.);
#10408=ORIENTED_EDGE('',*,*,#7448,.T.);
#10409=ORIENTED_EDGE('',*,*,#7449,.T.);
#10410=ORIENTED_EDGE('',*,*,#7448,.F.);
#10411=ORIENTED_EDGE('',*,*,#7449,.F.);
#10412=ORIENTED_EDGE('',*,*,#7374,.F.);
#10413=ORIENTED_EDGE('',*,*,#7424,.F.);
#10414=ORIENTED_EDGE('',*,*,#6884,.T.);
#10415=ORIENTED_EDGE('',*,*,#7128,.T.);
#10416=ORIENTED_EDGE('',*,*,#7006,.T.);
#10417=ORIENTED_EDGE('',*,*,#6945,.T.);
#10418=ORIENTED_EDGE('',*,*,#6762,.T.);
#10419=ORIENTED_EDGE('',*,*,#6823,.T.);
#10420=ORIENTED_EDGE('',*,*,#6701,.T.);
#10421=ORIENTED_EDGE('',*,*,#7067,.T.);
#10422=ORIENTED_EDGE('',*,*,#7447,.T.);
#10423=ORIENTED_EDGE('',*,*,#7208,.T.);
#10424=ORIENTED_EDGE('',*,*,#7206,.T.);
#10425=ORIENTED_EDGE('',*,*,#7204,.T.);
#10426=ORIENTED_EDGE('',*,*,#7202,.T.);
#13369=CYLINDRICAL_SURFACE('',#14866,2.5175);
#13370=CYLINDRICAL_SURFACE('',#14870,2.5175);
#13371=CYLINDRICAL_SURFACE('',#14871,2.5175);
#13372=CYLINDRICAL_SURFACE('',#14872,2.5175);
#13373=CYLINDRICAL_SURFACE('',#14873,2.5175);
#13374=CYLINDRICAL_SURFACE('',#14874,2.5175);
#13375=CYLINDRICAL_SURFACE('',#14875,2.5175);
#13376=CYLINDRICAL_SURFACE('',#14876,2.5175);
#13377=CYLINDRICAL_SURFACE('',#14877,2.5175);
#13378=CYLINDRICAL_SURFACE('',#14879,3.0735);
#13379=CYLINDRICAL_SURFACE('',#14881,3.0735);
#13380=CYLINDRICAL_SURFACE('',#14882,3.0735);
#13381=CYLINDRICAL_SURFACE('',#14883,3.0735);
#13382=CYLINDRICAL_SURFACE('',#14884,3.0735);
#13383=CYLINDRICAL_SURFACE('',#14885,3.0735);
#13384=CYLINDRICAL_SURFACE('',#14886,3.0735);
#13385=CYLINDRICAL_SURFACE('',#14887,3.0735);
#13386=CYLINDRICAL_SURFACE('',#14888,3.0735);
#13387=CYLINDRICAL_SURFACE('',#14890,2.5175);
#13388=CYLINDRICAL_SURFACE('',#14894,2.5175);
#13389=CYLINDRICAL_SURFACE('',#14895,2.5175);
#13390=CYLINDRICAL_SURFACE('',#14896,2.5175);
#13391=CYLINDRICAL_SURFACE('',#14897,2.5175);
#13392=CYLINDRICAL_SURFACE('',#14898,2.5175);
#13393=CYLINDRICAL_SURFACE('',#14899,2.5175);
#13394=CYLINDRICAL_SURFACE('',#14900,2.5175);
#13395=CYLINDRICAL_SURFACE('',#14901,2.5175);
#13396=CYLINDRICAL_SURFACE('',#14903,3.0735);
#13397=CYLINDRICAL_SURFACE('',#14905,3.0735);
#13398=CYLINDRICAL_SURFACE('',#14906,3.0735);
#13399=CYLINDRICAL_SURFACE('',#14907,3.0735);
#13400=CYLINDRICAL_SURFACE('',#14908,3.0735);
#13401=CYLINDRICAL_SURFACE('',#14909,3.0735);
#13402=CYLINDRICAL_SURFACE('',#14910,3.0735);
#13403=CYLINDRICAL_SURFACE('',#14911,3.0735);
#13404=CYLINDRICAL_SURFACE('',#14912,3.0735);
#13405=CYLINDRICAL_SURFACE('',#14914,2.5175);
#13406=CYLINDRICAL_SURFACE('',#14918,2.5175);
#13407=CYLINDRICAL_SURFACE('',#14919,2.5175);
#13408=CYLINDRICAL_SURFACE('',#14920,2.5175);
#13409=CYLINDRICAL_SURFACE('',#14921,2.5175);
#13410=CYLINDRICAL_SURFACE('',#14922,2.5175);
#13411=CYLINDRICAL_SURFACE('',#14923,2.5175);
#13412=CYLINDRICAL_SURFACE('',#14924,2.5175);
#13413=CYLINDRICAL_SURFACE('',#14925,2.5175);
#13414=CYLINDRICAL_SURFACE('',#14927,3.0735);
#13415=CYLINDRICAL_SURFACE('',#14929,3.0735);
#13416=CYLINDRICAL_SURFACE('',#14930,3.0735);
#13417=CYLINDRICAL_SURFACE('',#14931,3.0735);
#13418=CYLINDRICAL_SURFACE('',#14932,3.0735);
#13419=CYLINDRICAL_SURFACE('',#14933,3.0735);
#13420=CYLINDRICAL_SURFACE('',#14934,3.0735);
#13421=CYLINDRICAL_SURFACE('',#14935,3.0735);
#13422=CYLINDRICAL_SURFACE('',#14936,3.0735);
#13423=CYLINDRICAL_SURFACE('',#14938,2.5175);
#13424=CYLINDRICAL_SURFACE('',#14942,2.5175);
#13425=CYLINDRICAL_SURFACE('',#14943,2.5175);
#13426=CYLINDRICAL_SURFACE('',#14944,2.5175);
#13427=CYLINDRICAL_SURFACE('',#14945,2.5175);
#13428=CYLINDRICAL_SURFACE('',#14946,2.5175);
#13429=CYLINDRICAL_SURFACE('',#14947,2.5175);
#13430=CYLINDRICAL_SURFACE('',#14948,2.5175);
#13431=CYLINDRICAL_SURFACE('',#14949,2.5175);
#13432=CYLINDRICAL_SURFACE('',#14951,3.0735);
#13433=CYLINDRICAL_SURFACE('',#14953,3.0735);
#13434=CYLINDRICAL_SURFACE('',#14954,3.0735);
#13435=CYLINDRICAL_SURFACE('',#14955,3.0735);
#13436=CYLINDRICAL_SURFACE('',#14956,3.0735);
#13437=CYLINDRICAL_SURFACE('',#14957,3.0735);
#13438=CYLINDRICAL_SURFACE('',#14958,3.0735);
#13439=CYLINDRICAL_SURFACE('',#14959,3.0735);
#13440=CYLINDRICAL_SURFACE('',#14960,3.0735);
#13441=CYLINDRICAL_SURFACE('',#14962,2.5175);
#13442=CYLINDRICAL_SURFACE('',#14966,2.5175);
#13443=CYLINDRICAL_SURFACE('',#14967,2.5175);
#13444=CYLINDRICAL_SURFACE('',#14968,2.5175);
#13445=CYLINDRICAL_SURFACE('',#14969,2.5175);
#13446=CYLINDRICAL_SURFACE('',#14970,2.5175);
#13447=CYLINDRICAL_SURFACE('',#14971,2.5175);
#13448=CYLINDRICAL_SURFACE('',#14972,2.5175);
#13449=CYLINDRICAL_SURFACE('',#14973,2.5175);
#13450=CYLINDRICAL_SURFACE('',#14975,3.0735);
#13451=CYLINDRICAL_SURFACE('',#14977,3.0735);
#13452=CYLINDRICAL_SURFACE('',#14978,3.0735);
#13453=CYLINDRICAL_SURFACE('',#14979,3.0735);
#13454=CYLINDRICAL_SURFACE('',#14980,3.0735);
#13455=CYLINDRICAL_SURFACE('',#14981,3.0735);
#13456=CYLINDRICAL_SURFACE('',#14982,3.0735);
#13457=CYLINDRICAL_SURFACE('',#14983,3.0735);
#13458=CYLINDRICAL_SURFACE('',#14984,3.0735);
#13459=CYLINDRICAL_SURFACE('',#14986,2.5175);
#13460=CYLINDRICAL_SURFACE('',#14990,2.5175);
#13461=CYLINDRICAL_SURFACE('',#14991,2.5175);
#13462=CYLINDRICAL_SURFACE('',#14992,2.5175);
#13463=CYLINDRICAL_SURFACE('',#14993,2.5175);
#13464=CYLINDRICAL_SURFACE('',#14994,2.5175);
#13465=CYLINDRICAL_SURFACE('',#14995,2.5175);
#13466=CYLINDRICAL_SURFACE('',#14996,2.5175);
#13467=CYLINDRICAL_SURFACE('',#14997,2.5175);
#13468=CYLINDRICAL_SURFACE('',#14999,3.0735);
#13469=CYLINDRICAL_SURFACE('',#15001,3.0735);
#13470=CYLINDRICAL_SURFACE('',#15002,3.0735);
#13471=CYLINDRICAL_SURFACE('',#15003,3.0735);
#13472=CYLINDRICAL_SURFACE('',#15004,3.0735);
#13473=CYLINDRICAL_SURFACE('',#15005,3.0735);
#13474=CYLINDRICAL_SURFACE('',#15006,3.0735);
#13475=CYLINDRICAL_SURFACE('',#15007,3.0735);
#13476=CYLINDRICAL_SURFACE('',#15008,3.0735);
#13477=CYLINDRICAL_SURFACE('',#15010,2.5175);
#13478=CYLINDRICAL_SURFACE('',#15014,2.5175);
#13479=CYLINDRICAL_SURFACE('',#15015,2.5175);
#13480=CYLINDRICAL_SURFACE('',#15016,2.5175);
#13481=CYLINDRICAL_SURFACE('',#15017,2.5175);
#13482=CYLINDRICAL_SURFACE('',#15018,2.5175);
#13483=CYLINDRICAL_SURFACE('',#15019,2.5175);
#13484=CYLINDRICAL_SURFACE('',#15020,2.5175);
#13485=CYLINDRICAL_SURFACE('',#15021,2.5175);
#13486=CYLINDRICAL_SURFACE('',#15023,3.0735);
#13487=CYLINDRICAL_SURFACE('',#15025,3.0735);
#13488=CYLINDRICAL_SURFACE('',#15026,3.0735);
#13489=CYLINDRICAL_SURFACE('',#15027,3.0735);
#13490=CYLINDRICAL_SURFACE('',#15028,3.0735);
#13491=CYLINDRICAL_SURFACE('',#15029,3.0735);
#13492=CYLINDRICAL_SURFACE('',#15030,3.0735);
#13493=CYLINDRICAL_SURFACE('',#15031,3.0735);
#13494=CYLINDRICAL_SURFACE('',#15032,3.0735);
#13495=CYLINDRICAL_SURFACE('',#15034,2.5175);
#13496=CYLINDRICAL_SURFACE('',#15038,2.5175);
#13497=CYLINDRICAL_SURFACE('',#15039,2.5175);
#13498=CYLINDRICAL_SURFACE('',#15040,2.5175);
#13499=CYLINDRICAL_SURFACE('',#15041,2.5175);
#13500=CYLINDRICAL_SURFACE('',#15042,2.5175);
#13501=CYLINDRICAL_SURFACE('',#15043,2.5175);
#13502=CYLINDRICAL_SURFACE('',#15044,2.5175);
#13503=CYLINDRICAL_SURFACE('',#15045,2.5175);
#13504=CYLINDRICAL_SURFACE('',#15047,3.0735);
#13505=CYLINDRICAL_SURFACE('',#15049,3.0735);
#13506=CYLINDRICAL_SURFACE('',#15050,3.0735);
#13507=CYLINDRICAL_SURFACE('',#15051,3.0735);
#13508=CYLINDRICAL_SURFACE('',#15052,3.0735);
#13509=CYLINDRICAL_SURFACE('',#15053,3.0735);
#13510=CYLINDRICAL_SURFACE('',#15054,3.0735);
#13511=CYLINDRICAL_SURFACE('',#15055,3.0735);
#13512=CYLINDRICAL_SURFACE('',#15056,3.0735);
#13513=CYLINDRICAL_SURFACE('',#15058,7.);
#13514=CYLINDRICAL_SURFACE('',#15063,7.);
#13515=CYLINDRICAL_SURFACE('',#15068,7.);
#13516=CYLINDRICAL_SURFACE('',#15073,7.);
#13517=CYLINDRICAL_SURFACE('',#15078,4.5);
#13518=CYLINDRICAL_SURFACE('',#15080,4.5);
#13519=CYLINDRICAL_SURFACE('',#15082,4.5);
#13520=CYLINDRICAL_SURFACE('',#15084,4.5);
#13521=CYLINDRICAL_SURFACE('',#15087,3.0735);
#13522=CYLINDRICAL_SURFACE('',#15088,2.5175);
#13523=CYLINDRICAL_SURFACE('',#15090,3.0735);
#13524=CYLINDRICAL_SURFACE('',#15091,2.5175);
#13525=CYLINDRICAL_SURFACE('',#15093,3.0735);
#13526=CYLINDRICAL_SURFACE('',#15094,2.5175);
#13527=CYLINDRICAL_SURFACE('',#15096,3.0735);
#13528=CYLINDRICAL_SURFACE('',#15097,2.5175);
#13529=CYLINDRICAL_SURFACE('',#15099,3.0735);
#13530=CYLINDRICAL_SURFACE('',#15100,2.5175);
#13531=CYLINDRICAL_SURFACE('',#15102,3.0735);
#13532=CYLINDRICAL_SURFACE('',#15103,2.5175);
#13533=CYLINDRICAL_SURFACE('',#15105,3.0735);
#13534=CYLINDRICAL_SURFACE('',#15106,2.5175);
#13535=CYLINDRICAL_SURFACE('',#15108,3.0735);
#13536=CYLINDRICAL_SURFACE('',#15109,2.5175);
#13537=CYLINDRICAL_SURFACE('',#15143,20.);
#13538=CYLINDRICAL_SURFACE('',#15169,100.);
#13539=CYLINDRICAL_SURFACE('',#15188,40.);
#13950=ADVANCED_FACE('',(#522),#13369,.F.);
#13951=ADVANCED_FACE('',(#523),#13370,.F.);
#13952=ADVANCED_FACE('',(#524),#13371,.F.);
#13953=ADVANCED_FACE('',(#525),#13372,.F.);
#13954=ADVANCED_FACE('',(#526),#13373,.F.);
#13955=ADVANCED_FACE('',(#527),#13374,.F.);
#13956=ADVANCED_FACE('',(#528),#13375,.F.);
#13957=ADVANCED_FACE('',(#529),#13376,.F.);
#13958=ADVANCED_FACE('',(#530),#13377,.F.);
#13959=ADVANCED_FACE('',(#531),#13378,.F.);
#13960=ADVANCED_FACE('',(#532),#13379,.F.);
#13961=ADVANCED_FACE('',(#533),#13380,.F.);
#13962=ADVANCED_FACE('',(#534),#13381,.F.);
#13963=ADVANCED_FACE('',(#535),#13382,.F.);
#13964=ADVANCED_FACE('',(#536),#13383,.F.);
#13965=ADVANCED_FACE('',(#537),#13384,.F.);
#13966=ADVANCED_FACE('',(#538),#13385,.F.);
#13967=ADVANCED_FACE('',(#539),#13386,.F.);
#13968=ADVANCED_FACE('',(#540),#13387,.F.);
#13969=ADVANCED_FACE('',(#541),#13388,.F.);
#13970=ADVANCED_FACE('',(#542),#13389,.F.);
#13971=ADVANCED_FACE('',(#543),#13390,.F.);
#13972=ADVANCED_FACE('',(#544),#13391,.F.);
#13973=ADVANCED_FACE('',(#545),#13392,.F.);
#13974=ADVANCED_FACE('',(#546),#13393,.F.);
#13975=ADVANCED_FACE('',(#547),#13394,.F.);
#13976=ADVANCED_FACE('',(#548),#13395,.F.);
#13977=ADVANCED_FACE('',(#549),#13396,.F.);
#13978=ADVANCED_FACE('',(#550),#13397,.F.);
#13979=ADVANCED_FACE('',(#551),#13398,.F.);
#13980=ADVANCED_FACE('',(#552),#13399,.F.);
#13981=ADVANCED_FACE('',(#553),#13400,.F.);
#13982=ADVANCED_FACE('',(#554),#13401,.F.);
#13983=ADVANCED_FACE('',(#555),#13402,.F.);
#13984=ADVANCED_FACE('',(#556),#13403,.F.);
#13985=ADVANCED_FACE('',(#557),#13404,.F.);
#13986=ADVANCED_FACE('',(#558),#13405,.F.);
#13987=ADVANCED_FACE('',(#559),#13406,.F.);
#13988=ADVANCED_FACE('',(#560),#13407,.F.);
#13989=ADVANCED_FACE('',(#561),#13408,.F.);
#13990=ADVANCED_FACE('',(#562),#13409,.F.);
#13991=ADVANCED_FACE('',(#563),#13410,.F.);
#13992=ADVANCED_FACE('',(#564),#13411,.F.);
#13993=ADVANCED_FACE('',(#565),#13412,.F.);
#13994=ADVANCED_FACE('',(#566),#13413,.F.);
#13995=ADVANCED_FACE('',(#567),#13414,.F.);
#13996=ADVANCED_FACE('',(#568),#13415,.F.);
#13997=ADVANCED_FACE('',(#569),#13416,.F.);
#13998=ADVANCED_FACE('',(#570),#13417,.F.);
#13999=ADVANCED_FACE('',(#571),#13418,.F.);
#14000=ADVANCED_FACE('',(#572),#13419,.F.);
#14001=ADVANCED_FACE('',(#573),#13420,.F.);
#14002=ADVANCED_FACE('',(#574),#13421,.F.);
#14003=ADVANCED_FACE('',(#575),#13422,.F.);
#14004=ADVANCED_FACE('',(#576),#13423,.F.);
#14005=ADVANCED_FACE('',(#577),#13424,.F.);
#14006=ADVANCED_FACE('',(#578),#13425,.F.);
#14007=ADVANCED_FACE('',(#579),#13426,.F.);
#14008=ADVANCED_FACE('',(#580),#13427,.F.);
#14009=ADVANCED_FACE('',(#581),#13428,.F.);
#14010=ADVANCED_FACE('',(#582),#13429,.F.);
#14011=ADVANCED_FACE('',(#583),#13430,.F.);
#14012=ADVANCED_FACE('',(#584),#13431,.F.);
#14013=ADVANCED_FACE('',(#585),#13432,.F.);
#14014=ADVANCED_FACE('',(#586),#13433,.F.);
#14015=ADVANCED_FACE('',(#587),#13434,.F.);
#14016=ADVANCED_FACE('',(#588),#13435,.F.);
#14017=ADVANCED_FACE('',(#589),#13436,.F.);
#14018=ADVANCED_FACE('',(#590),#13437,.F.);
#14019=ADVANCED_FACE('',(#591),#13438,.F.);
#14020=ADVANCED_FACE('',(#592),#13439,.F.);
#14021=ADVANCED_FACE('',(#593),#13440,.F.);
#14022=ADVANCED_FACE('',(#594),#13441,.F.);
#14023=ADVANCED_FACE('',(#595),#13442,.F.);
#14024=ADVANCED_FACE('',(#596),#13443,.F.);
#14025=ADVANCED_FACE('',(#597),#13444,.F.);
#14026=ADVANCED_FACE('',(#598),#13445,.F.);
#14027=ADVANCED_FACE('',(#599),#13446,.F.);
#14028=ADVANCED_FACE('',(#600),#13447,.F.);
#14029=ADVANCED_FACE('',(#601),#13448,.F.);
#14030=ADVANCED_FACE('',(#602),#13449,.F.);
#14031=ADVANCED_FACE('',(#603),#13450,.F.);
#14032=ADVANCED_FACE('',(#604),#13451,.F.);
#14033=ADVANCED_FACE('',(#605),#13452,.F.);
#14034=ADVANCED_FACE('',(#606),#13453,.F.);
#14035=ADVANCED_FACE('',(#607),#13454,.F.);
#14036=ADVANCED_FACE('',(#608),#13455,.F.);
#14037=ADVANCED_FACE('',(#609),#13456,.F.);
#14038=ADVANCED_FACE('',(#610),#13457,.F.);
#14039=ADVANCED_FACE('',(#611),#13458,.F.);
#14040=ADVANCED_FACE('',(#612),#13459,.F.);
#14041=ADVANCED_FACE('',(#613),#13460,.F.);
#14042=ADVANCED_FACE('',(#614),#13461,.F.);
#14043=ADVANCED_FACE('',(#615),#13462,.F.);
#14044=ADVANCED_FACE('',(#616),#13463,.F.);
#14045=ADVANCED_FACE('',(#617),#13464,.F.);
#14046=ADVANCED_FACE('',(#618),#13465,.F.);
#14047=ADVANCED_FACE('',(#619),#13466,.F.);
#14048=ADVANCED_FACE('',(#620),#13467,.F.);
#14049=ADVANCED_FACE('',(#621),#13468,.F.);
#14050=ADVANCED_FACE('',(#622),#13469,.F.);
#14051=ADVANCED_FACE('',(#623),#13470,.F.);
#14052=ADVANCED_FACE('',(#624),#13471,.F.);
#14053=ADVANCED_FACE('',(#625),#13472,.F.);
#14054=ADVANCED_FACE('',(#626),#13473,.F.);
#14055=ADVANCED_FACE('',(#627),#13474,.F.);
#14056=ADVANCED_FACE('',(#628),#13475,.F.);
#14057=ADVANCED_FACE('',(#629),#13476,.F.);
#14058=ADVANCED_FACE('',(#630),#13477,.F.);
#14059=ADVANCED_FACE('',(#631),#13478,.F.);
#14060=ADVANCED_FACE('',(#632),#13479,.F.);
#14061=ADVANCED_FACE('',(#633),#13480,.F.);
#14062=ADVANCED_FACE('',(#634),#13481,.F.);
#14063=ADVANCED_FACE('',(#635),#13482,.F.);
#14064=ADVANCED_FACE('',(#636),#13483,.F.);
#14065=ADVANCED_FACE('',(#637),#13484,.F.);
#14066=ADVANCED_FACE('',(#638),#13485,.F.);
#14067=ADVANCED_FACE('',(#639),#13486,.F.);
#14068=ADVANCED_FACE('',(#640),#13487,.F.);
#14069=ADVANCED_FACE('',(#641),#13488,.F.);
#14070=ADVANCED_FACE('',(#642),#13489,.F.);
#14071=ADVANCED_FACE('',(#643),#13490,.F.);
#14072=ADVANCED_FACE('',(#644),#13491,.F.);
#14073=ADVANCED_FACE('',(#645),#13492,.F.);
#14074=ADVANCED_FACE('',(#646),#13493,.F.);
#14075=ADVANCED_FACE('',(#647),#13494,.F.);
#14076=ADVANCED_FACE('',(#648),#13495,.F.);
#14077=ADVANCED_FACE('',(#649),#13496,.F.);
#14078=ADVANCED_FACE('',(#650),#13497,.F.);
#14079=ADVANCED_FACE('',(#651),#13498,.F.);
#14080=ADVANCED_FACE('',(#652),#13499,.F.);
#14081=ADVANCED_FACE('',(#653),#13500,.F.);
#14082=ADVANCED_FACE('',(#654),#13501,.F.);
#14083=ADVANCED_FACE('',(#655),#13502,.F.);
#14084=ADVANCED_FACE('',(#656),#13503,.F.);
#14085=ADVANCED_FACE('',(#657),#13504,.F.);
#14086=ADVANCED_FACE('',(#658),#13505,.F.);
#14087=ADVANCED_FACE('',(#659),#13506,.F.);
#14088=ADVANCED_FACE('',(#660),#13507,.F.);
#14089=ADVANCED_FACE('',(#661),#13508,.F.);
#14090=ADVANCED_FACE('',(#662),#13509,.F.);
#14091=ADVANCED_FACE('',(#663),#13510,.F.);
#14092=ADVANCED_FACE('',(#664),#13511,.F.);
#14093=ADVANCED_FACE('',(#665),#13512,.F.);
#14094=ADVANCED_FACE('',(#666),#13513,.F.);
#14095=ADVANCED_FACE('',(#667,#298),#365,.F.);
#14096=ADVANCED_FACE('',(#668),#13514,.F.);
#14097=ADVANCED_FACE('',(#669,#299),#366,.F.);
#14098=ADVANCED_FACE('',(#670),#13515,.F.);
#14099=ADVANCED_FACE('',(#671,#300),#367,.F.);
#14100=ADVANCED_FACE('',(#672),#13516,.F.);
#14101=ADVANCED_FACE('',(#673,#301),#368,.F.);
#14102=ADVANCED_FACE('',(#674),#13517,.F.);
#14103=ADVANCED_FACE('',(#675),#13518,.F.);
#14104=ADVANCED_FACE('',(#676),#13519,.F.);
#14105=ADVANCED_FACE('',(#677),#13520,.F.);
#14106=ADVANCED_FACE('',(#678),#369,.T.);
#14107=ADVANCED_FACE('',(#679),#13521,.F.);
#14108=ADVANCED_FACE('',(#680),#258,.F.);
#14109=ADVANCED_FACE('',(#681),#259,.F.);
#14110=ADVANCED_FACE('',(#682),#13522,.F.);
#14111=ADVANCED_FACE('',(#683),#370,.T.);
#14112=ADVANCED_FACE('',(#684),#13523,.F.);
#14113=ADVANCED_FACE('',(#685),#260,.F.);
#14114=ADVANCED_FACE('',(#686),#261,.F.);
#14115=ADVANCED_FACE('',(#687),#13524,.F.);
#14116=ADVANCED_FACE('',(#688),#371,.T.);
#14117=ADVANCED_FACE('',(#689),#13525,.F.);
#14118=ADVANCED_FACE('',(#690),#262,.F.);
#14119=ADVANCED_FACE('',(#691),#263,.F.);
#14120=ADVANCED_FACE('',(#692),#13526,.F.);
#14121=ADVANCED_FACE('',(#693),#372,.T.);
#14122=ADVANCED_FACE('',(#694),#13527,.F.);
#14123=ADVANCED_FACE('',(#695),#264,.F.);
#14124=ADVANCED_FACE('',(#696),#265,.F.);
#14125=ADVANCED_FACE('',(#697),#13528,.F.);
#14126=ADVANCED_FACE('',(#698),#373,.T.);
#14127=ADVANCED_FACE('',(#699),#13529,.F.);
#14128=ADVANCED_FACE('',(#700),#266,.F.);
#14129=ADVANCED_FACE('',(#701),#267,.F.);
#14130=ADVANCED_FACE('',(#702),#13530,.F.);
#14131=ADVANCED_FACE('',(#703),#374,.T.);
#14132=ADVANCED_FACE('',(#704),#13531,.F.);
#14133=ADVANCED_FACE('',(#705),#268,.F.);
#14134=ADVANCED_FACE('',(#706),#269,.F.);
#14135=ADVANCED_FACE('',(#707),#13532,.F.);
#14136=ADVANCED_FACE('',(#708),#375,.T.);
#14137=ADVANCED_FACE('',(#709),#13533,.F.);
#14138=ADVANCED_FACE('',(#710),#270,.F.);
#14139=ADVANCED_FACE('',(#711),#271,.F.);
#14140=ADVANCED_FACE('',(#712),#13534,.F.);
#14141=ADVANCED_FACE('',(#713),#376,.T.);
#14142=ADVANCED_FACE('',(#714),#13535,.F.);
#14143=ADVANCED_FACE('',(#715),#272,.F.);
#14144=ADVANCED_FACE('',(#716),#273,.F.);
#14145=ADVANCED_FACE('',(#717),#13536,.F.);
#14146=ADVANCED_FACE('',(#718),#377,.F.);
#14147=ADVANCED_FACE('',(#719),#378,.F.);
#14148=ADVANCED_FACE('',(#720),#379,.F.);
#14149=ADVANCED_FACE('',(#721,#302,#303),#380,.F.);
#14150=ADVANCED_FACE('',(#722),#381,.F.);
#14151=ADVANCED_FACE('',(#723),#382,.F.);
#14152=ADVANCED_FACE('',(#724),#383,.F.);
#14153=ADVANCED_FACE('',(#725,#304,#305),#384,.F.);
#14154=ADVANCED_FACE('',(#726),#385,.F.);
#14155=ADVANCED_FACE('',(#727),#386,.F.);
#14156=ADVANCED_FACE('',(#728,#306),#387,.T.);
#14157=ADVANCED_FACE('',(#729,#307),#388,.T.);
#14158=ADVANCED_FACE('',(#730),#389,.F.);
#14159=ADVANCED_FACE('',(#731),#390,.F.);
#14160=ADVANCED_FACE('',(#732),#391,.F.);
#14161=ADVANCED_FACE('',(#733),#392,.F.);
#14162=ADVANCED_FACE('',(#734),#393,.F.);
#14163=ADVANCED_FACE('',(#735),#394,.F.);
#14164=ADVANCED_FACE('',(#736,#308),#395,.T.);
#14165=ADVANCED_FACE('',(#737),#396,.F.);
#14166=ADVANCED_FACE('',(#738),#397,.F.);
#14167=ADVANCED_FACE('',(#739),#398,.F.);
#14168=ADVANCED_FACE('',(#740),#399,.F.);
#14169=ADVANCED_FACE('',(#741),#13537,.F.);
#14170=ADVANCED_FACE('',(#742),#400,.F.);
#14171=ADVANCED_FACE('',(#743),#401,.F.);
#14172=ADVANCED_FACE('',(#744),#402,.F.);
#14173=ADVANCED_FACE('',(#745),#403,.F.);
#14174=ADVANCED_FACE('',(#746),#404,.F.);
#14175=ADVANCED_FACE('',(#747),#405,.F.);
#14176=ADVANCED_FACE('',(#748),#406,.F.);
#14177=ADVANCED_FACE('',(#749,#309,#310),#407,.F.);
#14178=ADVANCED_FACE('',(#750),#408,.F.);
#14179=ADVANCED_FACE('',(#751),#409,.F.);
#14180=ADVANCED_FACE('',(#752),#410,.F.);
#14181=ADVANCED_FACE('',(#753),#411,.F.);
#14182=ADVANCED_FACE('',(#754),#412,.F.);
#14183=ADVANCED_FACE('',(#755,#311,#312),#413,.F.);
#14184=ADVANCED_FACE('',(#756),#414,.F.);
#14185=ADVANCED_FACE('',(#757),#415,.F.);
#14186=ADVANCED_FACE('',(#758),#416,.F.);
#14187=ADVANCED_FACE('',(#759),#13538,.T.);
#14188=ADVANCED_FACE('',(#760),#417,.F.);
#14189=ADVANCED_FACE('',(#761),#418,.F.);
#14190=ADVANCED_FACE('',(#762,#313),#419,.T.);
#14191=ADVANCED_FACE('',(#763),#420,.F.);
#14192=ADVANCED_FACE('',(#764),#421,.F.);
#14193=ADVANCED_FACE('',(#765),#422,.F.);
#14194=ADVANCED_FACE('',(#766),#423,.F.);
#14195=ADVANCED_FACE('',(#767),#424,.F.);
#14196=ADVANCED_FACE('',(#768),#425,.F.);
#14197=ADVANCED_FACE('',(#769),#426,.F.);
#14198=ADVANCED_FACE('',(#770),#427,.F.);
#14199=ADVANCED_FACE('',(#771),#428,.F.);
#14200=ADVANCED_FACE('',(#772),#429,.F.);
#14201=ADVANCED_FACE('',(#773),#430,.F.);
#14202=ADVANCED_FACE('',(#774),#431,.F.);
#14203=ADVANCED_FACE('',(#775),#432,.F.);
#14204=ADVANCED_FACE('',(#776),#13539,.F.);
#14205=ADVANCED_FACE('',(#777,#314),#433,.F.);
#14206=ADVANCED_FACE('',(#778,#315,#316,#317,#318,#319,#320,#321,#322,#323,
#324,#325,#326,#327),#434,.F.);
#14731=CLOSED_SHELL('',(#13950,#13951,#13952,#13953,#13954,#13955,#13956,
#13957,#13958,#13959,#13960,#13961,#13962,#13963,#13964,#13965,#13966,#13967,
#13968,#13969,#13970,#13971,#13972,#13973,#13974,#13975,#13976,#13977,#13978,
#13979,#13980,#13981,#13982,#13983,#13984,#13985,#13986,#13987,#13988,#13989,
#13990,#13991,#13992,#13993,#13994,#13995,#13996,#13997,#13998,#13999,#14000,
#14001,#14002,#14003,#14004,#14005,#14006,#14007,#14008,#14009,#14010,#14011,
#14012,#14013,#14014,#14015,#14016,#14017,#14018,#14019,#14020,#14021,#14022,
#14023,#14024,#14025,#14026,#14027,#14028,#14029,#14030,#14031,#14032,#14033,
#14034,#14035,#14036,#14037,#14038,#14039,#14040,#14041,#14042,#14043,#14044,
#14045,#14046,#14047,#14048,#14049,#14050,#14051,#14052,#14053,#14054,#14055,
#14056,#14057,#14058,#14059,#14060,#14061,#14062,#14063,#14064,#14065,#14066,
#14067,#14068,#14069,#14070,#14071,#14072,#14073,#14074,#14075,#14076,#14077,
#14078,#14079,#14080,#14081,#14082,#14083,#14084,#14085,#14086,#14087,#14088,
#14089,#14090,#14091,#14092,#14093,#14094,#14095,#14096,#14097,#14098,#14099,
#14100,#14101,#14102,#14103,#14104,#14105,#14106,#14107,#14108,#14109,#14110,
#14111,#14112,#14113,#14114,#14115,#14116,#14117,#14118,#14119,#14120,#14121,
#14122,#14123,#14124,#14125,#14126,#14127,#14128,#14129,#14130,#14131,#14132,
#14133,#14134,#14135,#14136,#14137,#14138,#14139,#14140,#14141,#14142,#14143,
#14144,#14145,#14146,#14147,#14148,#14149,#14150,#14151,#14152,#14153,#14154,
#14155,#14156,#14157,#14158,#14159,#14160,#14161,#14162,#14163,#14164,#14165,
#14166,#14167,#14168,#14169,#14170,#14171,#14172,#14173,#14174,#14175,#14176,
#14177,#14178,#14179,#14180,#14181,#14182,#14183,#14184,#14185,#14186,#14187,
#14188,#14189,#14190,#14191,#14192,#14193,#14194,#14195,#14196,#14197,#14198,
#14199,#14200,#14201,#14202,#14203,#14204,#14205,#14206));
#14865=AXIS2_PLACEMENT_3D('',#18710,#15865,#15866);
#14866=AXIS2_PLACEMENT_3D('',#18711,#15867,#15868);
#14867=AXIS2_PLACEMENT_3D('',#18721,#15870,#15871);
#14868=AXIS2_PLACEMENT_3D('',#18724,#15873,#15874);
#14869=AXIS2_PLACEMENT_3D('',#18726,#15875,#15876);
#14870=AXIS2_PLACEMENT_3D('',#18737,#15877,#15878);
#14871=AXIS2_PLACEMENT_3D('',#18788,#15880,#15881);
#14872=AXIS2_PLACEMENT_3D('',#18839,#15883,#15884);
#14873=AXIS2_PLACEMENT_3D('',#18887,#15886,#15887);
#14874=AXIS2_PLACEMENT_3D('',#18938,#15889,#15890);
#14875=AXIS2_PLACEMENT_3D('',#18989,#15892,#15893);
#14876=AXIS2_PLACEMENT_3D('',#19037,#15895,#15896);
#14877=AXIS2_PLACEMENT_3D('',#19088,#15898,#15899);
#14878=AXIS2_PLACEMENT_3D('',#19107,#15901,#15902);
#14879=AXIS2_PLACEMENT_3D('',#19127,#15903,#15904);
#14880=AXIS2_PLACEMENT_3D('',#19141,#15906,#15907);
#14881=AXIS2_PLACEMENT_3D('',#19151,#15908,#15909);
#14882=AXIS2_PLACEMENT_3D('',#19175,#15911,#15912);
#14883=AXIS2_PLACEMENT_3D('',#19200,#15914,#15915);
#14884=AXIS2_PLACEMENT_3D('',#19225,#15917,#15918);
#14885=AXIS2_PLACEMENT_3D('',#19249,#15920,#15921);
#14886=AXIS2_PLACEMENT_3D('',#19274,#15923,#15924);
#14887=AXIS2_PLACEMENT_3D('',#19299,#15926,#15927);
#14888=AXIS2_PLACEMENT_3D('',#19323,#15929,#15930);
#14889=AXIS2_PLACEMENT_3D('',#19334,#15932,#15933);
#14890=AXIS2_PLACEMENT_3D('',#19340,#15934,#15935);
#14891=AXIS2_PLACEMENT_3D('',#19350,#15937,#15938);
#14892=AXIS2_PLACEMENT_3D('',#19353,#15940,#15941);
#14893=AXIS2_PLACEMENT_3D('',#19355,#15942,#15943);
#14894=AXIS2_PLACEMENT_3D('',#19366,#15944,#15945);
#14895=AXIS2_PLACEMENT_3D('',#19417,#15947,#15948);
#14896=AXIS2_PLACEMENT_3D('',#19468,#15950,#15951);
#14897=AXIS2_PLACEMENT_3D('',#19516,#15953,#15954);
#14898=AXIS2_PLACEMENT_3D('',#19567,#15956,#15957);
#14899=AXIS2_PLACEMENT_3D('',#19618,#15959,#15960);
#14900=AXIS2_PLACEMENT_3D('',#19666,#15962,#15963);
#14901=AXIS2_PLACEMENT_3D('',#19717,#15965,#15966);
#14902=AXIS2_PLACEMENT_3D('',#19736,#15968,#15969);
#14903=AXIS2_PLACEMENT_3D('',#19756,#15970,#15971);
#14904=AXIS2_PLACEMENT_3D('',#19770,#15973,#15974);
#14905=AXIS2_PLACEMENT_3D('',#19780,#15975,#15976);
#14906=AXIS2_PLACEMENT_3D('',#19804,#15978,#15979);
#14907=AXIS2_PLACEMENT_3D('',#19829,#15981,#15982);
#14908=AXIS2_PLACEMENT_3D('',#19854,#15984,#15985);
#14909=AXIS2_PLACEMENT_3D('',#19878,#15987,#15988);
#14910=AXIS2_PLACEMENT_3D('',#19903,#15990,#15991);
#14911=AXIS2_PLACEMENT_3D('',#19928,#15993,#15994);
#14912=AXIS2_PLACEMENT_3D('',#19952,#15996,#15997);
#14913=AXIS2_PLACEMENT_3D('',#19963,#15999,#16000);
#14914=AXIS2_PLACEMENT_3D('',#19969,#16001,#16002);
#14915=AXIS2_PLACEMENT_3D('',#19979,#16004,#16005);
#14916=AXIS2_PLACEMENT_3D('',#19982,#16007,#16008);
#14917=AXIS2_PLACEMENT_3D('',#19984,#16009,#16010);
#14918=AXIS2_PLACEMENT_3D('',#19995,#16011,#16012);
#14919=AXIS2_PLACEMENT_3D('',#20046,#16014,#16015);
#14920=AXIS2_PLACEMENT_3D('',#20097,#16017,#16018);
#14921=AXIS2_PLACEMENT_3D('',#20145,#16020,#16021);
#14922=AXIS2_PLACEMENT_3D('',#20196,#16023,#16024);
#14923=AXIS2_PLACEMENT_3D('',#20247,#16026,#16027);
#14924=AXIS2_PLACEMENT_3D('',#20295,#16029,#16030);
#14925=AXIS2_PLACEMENT_3D('',#20346,#16032,#16033);
#14926=AXIS2_PLACEMENT_3D('',#20365,#16035,#16036);
#14927=AXIS2_PLACEMENT_3D('',#20385,#16037,#16038);
#14928=AXIS2_PLACEMENT_3D('',#20399,#16040,#16041);
#14929=AXIS2_PLACEMENT_3D('',#20409,#16042,#16043);
#14930=AXIS2_PLACEMENT_3D('',#20433,#16045,#16046);
#14931=AXIS2_PLACEMENT_3D('',#20458,#16048,#16049);
#14932=AXIS2_PLACEMENT_3D('',#20483,#16051,#16052);
#14933=AXIS2_PLACEMENT_3D('',#20507,#16054,#16055);
#14934=AXIS2_PLACEMENT_3D('',#20532,#16057,#16058);
#14935=AXIS2_PLACEMENT_3D('',#20557,#16060,#16061);
#14936=AXIS2_PLACEMENT_3D('',#20581,#16063,#16064);
#14937=AXIS2_PLACEMENT_3D('',#20592,#16066,#16067);
#14938=AXIS2_PLACEMENT_3D('',#20598,#16068,#16069);
#14939=AXIS2_PLACEMENT_3D('',#20608,#16071,#16072);
#14940=AXIS2_PLACEMENT_3D('',#20611,#16074,#16075);
#14941=AXIS2_PLACEMENT_3D('',#20613,#16076,#16077);
#14942=AXIS2_PLACEMENT_3D('',#20624,#16078,#16079);
#14943=AXIS2_PLACEMENT_3D('',#20675,#16081,#16082);
#14944=AXIS2_PLACEMENT_3D('',#20726,#16084,#16085);
#14945=AXIS2_PLACEMENT_3D('',#20774,#16087,#16088);
#14946=AXIS2_PLACEMENT_3D('',#20825,#16090,#16091);
#14947=AXIS2_PLACEMENT_3D('',#20876,#16093,#16094);
#14948=AXIS2_PLACEMENT_3D('',#20924,#16096,#16097);
#14949=AXIS2_PLACEMENT_3D('',#20975,#16099,#16100);
#14950=AXIS2_PLACEMENT_3D('',#20994,#16102,#16103);
#14951=AXIS2_PLACEMENT_3D('',#21014,#16104,#16105);
#14952=AXIS2_PLACEMENT_3D('',#21028,#16107,#16108);
#14953=AXIS2_PLACEMENT_3D('',#21038,#16109,#16110);
#14954=AXIS2_PLACEMENT_3D('',#21062,#16112,#16113);
#14955=AXIS2_PLACEMENT_3D('',#21087,#16115,#16116);
#14956=AXIS2_PLACEMENT_3D('',#21112,#16118,#16119);
#14957=AXIS2_PLACEMENT_3D('',#21136,#16121,#16122);
#14958=AXIS2_PLACEMENT_3D('',#21161,#16124,#16125);
#14959=AXIS2_PLACEMENT_3D('',#21186,#16127,#16128);
#14960=AXIS2_PLACEMENT_3D('',#21210,#16130,#16131);
#14961=AXIS2_PLACEMENT_3D('',#21221,#16133,#16134);
#14962=AXIS2_PLACEMENT_3D('',#21227,#16135,#16136);
#14963=AXIS2_PLACEMENT_3D('',#21237,#16138,#16139);
#14964=AXIS2_PLACEMENT_3D('',#21240,#16141,#16142);
#14965=AXIS2_PLACEMENT_3D('',#21242,#16143,#16144);
#14966=AXIS2_PLACEMENT_3D('',#21253,#16145,#16146);
#14967=AXIS2_PLACEMENT_3D('',#21304,#16148,#16149);
#14968=AXIS2_PLACEMENT_3D('',#21355,#16151,#16152);
#14969=AXIS2_PLACEMENT_3D('',#21403,#16154,#16155);
#14970=AXIS2_PLACEMENT_3D('',#21454,#16157,#16158);
#14971=AXIS2_PLACEMENT_3D('',#21505,#16160,#16161);
#14972=AXIS2_PLACEMENT_3D('',#21553,#16163,#16164);
#14973=AXIS2_PLACEMENT_3D('',#21604,#16166,#16167);
#14974=AXIS2_PLACEMENT_3D('',#21623,#16169,#16170);
#14975=AXIS2_PLACEMENT_3D('',#21643,#16171,#16172);
#14976=AXIS2_PLACEMENT_3D('',#21657,#16174,#16175);
#14977=AXIS2_PLACEMENT_3D('',#21667,#16176,#16177);
#14978=AXIS2_PLACEMENT_3D('',#21691,#16179,#16180);
#14979=AXIS2_PLACEMENT_3D('',#21716,#16182,#16183);
#14980=AXIS2_PLACEMENT_3D('',#21741,#16185,#16186);
#14981=AXIS2_PLACEMENT_3D('',#21765,#16188,#16189);
#14982=AXIS2_PLACEMENT_3D('',#21790,#16191,#16192);
#14983=AXIS2_PLACEMENT_3D('',#21815,#16194,#16195);
#14984=AXIS2_PLACEMENT_3D('',#21839,#16197,#16198);
#14985=AXIS2_PLACEMENT_3D('',#21850,#16200,#16201);
#14986=AXIS2_PLACEMENT_3D('',#21856,#16202,#16203);
#14987=AXIS2_PLACEMENT_3D('',#21866,#16205,#16206);
#14988=AXIS2_PLACEMENT_3D('',#21869,#16208,#16209);
#14989=AXIS2_PLACEMENT_3D('',#21871,#16210,#16211);
#14990=AXIS2_PLACEMENT_3D('',#21882,#16212,#16213);
#14991=AXIS2_PLACEMENT_3D('',#21933,#16215,#16216);
#14992=AXIS2_PLACEMENT_3D('',#21984,#16218,#16219);
#14993=AXIS2_PLACEMENT_3D('',#22032,#16221,#16222);
#14994=AXIS2_PLACEMENT_3D('',#22083,#16224,#16225);
#14995=AXIS2_PLACEMENT_3D('',#22134,#16227,#16228);
#14996=AXIS2_PLACEMENT_3D('',#22182,#16230,#16231);
#14997=AXIS2_PLACEMENT_3D('',#22233,#16233,#16234);
#14998=AXIS2_PLACEMENT_3D('',#22252,#16236,#16237);
#14999=AXIS2_PLACEMENT_3D('',#22272,#16238,#16239);
#15000=AXIS2_PLACEMENT_3D('',#22286,#16241,#16242);
#15001=AXIS2_PLACEMENT_3D('',#22296,#16243,#16244);
#15002=AXIS2_PLACEMENT_3D('',#22320,#16246,#16247);
#15003=AXIS2_PLACEMENT_3D('',#22345,#16249,#16250);
#15004=AXIS2_PLACEMENT_3D('',#22370,#16252,#16253);
#15005=AXIS2_PLACEMENT_3D('',#22394,#16255,#16256);
#15006=AXIS2_PLACEMENT_3D('',#22419,#16258,#16259);
#15007=AXIS2_PLACEMENT_3D('',#22444,#16261,#16262);
#15008=AXIS2_PLACEMENT_3D('',#22468,#16264,#16265);
#15009=AXIS2_PLACEMENT_3D('',#22479,#16267,#16268);
#15010=AXIS2_PLACEMENT_3D('',#22485,#16269,#16270);
#15011=AXIS2_PLACEMENT_3D('',#22495,#16272,#16273);
#15012=AXIS2_PLACEMENT_3D('',#22498,#16275,#16276);
#15013=AXIS2_PLACEMENT_3D('',#22500,#16277,#16278);
#15014=AXIS2_PLACEMENT_3D('',#22511,#16279,#16280);
#15015=AXIS2_PLACEMENT_3D('',#22562,#16282,#16283);
#15016=AXIS2_PLACEMENT_3D('',#22613,#16285,#16286);
#15017=AXIS2_PLACEMENT_3D('',#22661,#16288,#16289);
#15018=AXIS2_PLACEMENT_3D('',#22712,#16291,#16292);
#15019=AXIS2_PLACEMENT_3D('',#22763,#16294,#16295);
#15020=AXIS2_PLACEMENT_3D('',#22811,#16297,#16298);
#15021=AXIS2_PLACEMENT_3D('',#22862,#16300,#16301);
#15022=AXIS2_PLACEMENT_3D('',#22881,#16303,#16304);
#15023=AXIS2_PLACEMENT_3D('',#22901,#16305,#16306);
#15024=AXIS2_PLACEMENT_3D('',#22915,#16308,#16309);
#15025=AXIS2_PLACEMENT_3D('',#22925,#16310,#16311);
#15026=AXIS2_PLACEMENT_3D('',#22949,#16313,#16314);
#15027=AXIS2_PLACEMENT_3D('',#22974,#16316,#16317);
#15028=AXIS2_PLACEMENT_3D('',#22999,#16319,#16320);
#15029=AXIS2_PLACEMENT_3D('',#23023,#16322,#16323);
#15030=AXIS2_PLACEMENT_3D('',#23048,#16325,#16326);
#15031=AXIS2_PLACEMENT_3D('',#23073,#16328,#16329);
#15032=AXIS2_PLACEMENT_3D('',#23097,#16331,#16332);
#15033=AXIS2_PLACEMENT_3D('',#23108,#16334,#16335);
#15034=AXIS2_PLACEMENT_3D('',#23114,#16336,#16337);
#15035=AXIS2_PLACEMENT_3D('',#23124,#16339,#16340);
#15036=AXIS2_PLACEMENT_3D('',#23127,#16342,#16343);
#15037=AXIS2_PLACEMENT_3D('',#23129,#16344,#16345);
#15038=AXIS2_PLACEMENT_3D('',#23140,#16346,#16347);
#15039=AXIS2_PLACEMENT_3D('',#23191,#16349,#16350);
#15040=AXIS2_PLACEMENT_3D('',#23242,#16352,#16353);
#15041=AXIS2_PLACEMENT_3D('',#23290,#16355,#16356);
#15042=AXIS2_PLACEMENT_3D('',#23341,#16358,#16359);
#15043=AXIS2_PLACEMENT_3D('',#23392,#16361,#16362);
#15044=AXIS2_PLACEMENT_3D('',#23440,#16364,#16365);
#15045=AXIS2_PLACEMENT_3D('',#23491,#16367,#16368);
#15046=AXIS2_PLACEMENT_3D('',#23510,#16370,#16371);
#15047=AXIS2_PLACEMENT_3D('',#23530,#16372,#16373);
#15048=AXIS2_PLACEMENT_3D('',#23544,#16375,#16376);
#15049=AXIS2_PLACEMENT_3D('',#23554,#16377,#16378);
#15050=AXIS2_PLACEMENT_3D('',#23578,#16380,#16381);
#15051=AXIS2_PLACEMENT_3D('',#23603,#16383,#16384);
#15052=AXIS2_PLACEMENT_3D('',#23628,#16386,#16387);
#15053=AXIS2_PLACEMENT_3D('',#23652,#16389,#16390);
#15054=AXIS2_PLACEMENT_3D('',#23677,#16392,#16393);
#15055=AXIS2_PLACEMENT_3D('',#23702,#16395,#16396);
#15056=AXIS2_PLACEMENT_3D('',#23726,#16398,#16399);
#15057=AXIS2_PLACEMENT_3D('',#23737,#16401,#16402);
#15058=AXIS2_PLACEMENT_3D('',#23743,#16403,#16404);
#15059=AXIS2_PLACEMENT_3D('',#23745,#16405,#16406);
#15060=AXIS2_PLACEMENT_3D('',#23748,#16408,#16409);
#15061=AXIS2_PLACEMENT_3D('',#23749,#16410,#16411);
#15062=AXIS2_PLACEMENT_3D('',#23751,#16412,#16413);
#15063=AXIS2_PLACEMENT_3D('',#23752,#16414,#16415);
#15064=AXIS2_PLACEMENT_3D('',#23754,#16416,#16417);
#15065=AXIS2_PLACEMENT_3D('',#23757,#16419,#16420);
#15066=AXIS2_PLACEMENT_3D('',#23758,#16421,#16422);
#15067=AXIS2_PLACEMENT_3D('',#23760,#16423,#16424);
#15068=AXIS2_PLACEMENT_3D('',#23761,#16425,#16426);
#15069=AXIS2_PLACEMENT_3D('',#23763,#16427,#16428);
#15070=AXIS2_PLACEMENT_3D('',#23766,#16430,#16431);
#15071=AXIS2_PLACEMENT_3D('',#23767,#16432,#16433);
#15072=AXIS2_PLACEMENT_3D('',#23769,#16434,#16435);
#15073=AXIS2_PLACEMENT_3D('',#23770,#16436,#16437);
#15074=AXIS2_PLACEMENT_3D('',#23772,#16438,#16439);
#15075=AXIS2_PLACEMENT_3D('',#23775,#16441,#16442);
#15076=AXIS2_PLACEMENT_3D('',#23776,#16443,#16444);
#15077=AXIS2_PLACEMENT_3D('',#23778,#16445,#16446);
#15078=AXIS2_PLACEMENT_3D('',#23779,#16447,#16448);
#15079=AXIS2_PLACEMENT_3D('',#23782,#16450,#16451);
#15080=AXIS2_PLACEMENT_3D('',#23783,#16452,#16453);
#15081=AXIS2_PLACEMENT_3D('',#23786,#16455,#16456);
#15082=AXIS2_PLACEMENT_3D('',#23787,#16457,#16458);
#15083=AXIS2_PLACEMENT_3D('',#23790,#16460,#16461);
#15084=AXIS2_PLACEMENT_3D('',#23791,#16462,#16463);
#15085=AXIS2_PLACEMENT_3D('',#23794,#16465,#16466);
#15086=AXIS2_PLACEMENT_3D('',#23795,#16467,#16468);
#15087=AXIS2_PLACEMENT_3D('',#23984,#16469,#16470);
#15088=AXIS2_PLACEMENT_3D('',#24731,#16471,#16472);
#15089=AXIS2_PLACEMENT_3D('',#24732,#16473,#16474);
#15090=AXIS2_PLACEMENT_3D('',#24921,#16475,#16476);
#15091=AXIS2_PLACEMENT_3D('',#25668,#16477,#16478);
#15092=AXIS2_PLACEMENT_3D('',#25669,#16479,#16480);
#15093=AXIS2_PLACEMENT_3D('',#25858,#16481,#16482);
#15094=AXIS2_PLACEMENT_3D('',#26605,#16483,#16484);
#15095=AXIS2_PLACEMENT_3D('',#26606,#16485,#16486);
#15096=AXIS2_PLACEMENT_3D('',#26795,#16487,#16488);
#15097=AXIS2_PLACEMENT_3D('',#27542,#16489,#16490);
#15098=AXIS2_PLACEMENT_3D('',#27543,#16491,#16492);
#15099=AXIS2_PLACEMENT_3D('',#27732,#16493,#16494);
#15100=AXIS2_PLACEMENT_3D('',#28479,#16495,#16496);
#15101=AXIS2_PLACEMENT_3D('',#28480,#16497,#16498);
#15102=AXIS2_PLACEMENT_3D('',#28669,#16499,#16500);
#15103=AXIS2_PLACEMENT_3D('',#29416,#16501,#16502);
#15104=AXIS2_PLACEMENT_3D('',#29417,#16503,#16504);
#15105=AXIS2_PLACEMENT_3D('',#29606,#16505,#16506);
#15106=AXIS2_PLACEMENT_3D('',#30353,#16507,#16508);
#15107=AXIS2_PLACEMENT_3D('',#30354,#16509,#16510);
#15108=AXIS2_PLACEMENT_3D('',#30543,#16511,#16512);
#15109=AXIS2_PLACEMENT_3D('',#31290,#16513,#16514);
#15110=AXIS2_PLACEMENT_3D('',#31291,#16515,#16516);
#15111=AXIS2_PLACEMENT_3D('',#31300,#16521,#16522);
#15112=AXIS2_PLACEMENT_3D('',#31322,#16534,#16535);
#15113=AXIS2_PLACEMENT_3D('',#31328,#16539,#16540);
#15114=AXIS2_PLACEMENT_3D('',#31329,#16541,#16542);
#15115=AXIS2_PLACEMENT_3D('',#31330,#16543,#16544);
#15116=AXIS2_PLACEMENT_3D('',#31355,#16557,#16558);
#15117=AXIS2_PLACEMENT_3D('',#31361,#16562,#16563);
#15118=AXIS2_PLACEMENT_3D('',#31367,#16567,#16568);
#15119=AXIS2_PLACEMENT_3D('',#31368,#16569,#16570);
#15120=AXIS2_PLACEMENT_3D('',#31369,#16571,#16572);
#15121=AXIS2_PLACEMENT_3D('',#31375,#16575,#16576);
#15122=AXIS2_PLACEMENT_3D('',#31379,#16579,#16580);
#15123=AXIS2_PLACEMENT_3D('',#31383,#16583,#16584);
#15124=AXIS2_PLACEMENT_3D('',#31385,#16585,#16586);
#15125=AXIS2_PLACEMENT_3D('',#31395,#16591,#16592);
#15126=AXIS2_PLACEMENT_3D('',#31399,#16595,#16596);
#15127=AXIS2_PLACEMENT_3D('',#31405,#16599,#16600);
#15128=AXIS2_PLACEMENT_3D('',#31414,#16605,#16606);
#15129=AXIS2_PLACEMENT_3D('',#31415,#16607,#16608);
#15130=AXIS2_PLACEMENT_3D('',#31419,#16611,#16612);
#15131=AXIS2_PLACEMENT_3D('',#31421,#16614,#16615);
#15132=AXIS2_PLACEMENT_3D('',#31427,#16618,#16619);
#15133=AXIS2_PLACEMENT_3D('',#31431,#16622,#16623);
#15134=AXIS2_PLACEMENT_3D('',#31435,#16626,#16627);
#15135=AXIS2_PLACEMENT_3D('',#31439,#16630,#16631);
#15136=AXIS2_PLACEMENT_3D('',#31443,#16634,#16635);
#15137=AXIS2_PLACEMENT_3D('',#31445,#16636,#16637);
#15138=AXIS2_PLACEMENT_3D('',#31455,#16642,#16643);
#15139=AXIS2_PLACEMENT_3D('',#31457,#16645,#16646);
#15140=AXIS2_PLACEMENT_3D('',#31461,#16649,#16650);
#15141=AXIS2_PLACEMENT_3D('',#31465,#16653,#16654);
#15142=AXIS2_PLACEMENT_3D('',#31471,#16658,#16659);
#15143=AXIS2_PLACEMENT_3D('',#31473,#16661,#16662);
#15144=AXIS2_PLACEMENT_3D('',#31479,#16666,#16667);
#15145=AXIS2_PLACEMENT_3D('',#31483,#16669,#16670);
#15146=AXIS2_PLACEMENT_3D('',#31489,#16674,#16675);
#15147=AXIS2_PLACEMENT_3D('',#31492,#16677,#16678);
#15148=AXIS2_PLACEMENT_3D('',#31494,#16679,#16680);
#15149=AXIS2_PLACEMENT_3D('',#31496,#16682,#16683);
#15150=AXIS2_PLACEMENT_3D('',#31499,#16686,#16687);
#15151=AXIS2_PLACEMENT_3D('',#31501,#16689,#16690);
#15152=AXIS2_PLACEMENT_3D('',#31502,#16691,#16692);
#15153=AXIS2_PLACEMENT_3D('',#31504,#16694,#16695);
#15154=AXIS2_PLACEMENT_3D('',#31509,#16699,#16700);
#15155=AXIS2_PLACEMENT_3D('',#31511,#16702,#16703);
#15156=AXIS2_PLACEMENT_3D('',#31517,#16707,#16708);
#15157=AXIS2_PLACEMENT_3D('',#31519,#16709,#16710);
#15158=AXIS2_PLACEMENT_3D('',#31524,#16713,#16714);
#15159=AXIS2_PLACEMENT_3D('',#31525,#16715,#16716);
#15160=AXIS2_PLACEMENT_3D('',#31540,#16725,#16726);
#15161=AXIS2_PLACEMENT_3D('',#31542,#16728,#16729);
#15162=AXIS2_PLACEMENT_3D('',#31548,#16733,#16734);
#15163=AXIS2_PLACEMENT_3D('',#31568,#16745,#16746);
#15164=AXIS2_PLACEMENT_3D('',#31574,#16750,#16751);
#15165=AXIS2_PLACEMENT_3D('',#31575,#16752,#16753);
#15166=AXIS2_PLACEMENT_3D('',#31576,#16754,#16755);
#15167=AXIS2_PLACEMENT_3D('',#31579,#16758,#16759);
#15168=AXIS2_PLACEMENT_3D('',#31583,#16762,#16763);
#15169=AXIS2_PLACEMENT_3D('',#31585,#16765,#16766);
#15170=AXIS2_PLACEMENT_3D('',#31588,#16768,#16769);
#15171=AXIS2_PLACEMENT_3D('',#31589,#16770,#16771);
#15172=AXIS2_PLACEMENT_3D('',#31590,#16772,#16773);
#15173=AXIS2_PLACEMENT_3D('',#31594,#16776,#16777);
#15174=AXIS2_PLACEMENT_3D('',#31597,#16780,#16781);
#15175=AXIS2_PLACEMENT_3D('',#31601,#16784,#16785);
#15176=AXIS2_PLACEMENT_3D('',#31603,#16787,#16788);
#15177=AXIS2_PLACEMENT_3D('',#31607,#16792,#16793);
#15178=AXIS2_PLACEMENT_3D('',#31609,#16795,#16796);
#15179=AXIS2_PLACEMENT_3D('',#31613,#16800,#16801);
#15180=AXIS2_PLACEMENT_3D('',#31618,#16805,#16806);
#15181=AXIS2_PLACEMENT_3D('',#31619,#16807,#16808);
#15182=AXIS2_PLACEMENT_3D('',#31623,#16811,#16812);
#15183=AXIS2_PLACEMENT_3D('',#31624,#16813,#16814);
#15184=AXIS2_PLACEMENT_3D('',#31626,#16816,#16817);
#15185=AXIS2_PLACEMENT_3D('',#31627,#16818,#16819);
#15186=AXIS2_PLACEMENT_3D('',#31628,#16820,#16821);
#15187=AXIS2_PLACEMENT_3D('',#31630,#16823,#16824);
#15188=AXIS2_PLACEMENT_3D('',#31631,#16825,#16826);
#15189=AXIS2_PLACEMENT_3D('',#31633,#16827,#16828);
#15190=AXIS2_PLACEMENT_3D('',#31636,#16830,#16831);
#15191=AXIS2_PLACEMENT_3D('',#31637,#16832,#16833);
#15192=AXIS2_PLACEMENT_3D('',#31638,#16834,#16835);
#15865=DIRECTION('axis',(0.,0.,1.));
#15866=DIRECTION('refdir',(1.,0.,0.));
#15867=DIRECTION('center_axis',(0.,0.,-1.));
#15868=DIRECTION('ref_axis',(1.,0.,0.));
#15869=DIRECTION('',(0.,0.,-1.));
#15870=DIRECTION('center_axis',(0.,0.,1.));
#15871=DIRECTION('ref_axis',(1.,0.,0.));
#15872=DIRECTION('',(0.,0.,-1.));
#15873=DIRECTION('center_axis',(0.,0.,-1.));
#15874=DIRECTION('ref_axis',(1.,0.,0.));
#15875=DIRECTION('center_axis',(0.,0.,1.));
#15876=DIRECTION('ref_axis',(1.,0.,0.));
#15877=DIRECTION('center_axis',(0.,0.,-1.));
#15878=DIRECTION('ref_axis',(1.,0.,0.));
#15879=DIRECTION('',(0.,0.,-1.));
#15880=DIRECTION('center_axis',(0.,0.,-1.));
#15881=DIRECTION('ref_axis',(1.,0.,0.));
#15882=DIRECTION('',(0.,0.,-1.));
#15883=DIRECTION('center_axis',(0.,0.,-1.));
#15884=DIRECTION('ref_axis',(1.,0.,0.));
#15885=DIRECTION('',(0.,0.,-1.));
#15886=DIRECTION('center_axis',(0.,0.,-1.));
#15887=DIRECTION('ref_axis',(1.,0.,0.));
#15888=DIRECTION('',(0.,0.,-1.));
#15889=DIRECTION('center_axis',(0.,0.,-1.));
#15890=DIRECTION('ref_axis',(1.,0.,0.));
#15891=DIRECTION('',(0.,0.,-1.));
#15892=DIRECTION('center_axis',(0.,0.,-1.));
#15893=DIRECTION('ref_axis',(1.,0.,0.));
#15894=DIRECTION('',(0.,0.,-1.));
#15895=DIRECTION('center_axis',(0.,0.,-1.));
#15896=DIRECTION('ref_axis',(1.,0.,0.));
#15897=DIRECTION('',(0.,0.,-1.));
#15898=DIRECTION('center_axis',(0.,0.,-1.));
#15899=DIRECTION('ref_axis',(0.938009665675859,-0.346609098407217,0.));
#15900=DIRECTION('',(0.,0.,-1.));
#15901=DIRECTION('center_axis',(0.,0.,1.));
#15902=DIRECTION('ref_axis',(1.,0.,0.));
#15903=DIRECTION('center_axis',(0.,0.,-1.));
#15904=DIRECTION('ref_axis',(1.,-3.61224345087086E-14,0.));
#15905=DIRECTION('',(1.22464679914735E-16,-4.4387199776766E-30,-1.));
#15906=DIRECTION('center_axis',(0.,0.,1.));
#15907=DIRECTION('ref_axis',(1.,-3.61224345087086E-14,0.));
#15908=DIRECTION('center_axis',(0.,0.,-1.));
#15909=DIRECTION('ref_axis',(1.,-3.61224345087086E-14,0.));
#15910=DIRECTION('',(1.22464679914735E-16,-4.4387199776766E-30,-1.));
#15911=DIRECTION('center_axis',(0.,0.,-1.));
#15912=DIRECTION('ref_axis',(1.,-3.61224345087086E-14,0.));
#15913=DIRECTION('',(1.22464679914735E-16,-4.4387199776766E-30,-1.));
#15914=DIRECTION('center_axis',(0.,0.,-1.));
#15915=DIRECTION('ref_axis',(1.,-3.61224345087086E-14,0.));
#15916=DIRECTION('',(1.22464679914735E-16,-4.4387199776766E-30,-1.));
#15917=DIRECTION('center_axis',(0.,0.,-1.));
#15918=DIRECTION('ref_axis',(1.,-3.61224345087086E-14,0.));
#15919=DIRECTION('',(1.22464679914735E-16,-4.4387199776766E-30,-1.));
#15920=DIRECTION('center_axis',(0.,0.,-1.));
#15921=DIRECTION('ref_axis',(1.,-3.61224345087086E-14,0.));
#15922=DIRECTION('',(1.22464679914735E-16,-4.4387199776766E-30,-1.));
#15923=DIRECTION('center_axis',(0.,0.,-1.));
#15924=DIRECTION('ref_axis',(1.,-3.61224345087086E-14,0.));
#15925=DIRECTION('',(1.22464679914735E-16,-4.4387199776766E-30,-1.));
#15926=DIRECTION('center_axis',(0.,0.,-1.));
#15927=DIRECTION('ref_axis',(1.,-3.61224345087086E-14,0.));
#15928=DIRECTION('',(1.22464679914735E-16,-4.4387199776766E-30,-1.));
#15929=DIRECTION('center_axis',(0.,0.,-1.));
#15930=DIRECTION('ref_axis',(-0.609168291270311,-0.793040978077936,0.));
#15931=DIRECTION('',(1.22464679914735E-16,-4.4387199776766E-30,-1.));
#15932=DIRECTION('center_axis',(0.,0.,-1.));
#15933=DIRECTION('ref_axis',(1.,-3.61224345087086E-14,0.));
#15934=DIRECTION('center_axis',(0.,0.,-1.));
#15935=DIRECTION('ref_axis',(1.,0.,0.));
#15936=DIRECTION('',(0.,0.,-1.));
#15937=DIRECTION('center_axis',(0.,0.,1.));
#15938=DIRECTION('ref_axis',(1.,0.,0.));
#15939=DIRECTION('',(0.,0.,-1.));
#15940=DIRECTION('center_axis',(0.,0.,-1.));
#15941=DIRECTION('ref_axis',(1.,0.,0.));
#15942=DIRECTION('center_axis',(0.,0.,1.));
#15943=DIRECTION('ref_axis',(1.,0.,0.));
#15944=DIRECTION('center_axis',(0.,0.,-1.));
#15945=DIRECTION('ref_axis',(1.,0.,0.));
#15946=DIRECTION('',(0.,0.,-1.));
#15947=DIRECTION('center_axis',(0.,0.,-1.));
#15948=DIRECTION('ref_axis',(1.,0.,0.));
#15949=DIRECTION('',(0.,0.,-1.));
#15950=DIRECTION('center_axis',(0.,0.,-1.));
#15951=DIRECTION('ref_axis',(1.,0.,0.));
#15952=DIRECTION('',(0.,0.,-1.));
#15953=DIRECTION('center_axis',(0.,0.,-1.));
#15954=DIRECTION('ref_axis',(1.,0.,0.));
#15955=DIRECTION('',(0.,0.,-1.));
#15956=DIRECTION('center_axis',(0.,0.,-1.));
#15957=DIRECTION('ref_axis',(1.,0.,0.));
#15958=DIRECTION('',(0.,0.,-1.));
#15959=DIRECTION('center_axis',(0.,0.,-1.));
#15960=DIRECTION('ref_axis',(1.,0.,0.));
#15961=DIRECTION('',(0.,0.,-1.));
#15962=DIRECTION('center_axis',(0.,0.,-1.));
#15963=DIRECTION('ref_axis',(1.,0.,0.));
#15964=DIRECTION('',(0.,0.,-1.));
#15965=DIRECTION('center_axis',(0.,0.,-1.));
#15966=DIRECTION('ref_axis',(0.938009657291012,-0.346609121098678,0.));
#15967=DIRECTION('',(0.,0.,-1.));
#15968=DIRECTION('center_axis',(0.,0.,1.));
#15969=DIRECTION('ref_axis',(1.,0.,0.));
#15970=DIRECTION('center_axis',(0.,0.,-1.));
#15971=DIRECTION('ref_axis',(1.,-3.46775371283602E-14,0.));
#15972=DIRECTION('',(1.22464679914735E-16,-4.2617710824826E-30,-1.));
#15973=DIRECTION('center_axis',(0.,0.,1.));
#15974=DIRECTION('ref_axis',(1.,-3.46775371283602E-14,0.));
#15975=DIRECTION('center_axis',(0.,0.,-1.));
#15976=DIRECTION('ref_axis',(1.,-3.46775371283602E-14,0.));
#15977=DIRECTION('',(1.22464679914735E-16,-4.2617710824826E-30,-1.));
#15978=DIRECTION('center_axis',(0.,0.,-1.));
#15979=DIRECTION('ref_axis',(1.,-3.46775371283602E-14,0.));
#15980=DIRECTION('',(1.22464679914735E-16,-4.2617710824826E-30,-1.));
#15981=DIRECTION('center_axis',(0.,0.,-1.));
#15982=DIRECTION('ref_axis',(1.,-3.46775371283602E-14,0.));
#15983=DIRECTION('',(1.22464679914735E-16,-4.2617710824826E-30,-1.));
#15984=DIRECTION('center_axis',(0.,0.,-1.));
#15985=DIRECTION('ref_axis',(1.,-3.46775371283602E-14,0.));
#15986=DIRECTION('',(1.22464679914735E-16,-4.2617710824826E-30,-1.));
#15987=DIRECTION('center_axis',(0.,0.,-1.));
#15988=DIRECTION('ref_axis',(1.,-3.46775371283602E-14,0.));
#15989=DIRECTION('',(1.22464679914735E-16,-4.2617710824826E-30,-1.));
#15990=DIRECTION('center_axis',(0.,0.,-1.));
#15991=DIRECTION('ref_axis',(1.,-3.46775371283602E-14,0.));
#15992=DIRECTION('',(1.22464679914735E-16,-4.2617710824826E-30,-1.));
#15993=DIRECTION('center_axis',(0.,0.,-1.));
#15994=DIRECTION('ref_axis',(1.,-3.46775371283602E-14,0.));
#15995=DIRECTION('',(1.22464679914735E-16,-4.2617710824826E-30,-1.));
#15996=DIRECTION('center_axis',(0.,0.,-1.));
#15997=DIRECTION('ref_axis',(-0.609168284311007,-0.793040983423672,0.));
#15998=DIRECTION('',(1.22464679914735E-16,-4.2617710824826E-30,-1.));
#15999=DIRECTION('center_axis',(0.,0.,-1.));
#16000=DIRECTION('ref_axis',(1.,-3.46775371283602E-14,0.));
#16001=DIRECTION('center_axis',(0.,0.,-1.));
#16002=DIRECTION('ref_axis',(1.,0.,0.));
#16003=DIRECTION('',(0.,0.,-1.));
#16004=DIRECTION('center_axis',(0.,0.,1.));
#16005=DIRECTION('ref_axis',(1.,0.,0.));
#16006=DIRECTION('',(0.,0.,-1.));
#16007=DIRECTION('center_axis',(0.,0.,-1.));
#16008=DIRECTION('ref_axis',(1.,0.,0.));
#16009=DIRECTION('center_axis',(0.,0.,1.));
#16010=DIRECTION('ref_axis',(1.,0.,0.));
#16011=DIRECTION('center_axis',(0.,0.,-1.));
#16012=DIRECTION('ref_axis',(1.,0.,0.));
#16013=DIRECTION('',(0.,0.,-1.));
#16014=DIRECTION('center_axis',(0.,0.,-1.));
#16015=DIRECTION('ref_axis',(1.,0.,0.));
#16016=DIRECTION('',(0.,0.,-1.));
#16017=DIRECTION('center_axis',(0.,0.,-1.));
#16018=DIRECTION('ref_axis',(1.,0.,0.));
#16019=DIRECTION('',(0.,0.,-1.));
#16020=DIRECTION('center_axis',(0.,0.,-1.));
#16021=DIRECTION('ref_axis',(1.,0.,0.));
#16022=DIRECTION('',(0.,0.,-1.));
#16023=DIRECTION('center_axis',(0.,0.,-1.));
#16024=DIRECTION('ref_axis',(1.,0.,0.));
#16025=DIRECTION('',(0.,0.,-1.));
#16026=DIRECTION('center_axis',(0.,0.,-1.));
#16027=DIRECTION('ref_axis',(1.,0.,0.));
#16028=DIRECTION('',(0.,0.,-1.));
#16029=DIRECTION('center_axis',(0.,0.,-1.));
#16030=DIRECTION('ref_axis',(1.,0.,0.));
#16031=DIRECTION('',(0.,0.,-1.));
#16032=DIRECTION('center_axis',(0.,0.,-1.));
#16033=DIRECTION('ref_axis',(0.938009661722287,-0.346609109106558,0.));
#16034=DIRECTION('',(0.,0.,-1.));
#16035=DIRECTION('center_axis',(0.,0.,1.));
#16036=DIRECTION('ref_axis',(1.,0.,0.));
#16037=DIRECTION('center_axis',(0.,0.,-1.));
#16038=DIRECTION('ref_axis',(1.,-3.46775371283602E-14,0.));
#16039=DIRECTION('',(1.22464679914735E-16,-4.2617710824826E-30,-1.));
#16040=DIRECTION('center_axis',(0.,0.,1.));
#16041=DIRECTION('ref_axis',(1.,-3.46775371283602E-14,0.));
#16042=DIRECTION('center_axis',(0.,0.,-1.));
#16043=DIRECTION('ref_axis',(1.,-3.46775371283602E-14,0.));
#16044=DIRECTION('',(1.22464679914735E-16,-4.2617710824826E-30,-1.));
#16045=DIRECTION('center_axis',(0.,0.,-1.));
#16046=DIRECTION('ref_axis',(1.,-3.46775371283602E-14,0.));
#16047=DIRECTION('',(1.22464679914735E-16,-4.2617710824826E-30,-1.));
#16048=DIRECTION('center_axis',(0.,0.,-1.));
#16049=DIRECTION('ref_axis',(1.,-3.46775371283602E-14,0.));
#16050=DIRECTION('',(1.22464679914735E-16,-4.2617710824826E-30,-1.));
#16051=DIRECTION('center_axis',(0.,0.,-1.));
#16052=DIRECTION('ref_axis',(1.,-3.46775371283602E-14,0.));
#16053=DIRECTION('',(1.22464679914735E-16,-4.2617710824826E-30,-1.));
#16054=DIRECTION('center_axis',(0.,0.,-1.));
#16055=DIRECTION('ref_axis',(1.,-3.46775371283602E-14,0.));
#16056=DIRECTION('',(1.22464679914735E-16,-4.2617710824826E-30,-1.));
#16057=DIRECTION('center_axis',(0.,0.,-1.));
#16058=DIRECTION('ref_axis',(1.,-3.46775371283602E-14,0.));
#16059=DIRECTION('',(1.22464679914735E-16,-4.2617710824826E-30,-1.));
#16060=DIRECTION('center_axis',(0.,0.,-1.));
#16061=DIRECTION('ref_axis',(1.,-3.46775371283602E-14,0.));
#16062=DIRECTION('',(1.22464679914735E-16,-4.2617710824826E-30,-1.));
#16063=DIRECTION('center_axis',(0.,0.,-1.));
#16064=DIRECTION('ref_axis',(-0.609168295488507,-0.793040974837761,0.));
#16065=DIRECTION('',(1.22464679914735E-16,-4.2617710824826E-30,-1.));
#16066=DIRECTION('center_axis',(0.,0.,-1.));
#16067=DIRECTION('ref_axis',(1.,-3.46775371283602E-14,0.));
#16068=DIRECTION('center_axis',(0.,0.,-1.));
#16069=DIRECTION('ref_axis',(1.,0.,0.));
#16070=DIRECTION('',(0.,0.,-1.));
#16071=DIRECTION('center_axis',(0.,0.,1.));
#16072=DIRECTION('ref_axis',(1.,0.,0.));
#16073=DIRECTION('',(0.,0.,-1.));
#16074=DIRECTION('center_axis',(0.,0.,-1.));
#16075=DIRECTION('ref_axis',(1.,0.,0.));
#16076=DIRECTION('center_axis',(0.,0.,1.));
#16077=DIRECTION('ref_axis',(1.,0.,0.));
#16078=DIRECTION('center_axis',(0.,0.,-1.));
#16079=DIRECTION('ref_axis',(1.,0.,0.));
#16080=DIRECTION('',(0.,0.,-1.));
#16081=DIRECTION('center_axis',(0.,0.,-1.));
#16082=DIRECTION('ref_axis',(1.,0.,0.));
#16083=DIRECTION('',(0.,0.,-1.));
#16084=DIRECTION('center_axis',(0.,0.,-1.));
#16085=DIRECTION('ref_axis',(1.,0.,0.));
#16086=DIRECTION('',(0.,0.,-1.));
#16087=DIRECTION('center_axis',(0.,0.,-1.));
#16088=DIRECTION('ref_axis',(1.,0.,0.));
#16089=DIRECTION('',(0.,0.,-1.));
#16090=DIRECTION('center_axis',(0.,0.,-1.));
#16091=DIRECTION('ref_axis',(1.,0.,0.));
#16092=DIRECTION('',(0.,0.,-1.));
#16093=DIRECTION('center_axis',(0.,0.,-1.));
#16094=DIRECTION('ref_axis',(1.,0.,0.));
#16095=DIRECTION('',(0.,0.,-1.));
#16096=DIRECTION('center_axis',(0.,0.,-1.));
#16097=DIRECTION('ref_axis',(1.,0.,0.));
#16098=DIRECTION('',(0.,0.,-1.));
#16099=DIRECTION('center_axis',(0.,0.,-1.));
#16100=DIRECTION('ref_axis',(0.938009665675849,-0.346609098407243,0.));
#16101=DIRECTION('',(0.,0.,-1.));
#16102=DIRECTION('center_axis',(0.,0.,1.));
#16103=DIRECTION('ref_axis',(1.,0.,0.));
#16104=DIRECTION('center_axis',(0.,0.,-1.));
#16105=DIRECTION('ref_axis',(1.,-3.46775371283602E-14,0.));
#16106=DIRECTION('',(1.22464679914735E-16,-4.2617710824826E-30,-1.));
#16107=DIRECTION('center_axis',(0.,0.,1.));
#16108=DIRECTION('ref_axis',(1.,-3.46775371283602E-14,0.));
#16109=DIRECTION('center_axis',(0.,0.,-1.));
#16110=DIRECTION('ref_axis',(1.,-3.46775371283602E-14,0.));
#16111=DIRECTION('',(1.22464679914735E-16,-4.2617710824826E-30,-1.));
#16112=DIRECTION('center_axis',(0.,0.,-1.));
#16113=DIRECTION('ref_axis',(1.,-3.46775371283602E-14,0.));
#16114=DIRECTION('',(1.22464679914735E-16,-4.2617710824826E-30,-1.));
#16115=DIRECTION('center_axis',(0.,0.,-1.));
#16116=DIRECTION('ref_axis',(1.,-3.46775371283602E-14,0.));
#16117=DIRECTION('',(1.22464679914735E-16,-4.2617710824826E-30,-1.));
#16118=DIRECTION('center_axis',(0.,0.,-1.));
#16119=DIRECTION('ref_axis',(1.,-3.46775371283602E-14,0.));
#16120=DIRECTION('',(1.22464679914735E-16,-4.2617710824826E-30,-1.));
#16121=DIRECTION('center_axis',(0.,0.,-1.));
#16122=DIRECTION('ref_axis',(1.,-3.46775371283602E-14,0.));
#16123=DIRECTION('',(1.22464679914735E-16,-4.2617710824826E-30,-1.));
#16124=DIRECTION('center_axis',(0.,0.,-1.));
#16125=DIRECTION('ref_axis',(1.,-3.46775371283602E-14,0.));
#16126=DIRECTION('',(1.22464679914735E-16,-4.2617710824826E-30,-1.));
#16127=DIRECTION('center_axis',(0.,0.,-1.));
#16128=DIRECTION('ref_axis',(1.,-3.46775371283602E-14,0.));
#16129=DIRECTION('',(1.22464679914735E-16,-4.2617710824826E-30,-1.));
#16130=DIRECTION('center_axis',(0.,0.,-1.));
#16131=DIRECTION('ref_axis',(-0.609168291270306,-0.79304097807794,0.));
#16132=DIRECTION('',(1.22464679914735E-16,-4.2617710824826E-30,-1.));
#16133=DIRECTION('center_axis',(0.,0.,-1.));
#16134=DIRECTION('ref_axis',(1.,-3.46775371283602E-14,0.));
#16135=DIRECTION('center_axis',(0.,0.,-1.));
#16136=DIRECTION('ref_axis',(1.,0.,0.));
#16137=DIRECTION('',(0.,0.,-1.));
#16138=DIRECTION('center_axis',(0.,0.,1.));
#16139=DIRECTION('ref_axis',(1.,0.,0.));
#16140=DIRECTION('',(0.,0.,-1.));
#16141=DIRECTION('center_axis',(0.,0.,-1.));
#16142=DIRECTION('ref_axis',(1.,0.,0.));
#16143=DIRECTION('center_axis',(0.,0.,1.));
#16144=DIRECTION('ref_axis',(1.,0.,0.));
#16145=DIRECTION('center_axis',(0.,0.,-1.));
#16146=DIRECTION('ref_axis',(1.,0.,0.));
#16147=DIRECTION('',(0.,0.,-1.));
#16148=DIRECTION('center_axis',(0.,0.,-1.));
#16149=DIRECTION('ref_axis',(1.,0.,0.));
#16150=DIRECTION('',(0.,0.,-1.));
#16151=DIRECTION('center_axis',(0.,0.,-1.));
#16152=DIRECTION('ref_axis',(1.,0.,0.));
#16153=DIRECTION('',(0.,0.,-1.));
#16154=DIRECTION('center_axis',(0.,0.,-1.));
#16155=DIRECTION('ref_axis',(1.,0.,0.));
#16156=DIRECTION('',(0.,0.,-1.));
#16157=DIRECTION('center_axis',(0.,0.,-1.));
#16158=DIRECTION('ref_axis',(1.,0.,0.));
#16159=DIRECTION('',(0.,0.,-1.));
#16160=DIRECTION('center_axis',(0.,0.,-1.));
#16161=DIRECTION('ref_axis',(1.,0.,0.));
#16162=DIRECTION('',(0.,0.,-1.));
#16163=DIRECTION('center_axis',(0.,0.,-1.));
#16164=DIRECTION('ref_axis',(1.,0.,0.));
#16165=DIRECTION('',(0.,0.,-1.));
#16166=DIRECTION('center_axis',(0.,0.,-1.));
#16167=DIRECTION('ref_axis',(0.938009652374732,-0.346609134403343,0.));
#16168=DIRECTION('',(0.,0.,-1.));
#16169=DIRECTION('center_axis',(0.,0.,1.));
#16170=DIRECTION('ref_axis',(1.,0.,0.));
#16171=DIRECTION('center_axis',(0.,0.,-1.));
#16172=DIRECTION('ref_axis',(1.,-3.46775371283602E-14,0.));
#16173=DIRECTION('',(1.22464679914735E-16,-4.2617710824826E-30,-1.));
#16174=DIRECTION('center_axis',(0.,0.,1.));
#16175=DIRECTION('ref_axis',(1.,-3.46775371283602E-14,0.));
#16176=DIRECTION('center_axis',(0.,0.,-1.));
#16177=DIRECTION('ref_axis',(1.,-3.46775371283602E-14,0.));
#16178=DIRECTION('',(1.22464679914735E-16,-4.2617710824826E-30,-1.));
#16179=DIRECTION('center_axis',(0.,0.,-1.));
#16180=DIRECTION('ref_axis',(1.,-3.46775371283602E-14,0.));
#16181=DIRECTION('',(1.22464679914735E-16,-4.2617710824826E-30,-1.));
#16182=DIRECTION('center_axis',(0.,0.,-1.));
#16183=DIRECTION('ref_axis',(1.,-3.46775371283602E-14,0.));
#16184=DIRECTION('',(1.22464679914735E-16,-4.2617710824826E-30,-1.));
#16185=DIRECTION('center_axis',(0.,0.,-1.));
#16186=DIRECTION('ref_axis',(1.,-3.46775371283602E-14,0.));
#16187=DIRECTION('',(1.22464679914735E-16,-4.2617710824826E-30,-1.));
#16188=DIRECTION('center_axis',(0.,0.,-1.));
#16189=DIRECTION('ref_axis',(1.,-3.46775371283602E-14,0.));
#16190=DIRECTION('',(1.22464679914735E-16,-4.2617710824826E-30,-1.));
#16191=DIRECTION('center_axis',(0.,0.,-1.));
#16192=DIRECTION('ref_axis',(1.,-3.46775371283602E-14,0.));
#16193=DIRECTION('',(1.22464679914735E-16,-4.2617710824826E-30,-1.));
#16194=DIRECTION('center_axis',(0.,0.,-1.));
#16195=DIRECTION('ref_axis',(1.,-3.46775371283602E-14,0.));
#16196=DIRECTION('',(1.22464679914735E-16,-4.2617710824826E-30,-1.));
#16197=DIRECTION('center_axis',(0.,0.,-1.));
#16198=DIRECTION('ref_axis',(-0.609168287551074,-0.793040980934839,0.));
#16199=DIRECTION('',(1.22464679914735E-16,-4.2617710824826E-30,-1.));
#16200=DIRECTION('center_axis',(0.,0.,-1.));
#16201=DIRECTION('ref_axis',(1.,-3.46775371283602E-14,0.));
#16202=DIRECTION('center_axis',(0.,0.,-1.));
#16203=DIRECTION('ref_axis',(1.,0.,0.));
#16204=DIRECTION('',(0.,0.,-1.));
#16205=DIRECTION('center_axis',(0.,0.,1.));
#16206=DIRECTION('ref_axis',(1.,0.,0.));
#16207=DIRECTION('',(0.,0.,-1.));
#16208=DIRECTION('center_axis',(0.,0.,-1.));
#16209=DIRECTION('ref_axis',(1.,0.,0.));
#16210=DIRECTION('center_axis',(0.,0.,1.));
#16211=DIRECTION('ref_axis',(1.,0.,0.));
#16212=DIRECTION('center_axis',(0.,0.,-1.));
#16213=DIRECTION('ref_axis',(1.,0.,0.));
#16214=DIRECTION('',(0.,0.,-1.));
#16215=DIRECTION('center_axis',(0.,0.,-1.));
#16216=DIRECTION('ref_axis',(1.,0.,0.));
#16217=DIRECTION('',(0.,0.,-1.));
#16218=DIRECTION('center_axis',(0.,0.,-1.));
#16219=DIRECTION('ref_axis',(1.,0.,0.));
#16220=DIRECTION('',(0.,0.,-1.));
#16221=DIRECTION('center_axis',(0.,0.,-1.));
#16222=DIRECTION('ref_axis',(1.,0.,0.));
#16223=DIRECTION('',(0.,0.,-1.));
#16224=DIRECTION('center_axis',(0.,0.,-1.));
#16225=DIRECTION('ref_axis',(1.,0.,0.));
#16226=DIRECTION('',(0.,0.,-1.));
#16227=DIRECTION('center_axis',(0.,0.,-1.));
#16228=DIRECTION('ref_axis',(1.,0.,0.));
#16229=DIRECTION('',(0.,0.,-1.));
#16230=DIRECTION('center_axis',(0.,0.,-1.));
#16231=DIRECTION('ref_axis',(1.,0.,0.));
#16232=DIRECTION('',(0.,0.,-1.));
#16233=DIRECTION('center_axis',(0.,0.,-1.));
#16234=DIRECTION('ref_axis',(0.938009657291017,-0.346609121098665,0.));
#16235=DIRECTION('',(0.,0.,-1.));
#16236=DIRECTION('center_axis',(0.,0.,1.));
#16237=DIRECTION('ref_axis',(1.,0.,0.));
#16238=DIRECTION('center_axis',(0.,0.,-1.));
#16239=DIRECTION('ref_axis',(1.,-4.04571266497535E-14,0.));
#16240=DIRECTION('',(1.22464679914735E-16,-4.9695666632586E-30,-1.));
#16241=DIRECTION('center_axis',(0.,0.,1.));
#16242=DIRECTION('ref_axis',(1.,-4.04571266497535E-14,0.));
#16243=DIRECTION('center_axis',(0.,0.,-1.));
#16244=DIRECTION('ref_axis',(1.,-4.04571266497535E-14,0.));
#16245=DIRECTION('',(1.22464679914735E-16,-4.9695666632586E-30,-1.));
#16246=DIRECTION('center_axis',(0.,0.,-1.));
#16247=DIRECTION('ref_axis',(1.,-4.04571266497535E-14,0.));
#16248=DIRECTION('',(1.22464679914735E-16,-4.9695666632586E-30,-1.));
#16249=DIRECTION('center_axis',(0.,0.,-1.));
#16250=DIRECTION('ref_axis',(1.,-4.04571266497535E-14,0.));
#16251=DIRECTION('',(1.22464679914735E-16,-4.9695666632586E-30,-1.));
#16252=DIRECTION('center_axis',(0.,0.,-1.));
#16253=DIRECTION('ref_axis',(1.,-4.04571266497535E-14,0.));
#16254=DIRECTION('',(1.22464679914735E-16,-4.9695666632586E-30,-1.));
#16255=DIRECTION('center_axis',(0.,0.,-1.));
#16256=DIRECTION('ref_axis',(1.,-4.04571266497535E-14,0.));
#16257=DIRECTION('',(1.22464679914735E-16,-4.9695666632586E-30,-1.));
#16258=DIRECTION('center_axis',(0.,0.,-1.));
#16259=DIRECTION('ref_axis',(1.,-4.04571266497535E-14,0.));
#16260=DIRECTION('',(1.22464679914735E-16,-4.9695666632586E-30,-1.));
#16261=DIRECTION('center_axis',(0.,0.,-1.));
#16262=DIRECTION('ref_axis',(1.,-4.04571266497535E-14,0.));
#16263=DIRECTION('',(1.22464679914735E-16,-4.9695666632586E-30,-1.));
#16264=DIRECTION('center_axis',(0.,0.,-1.));
#16265=DIRECTION('ref_axis',(-0.609168284311011,-0.793040983423669,0.));
#16266=DIRECTION('',(1.22464679914735E-16,-4.9695666632586E-30,-1.));
#16267=DIRECTION('center_axis',(0.,0.,-1.));
#16268=DIRECTION('ref_axis',(1.,-4.04571266497535E-14,0.));
#16269=DIRECTION('center_axis',(0.,0.,-1.));
#16270=DIRECTION('ref_axis',(1.,0.,0.));
#16271=DIRECTION('',(0.,0.,-1.));
#16272=DIRECTION('center_axis',(0.,0.,1.));
#16273=DIRECTION('ref_axis',(1.,0.,0.));
#16274=DIRECTION('',(0.,0.,-1.));
#16275=DIRECTION('center_axis',(0.,0.,-1.));
#16276=DIRECTION('ref_axis',(1.,0.,0.));
#16277=DIRECTION('center_axis',(0.,0.,1.));
#16278=DIRECTION('ref_axis',(1.,0.,0.));
#16279=DIRECTION('center_axis',(0.,0.,-1.));
#16280=DIRECTION('ref_axis',(1.,0.,0.));
#16281=DIRECTION('',(0.,0.,-1.));
#16282=DIRECTION('center_axis',(0.,0.,-1.));
#16283=DIRECTION('ref_axis',(1.,0.,0.));
#16284=DIRECTION('',(0.,0.,-1.));
#16285=DIRECTION('center_axis',(0.,0.,-1.));
#16286=DIRECTION('ref_axis',(1.,0.,0.));
#16287=DIRECTION('',(0.,0.,-1.));
#16288=DIRECTION('center_axis',(0.,0.,-1.));
#16289=DIRECTION('ref_axis',(1.,0.,0.));
#16290=DIRECTION('',(0.,0.,-1.));
#16291=DIRECTION('center_axis',(0.,0.,-1.));
#16292=DIRECTION('ref_axis',(1.,0.,0.));
#16293=DIRECTION('',(0.,0.,-1.));
#16294=DIRECTION('center_axis',(0.,0.,-1.));
#16295=DIRECTION('ref_axis',(1.,0.,0.));
#16296=DIRECTION('',(0.,0.,-1.));
#16297=DIRECTION('center_axis',(0.,0.,-1.));
#16298=DIRECTION('ref_axis',(1.,0.,0.));
#16299=DIRECTION('',(0.,0.,-1.));
#16300=DIRECTION('center_axis',(0.,0.,-1.));
#16301=DIRECTION('ref_axis',(0.938009652374729,-0.346609134403351,0.));
#16302=DIRECTION('',(0.,0.,-1.));
#16303=DIRECTION('center_axis',(0.,0.,1.));
#16304=DIRECTION('ref_axis',(1.,0.,0.));
#16305=DIRECTION('center_axis',(0.,0.,-1.));
#16306=DIRECTION('ref_axis',(1.,-2.88979476069668E-14,0.));
#16307=DIRECTION('',(1.22464679914735E-16,-3.5539755017066E-30,-1.));
#16308=DIRECTION('center_axis',(0.,0.,1.));
#16309=DIRECTION('ref_axis',(1.,-2.88979476069668E-14,0.));
#16310=DIRECTION('center_axis',(0.,0.,-1.));
#16311=DIRECTION('ref_axis',(1.,-2.88979476069668E-14,0.));
#16312=DIRECTION('',(1.22464679914735E-16,-3.5539755017066E-30,-1.));
#16313=DIRECTION('center_axis',(0.,0.,-1.));
#16314=DIRECTION('ref_axis',(1.,-2.88979476069668E-14,0.));
#16315=DIRECTION('',(1.22464679914735E-16,-3.5539755017066E-30,-1.));
#16316=DIRECTION('center_axis',(0.,0.,-1.));
#16317=DIRECTION('ref_axis',(1.,-2.88979476069668E-14,0.));
#16318=DIRECTION('',(1.22464679914735E-16,-3.5539755017066E-30,-1.));
#16319=DIRECTION('center_axis',(0.,0.,-1.));
#16320=DIRECTION('ref_axis',(1.,-2.88979476069668E-14,0.));
#16321=DIRECTION('',(1.22464679914735E-16,-3.5539755017066E-30,-1.));
#16322=DIRECTION('center_axis',(0.,0.,-1.));
#16323=DIRECTION('ref_axis',(1.,-2.88979476069668E-14,0.));
#16324=DIRECTION('',(1.22464679914735E-16,-3.5539755017066E-30,-1.));
#16325=DIRECTION('center_axis',(0.,0.,-1.));
#16326=DIRECTION('ref_axis',(1.,-2.88979476069668E-14,0.));
#16327=DIRECTION('',(1.22464679914735E-16,-3.5539755017066E-30,-1.));
#16328=DIRECTION('center_axis',(0.,0.,-1.));
#16329=DIRECTION('ref_axis',(1.,-2.88979476069668E-14,0.));
#16330=DIRECTION('',(1.22464679914735E-16,-3.5539755017066E-30,-1.));
#16331=DIRECTION('center_axis',(0.,0.,-1.));
#16332=DIRECTION('ref_axis',(-0.609168287551063,-0.793040980934848,0.));
#16333=DIRECTION('',(1.22464679914735E-16,-3.5539755017066E-30,-1.));
#16334=DIRECTION('center_axis',(0.,0.,-1.));
#16335=DIRECTION('ref_axis',(1.,-2.88979476069668E-14,0.));
#16336=DIRECTION('center_axis',(0.,0.,-1.));
#16337=DIRECTION('ref_axis',(1.,0.,0.));
#16338=DIRECTION('',(0.,0.,-1.));
#16339=DIRECTION('center_axis',(0.,0.,1.));
#16340=DIRECTION('ref_axis',(1.,0.,0.));
#16341=DIRECTION('',(0.,0.,-1.));
#16342=DIRECTION('center_axis',(0.,0.,-1.));
#16343=DIRECTION('ref_axis',(1.,0.,0.));
#16344=DIRECTION('center_axis',(0.,0.,1.));
#16345=DIRECTION('ref_axis',(1.,0.,0.));
#16346=DIRECTION('center_axis',(0.,0.,-1.));
#16347=DIRECTION('ref_axis',(1.,0.,0.));
#16348=DIRECTION('',(0.,0.,-1.));
#16349=DIRECTION('center_axis',(0.,0.,-1.));
#16350=DIRECTION('ref_axis',(1.,0.,0.));
#16351=DIRECTION('',(0.,0.,-1.));
#16352=DIRECTION('center_axis',(0.,0.,-1.));
#16353=DIRECTION('ref_axis',(1.,0.,0.));
#16354=DIRECTION('',(0.,0.,-1.));
#16355=DIRECTION('center_axis',(0.,0.,-1.));
#16356=DIRECTION('ref_axis',(1.,0.,0.));
#16357=DIRECTION('',(0.,0.,-1.));
#16358=DIRECTION('center_axis',(0.,0.,-1.));
#16359=DIRECTION('ref_axis',(1.,0.,0.));
#16360=DIRECTION('',(0.,0.,-1.));
#16361=DIRECTION('center_axis',(0.,0.,-1.));
#16362=DIRECTION('ref_axis',(1.,0.,0.));
#16363=DIRECTION('',(0.,0.,-1.));
#16364=DIRECTION('center_axis',(0.,0.,-1.));
#16365=DIRECTION('ref_axis',(1.,0.,0.));
#16366=DIRECTION('',(0.,0.,-1.));
#16367=DIRECTION('center_axis',(0.,0.,-1.));
#16368=DIRECTION('ref_axis',(0.93800966172229,-0.346609109106549,0.));
#16369=DIRECTION('',(0.,0.,-1.));
#16370=DIRECTION('center_axis',(0.,0.,1.));
#16371=DIRECTION('ref_axis',(1.,0.,0.));
#16372=DIRECTION('center_axis',(0.,0.,-1.));
#16373=DIRECTION('ref_axis',(1.,-3.32326397480119E-14,0.));
#16374=DIRECTION('',(1.22464679914735E-16,-4.0848221872886E-30,-1.));
#16375=DIRECTION('center_axis',(0.,0.,1.));
#16376=DIRECTION('ref_axis',(1.,-3.32326397480119E-14,0.));
#16377=DIRECTION('center_axis',(0.,0.,-1.));
#16378=DIRECTION('ref_axis',(1.,-3.32326397480119E-14,0.));
#16379=DIRECTION('',(1.22464679914735E-16,-4.0848221872886E-30,-1.));
#16380=DIRECTION('center_axis',(0.,0.,-1.));
#16381=DIRECTION('ref_axis',(1.,-3.32326397480119E-14,0.));
#16382=DIRECTION('',(1.22464679914735E-16,-4.0848221872886E-30,-1.));
#16383=DIRECTION('center_axis',(0.,0.,-1.));
#16384=DIRECTION('ref_axis',(1.,-3.32326397480119E-14,0.));
#16385=DIRECTION('',(1.22464679914735E-16,-4.0848221872886E-30,-1.));
#16386=DIRECTION('center_axis',(0.,0.,-1.));
#16387=DIRECTION('ref_axis',(1.,-3.32326397480119E-14,0.));
#16388=DIRECTION('',(1.22464679914735E-16,-4.0848221872886E-30,-1.));
#16389=DIRECTION('center_axis',(0.,0.,-1.));
#16390=DIRECTION('ref_axis',(1.,-3.32326397480119E-14,0.));
#16391=DIRECTION('',(1.22464679914735E-16,-4.0848221872886E-30,-1.));
#16392=DIRECTION('center_axis',(0.,0.,-1.));
#16393=DIRECTION('ref_axis',(1.,-3.32326397480119E-14,0.));
#16394=DIRECTION('',(1.22464679914735E-16,-4.0848221872886E-30,-1.));
#16395=DIRECTION('center_axis',(0.,0.,-1.));
#16396=DIRECTION('ref_axis',(1.,-3.32326397480119E-14,0.));
#16397=DIRECTION('',(1.22464679914735E-16,-4.0848221872886E-30,-1.));
#16398=DIRECTION('center_axis',(0.,0.,-1.));
#16399=DIRECTION('ref_axis',(-0.609168295488513,-0.793040974837757,0.));
#16400=DIRECTION('',(1.22464679914735E-16,-4.0848221872886E-30,-1.));
#16401=DIRECTION('center_axis',(0.,0.,-1.));
#16402=DIRECTION('ref_axis',(1.,-3.32326397480119E-14,0.));
#16403=DIRECTION('center_axis',(0.,0.,-1.));
#16404=DIRECTION('ref_axis',(1.,0.,0.));
#16405=DIRECTION('center_axis',(0.,0.,-1.));
#16406=DIRECTION('ref_axis',(1.,0.,0.));
#16407=DIRECTION('',(0.,0.,-1.));
#16408=DIRECTION('center_axis',(0.,0.,-1.));
#16409=DIRECTION('ref_axis',(1.,0.,0.));
#16410=DIRECTION('center_axis',(0.,0.,-1.));
#16411=DIRECTION('ref_axis',(1.,0.,0.));
#16412=DIRECTION('center_axis',(0.,0.,1.));
#16413=DIRECTION('ref_axis',(1.,0.,0.));
#16414=DIRECTION('center_axis',(0.,0.,-1.));
#16415=DIRECTION('ref_axis',(1.,0.,0.));
#16416=DIRECTION('center_axis',(0.,0.,-1.));
#16417=DIRECTION('ref_axis',(1.,0.,0.));
#16418=DIRECTION('',(0.,0.,-1.));
#16419=DIRECTION('center_axis',(0.,0.,-1.));
#16420=DIRECTION('ref_axis',(1.,0.,0.));
#16421=DIRECTION('center_axis',(0.,0.,-1.));
#16422=DIRECTION('ref_axis',(1.,0.,0.));
#16423=DIRECTION('center_axis',(0.,0.,1.));
#16424=DIRECTION('ref_axis',(1.,0.,0.));
#16425=DIRECTION('center_axis',(0.,0.,-1.));
#16426=DIRECTION('ref_axis',(1.,0.,0.));
#16427=DIRECTION('center_axis',(0.,0.,-1.));
#16428=DIRECTION('ref_axis',(1.,0.,0.));
#16429=DIRECTION('',(0.,0.,-1.));
#16430=DIRECTION('center_axis',(0.,0.,-1.));
#16431=DIRECTION('ref_axis',(1.,0.,0.));
#16432=DIRECTION('center_axis',(0.,0.,-1.));
#16433=DIRECTION('ref_axis',(1.,0.,0.));
#16434=DIRECTION('center_axis',(0.,0.,1.));
#16435=DIRECTION('ref_axis',(1.,0.,0.));
#16436=DIRECTION('center_axis',(0.,0.,-1.));
#16437=DIRECTION('ref_axis',(1.,0.,0.));
#16438=DIRECTION('center_axis',(0.,0.,-1.));
#16439=DIRECTION('ref_axis',(1.,0.,0.));
#16440=DIRECTION('',(0.,0.,-1.));
#16441=DIRECTION('center_axis',(0.,0.,-1.));
#16442=DIRECTION('ref_axis',(1.,0.,0.));
#16443=DIRECTION('center_axis',(0.,0.,-1.));
#16444=DIRECTION('ref_axis',(1.,0.,0.));
#16445=DIRECTION('center_axis',(0.,0.,1.));
#16446=DIRECTION('ref_axis',(1.,0.,0.));
#16447=DIRECTION('center_axis',(0.,0.,-1.));
#16448=DIRECTION('ref_axis',(1.,0.,0.));
#16449=DIRECTION('',(0.,0.,-1.));
#16450=DIRECTION('center_axis',(0.,0.,1.));
#16451=DIRECTION('ref_axis',(1.,0.,0.));
#16452=DIRECTION('center_axis',(0.,0.,-1.));
#16453=DIRECTION('ref_axis',(1.,0.,0.));
#16454=DIRECTION('',(0.,0.,-1.));
#16455=DIRECTION('center_axis',(0.,0.,1.));
#16456=DIRECTION('ref_axis',(1.,0.,0.));
#16457=DIRECTION('center_axis',(0.,0.,-1.));
#16458=DIRECTION('ref_axis',(1.,0.,0.));
#16459=DIRECTION('',(0.,0.,-1.));
#16460=DIRECTION('center_axis',(0.,0.,1.));
#16461=DIRECTION('ref_axis',(1.,0.,0.));
#16462=DIRECTION('center_axis',(0.,0.,-1.));
#16463=DIRECTION('ref_axis',(1.,0.,0.));
#16464=DIRECTION('',(0.,0.,-1.));
#16465=DIRECTION('center_axis',(0.,0.,1.));
#16466=DIRECTION('ref_axis',(1.,0.,0.));
#16467=DIRECTION('center_axis',(0.,0.,1.));
#16468=DIRECTION('ref_axis',(1.,0.,0.));
#16469=DIRECTION('center_axis',(0.,0.,-1.));
#16470=DIRECTION('ref_axis',(1.,-3.32326397480119E-14,0.));
#16471=DIRECTION('center_axis',(0.,0.,-1.));
#16472=DIRECTION('ref_axis',(1.,0.,0.));
#16473=DIRECTION('center_axis',(0.,0.,1.));
#16474=DIRECTION('ref_axis',(1.,0.,0.));
#16475=DIRECTION('center_axis',(0.,0.,-1.));
#16476=DIRECTION('ref_axis',(1.,-2.88979476069668E-14,0.));
#16477=DIRECTION('center_axis',(0.,0.,-1.));
#16478=DIRECTION('ref_axis',(1.,0.,0.));
#16479=DIRECTION('center_axis',(0.,0.,1.));
#16480=DIRECTION('ref_axis',(1.,0.,0.));
#16481=DIRECTION('center_axis',(0.,0.,-1.));
#16482=DIRECTION('ref_axis',(1.,-4.04571266497535E-14,0.));
#16483=DIRECTION('center_axis',(0.,0.,-1.));
#16484=DIRECTION('ref_axis',(1.,0.,0.));
#16485=DIRECTION('center_axis',(0.,0.,1.));
#16486=DIRECTION('ref_axis',(1.,0.,0.));
#16487=DIRECTION('center_axis',(0.,0.,-1.));
#16488=DIRECTION('ref_axis',(1.,-3.46775371283602E-14,0.));
#16489=DIRECTION('center_axis',(0.,0.,-1.));
#16490=DIRECTION('ref_axis',(1.,0.,0.));
#16491=DIRECTION('center_axis',(0.,0.,1.));
#16492=DIRECTION('ref_axis',(1.,0.,0.));
#16493=DIRECTION('center_axis',(0.,0.,-1.));
#16494=DIRECTION('ref_axis',(1.,-3.46775371283602E-14,0.));
#16495=DIRECTION('center_axis',(0.,0.,-1.));
#16496=DIRECTION('ref_axis',(1.,0.,0.));
#16497=DIRECTION('center_axis',(0.,0.,1.));
#16498=DIRECTION('ref_axis',(1.,0.,0.));
#16499=DIRECTION('center_axis',(0.,0.,-1.));
#16500=DIRECTION('ref_axis',(1.,-3.46775371283602E-14,0.));
#16501=DIRECTION('center_axis',(0.,0.,-1.));
#16502=DIRECTION('ref_axis',(1.,0.,0.));
#16503=DIRECTION('center_axis',(0.,0.,1.));
#16504=DIRECTION('ref_axis',(1.,0.,0.));
#16505=DIRECTION('center_axis',(0.,0.,-1.));
#16506=DIRECTION('ref_axis',(1.,-3.46775371283602E-14,0.));
#16507=DIRECTION('center_axis',(0.,0.,-1.));
#16508=DIRECTION('ref_axis',(1.,0.,0.));
#16509=DIRECTION('center_axis',(0.,0.,1.));
#16510=DIRECTION('ref_axis',(1.,0.,0.));
#16511=DIRECTION('center_axis',(0.,0.,-1.));
#16512=DIRECTION('ref_axis',(1.,-3.61224345087086E-14,0.));
#16513=DIRECTION('center_axis',(0.,0.,-1.));
#16514=DIRECTION('ref_axis',(1.,0.,0.));
#16515=DIRECTION('center_axis',(-1.,0.,0.));
#16516=DIRECTION('ref_axis',(0.,1.,0.));
#16517=DIRECTION('',(0.,0.,1.));
#16518=DIRECTION('',(0.,1.,0.));
#16519=DIRECTION('',(0.,0.,-1.));
#16520=DIRECTION('',(0.,1.,0.));
#16521=DIRECTION('center_axis',(0.,1.,0.));
#16522=DIRECTION('ref_axis',(1.,0.,0.));
#16523=DIRECTION('',(0.,0.,-1.));
#16524=DIRECTION('',(1.,0.,0.));
#16525=DIRECTION('',(1.,0.,0.));
#16526=DIRECTION('',(0.,0.,-1.));
#16527=DIRECTION('',(1.,0.,0.));
#16528=DIRECTION('',(0.,0.,1.));
#16529=DIRECTION('',(-1.,0.,0.));
#16530=DIRECTION('',(0.,0.,1.));
#16531=DIRECTION('',(1.,0.,0.));
#16532=DIRECTION('',(0.,0.,-1.));
#16533=DIRECTION('',(-1.,0.,0.));
#16534=DIRECTION('center_axis',(1.,0.,0.));
#16535=DIRECTION('ref_axis',(0.,-1.,0.));
#16536=DIRECTION('',(0.,0.,-1.));
#16537=DIRECTION('',(0.,-1.,0.));
#16538=DIRECTION('',(0.,-1.,0.));
#16539=DIRECTION('center_axis',(0.,0.,-1.));
#16540=DIRECTION('ref_axis',(-1.,0.,0.));
#16541=DIRECTION('center_axis',(0.,0.,-1.));
#16542=DIRECTION('ref_axis',(1.,0.,0.));
#16543=DIRECTION('center_axis',(0.,-1.,0.));
#16544=DIRECTION('ref_axis',(-1.,0.,0.));
#16545=DIRECTION('',(0.,0.,-1.));
#16546=DIRECTION('',(-1.,0.,0.));
#16547=DIRECTION('',(0.,0.,-1.));
#16548=DIRECTION('',(-1.,0.,0.));
#16549=DIRECTION('',(0.,0.,-1.));
#16550=DIRECTION('',(-1.,0.,0.));
#16551=DIRECTION('',(0.,0.,1.));
#16552=DIRECTION('',(1.,0.,0.));
#16553=DIRECTION('',(0.,0.,1.));
#16554=DIRECTION('',(-1.,0.,0.));
#16555=DIRECTION('',(0.,0.,-1.));
#16556=DIRECTION('',(1.,0.,0.));
#16557=DIRECTION('center_axis',(1.,0.,0.));
#16558=DIRECTION('ref_axis',(0.,-1.,0.));
#16559=DIRECTION('',(0.,0.,1.));
#16560=DIRECTION('',(0.,-1.,0.));
#16561=DIRECTION('',(0.,-1.,0.));
#16562=DIRECTION('center_axis',(-1.,0.,0.));
#16563=DIRECTION('ref_axis',(0.,1.,0.));
#16564=DIRECTION('',(0.,0.,-1.));
#16565=DIRECTION('',(0.,1.,0.));
#16566=DIRECTION('',(0.,1.,0.));
#16567=DIRECTION('center_axis',(0.,0.,-1.));
#16568=DIRECTION('ref_axis',(-1.,0.,0.));
#16569=DIRECTION('center_axis',(0.,0.,-1.));
#16570=DIRECTION('ref_axis',(1.,0.,0.));
#16571=DIRECTION('center_axis',(0.,0.,-1.));
#16572=DIRECTION('ref_axis',(-1.,0.,0.));
#16573=DIRECTION('',(0.,-1.,0.));
#16574=DIRECTION('',(1.,0.,0.));
#16575=DIRECTION('center_axis',(0.,0.,1.));
#16576=DIRECTION('ref_axis',(1.,0.,0.));
#16577=DIRECTION('',(1.,0.,0.));
#16578=DIRECTION('',(0.,1.,0.));
#16579=DIRECTION('center_axis',(1.,0.,0.));
#16580=DIRECTION('ref_axis',(0.,-1.,0.));
#16581=DIRECTION('',(0.,1.,0.));
#16582=DIRECTION('',(0.,0.,-1.));
#16583=DIRECTION('center_axis',(0.,0.,1.));
#16584=DIRECTION('ref_axis',(1.,0.,0.));
#16585=DIRECTION('center_axis',(0.,0.,1.));
#16586=DIRECTION('ref_axis',(1.,0.,0.));
#16587=DIRECTION('',(-1.,0.,0.));
#16588=DIRECTION('',(0.,1.,0.));
#16589=DIRECTION('',(-1.,0.,0.));
#16590=DIRECTION('',(0.,1.,0.));
#16591=DIRECTION('center_axis',(0.,0.,-1.));
#16592=DIRECTION('ref_axis',(1.,0.,0.));
#16593=DIRECTION('',(1.,0.,0.));
#16594=DIRECTION('',(0.,-1.,0.));
#16595=DIRECTION('center_axis',(0.,0.,1.));
#16596=DIRECTION('ref_axis',(1.,0.,0.));
#16597=DIRECTION('',(0.,1.,0.));
#16598=DIRECTION('',(1.,0.,0.));
#16599=DIRECTION('center_axis',(0.,0.,-1.));
#16600=DIRECTION('ref_axis',(1.,0.,0.));
#16601=DIRECTION('',(0.,-1.,0.));
#16602=DIRECTION('',(-1.,0.,0.));
#16603=DIRECTION('',(0.,-1.,0.));
#16604=DIRECTION('',(-1.,0.,0.));
#16605=DIRECTION('center_axis',(0.,0.,1.));
#16606=DIRECTION('ref_axis',(1.,0.,0.));
#16607=DIRECTION('center_axis',(0.,0.,1.));
#16608=DIRECTION('ref_axis',(1.,0.,0.));
#16609=DIRECTION('',(0.,-1.,0.));
#16610=DIRECTION('',(-1.,0.,0.));
#16611=DIRECTION('center_axis',(1.,0.,0.));
#16612=DIRECTION('ref_axis',(0.,-1.,0.));
#16613=DIRECTION('',(0.,0.,-1.));
#16614=DIRECTION('center_axis',(0.,0.,-1.));
#16615=DIRECTION('ref_axis',(-1.,0.,0.));
#16616=DIRECTION('',(0.,1.,0.));
#16617=DIRECTION('',(-1.,0.,0.));
#16618=DIRECTION('center_axis',(0.,0.,1.));
#16619=DIRECTION('ref_axis',(1.,0.,0.));
#16620=DIRECTION('',(-1.,0.,0.));
#16621=DIRECTION('',(0.,-1.,0.));
#16622=DIRECTION('center_axis',(-1.,0.,0.));
#16623=DIRECTION('ref_axis',(0.,1.,0.));
#16624=DIRECTION('',(0.,-1.,0.));
#16625=DIRECTION('',(0.,0.,-1.));
#16626=DIRECTION('center_axis',(0.,0.,1.));
#16627=DIRECTION('ref_axis',(1.,0.,0.));
#16628=DIRECTION('',(0.,1.,0.));
#16629=DIRECTION('',(1.,0.,0.));
#16630=DIRECTION('center_axis',(-1.,0.,0.));
#16631=DIRECTION('ref_axis',(0.,1.,0.));
#16632=DIRECTION('',(0.,1.,0.));
#16633=DIRECTION('',(0.,0.,-1.));
#16634=DIRECTION('center_axis',(0.,0.,1.));
#16635=DIRECTION('ref_axis',(1.,0.,0.));
#16636=DIRECTION('center_axis',(0.,0.,1.));
#16637=DIRECTION('ref_axis',(1.,0.,0.));
#16638=DIRECTION('',(1.,0.,0.));
#16639=DIRECTION('',(0.,-1.,0.));
#16640=DIRECTION('',(1.,0.,0.));
#16641=DIRECTION('',(0.,-1.,0.));
#16642=DIRECTION('center_axis',(0.,0.,-1.));
#16643=DIRECTION('ref_axis',(1.,0.,0.));
#16644=DIRECTION('',(-1.,0.,0.));
#16645=DIRECTION('center_axis',(-1.,0.,0.));
#16646=DIRECTION('ref_axis',(0.,1.,0.));
#16647=DIRECTION('',(0.,0.,-1.));
#16648=DIRECTION('',(0.,-1.,0.));
#16649=DIRECTION('center_axis',(0.,0.,1.));
#16650=DIRECTION('ref_axis',(1.,0.,0.));
#16651=DIRECTION('',(-1.,0.,0.));
#16652=DIRECTION('',(0.,1.,0.));
#16653=DIRECTION('center_axis',(0.,0.,1.));
#16654=DIRECTION('ref_axis',(1.,0.,0.));
#16655=DIRECTION('',(0.,1.,0.));
#16656=DIRECTION('',(1.,0.,0.));
#16657=DIRECTION('',(0.,-1.,0.));
#16658=DIRECTION('center_axis',(1.,0.,0.));
#16659=DIRECTION('ref_axis',(0.,-1.,0.));
#16660=DIRECTION('',(0.,0.,-1.));
#16661=DIRECTION('center_axis',(0.,0.,1.));
#16662=DIRECTION('ref_axis',(1.,0.,0.));
#16663=DIRECTION('',(0.,0.,-1.));
#16664=DIRECTION('',(0.,0.,1.));
#16665=DIRECTION('',(0.,0.,-1.));
#16666=DIRECTION('center_axis',(0.,0.,1.));
#16667=DIRECTION('ref_axis',(1.,0.,0.));
#16668=DIRECTION('',(0.,0.,1.));
#16669=DIRECTION('center_axis',(0.,0.,-1.));
#16670=DIRECTION('ref_axis',(1.,0.,0.));
#16671=DIRECTION('',(0.,0.,-1.));
#16672=DIRECTION('',(0.,0.,1.));
#16673=DIRECTION('',(0.,0.,-1.));
#16674=DIRECTION('center_axis',(0.,0.,1.));
#16675=DIRECTION('ref_axis',(1.,0.,0.));
#16676=DIRECTION('',(0.,0.,-1.));
#16677=DIRECTION('center_axis',(0.,0.,-1.));
#16678=DIRECTION('ref_axis',(1.,0.,0.));
#16679=DIRECTION('center_axis',(0.,0.,1.));
#16680=DIRECTION('ref_axis',(1.,0.,0.));
#16681=DIRECTION('',(0.,0.,1.));
#16682=DIRECTION('center_axis',(0.,1.,0.));
#16683=DIRECTION('ref_axis',(1.,0.,0.));
#16684=DIRECTION('',(0.,0.,-1.));
#16685=DIRECTION('',(0.,0.,-1.));
#16686=DIRECTION('center_axis',(0.,1.,0.));
#16687=DIRECTION('ref_axis',(1.,0.,0.));
#16688=DIRECTION('',(0.,0.,-1.));
#16689=DIRECTION('center_axis',(-1.,0.,0.));
#16690=DIRECTION('ref_axis',(0.,1.,0.));
#16691=DIRECTION('center_axis',(0.,-1.,0.));
#16692=DIRECTION('ref_axis',(-1.,0.,0.));
#16693=DIRECTION('',(0.,0.,-1.));
#16694=DIRECTION('center_axis',(0.,-1.,0.));
#16695=DIRECTION('ref_axis',(-1.,0.,0.));
#16696=DIRECTION('',(-1.,0.,0.));
#16697=DIRECTION('',(0.,0.,-1.));
#16698=DIRECTION('',(0.,0.,-1.));
#16699=DIRECTION('center_axis',(1.,0.,0.));
#16700=DIRECTION('ref_axis',(0.,-1.,0.));
#16701=DIRECTION('',(0.,-1.,0.));
#16702=DIRECTION('center_axis',(0.,-1.,0.));
#16703=DIRECTION('ref_axis',(-1.,0.,0.));
#16704=DIRECTION('',(0.,0.,-1.));
#16705=DIRECTION('',(0.,0.,-1.));
#16706=DIRECTION('',(-1.,0.,0.));
#16707=DIRECTION('center_axis',(0.,0.,-1.));
#16708=DIRECTION('ref_axis',(-1.,0.,0.));
#16709=DIRECTION('center_axis',(0.,0.,-1.));
#16710=DIRECTION('ref_axis',(1.,0.,0.));
#16711=DIRECTION('',(0.,-1.,0.));
#16712=DIRECTION('',(1.,0.,0.));
#16713=DIRECTION('center_axis',(0.,0.,-1.));
#16714=DIRECTION('ref_axis',(1.,0.,0.));
#16715=DIRECTION('center_axis',(1.,0.,0.));
#16716=DIRECTION('ref_axis',(0.,-1.,0.));
#16717=DIRECTION('',(0.,0.,1.));
#16718=DIRECTION('',(0.,1.,0.));
#16719=DIRECTION('',(0.,0.,1.));
#16720=DIRECTION('',(0.,-1.,0.));
#16721=DIRECTION('',(0.,0.,-1.));
#16722=DIRECTION('',(0.,1.,0.));
#16723=DIRECTION('',(0.,0.,-1.));
#16724=DIRECTION('',(0.,0.,-1.));
#16725=DIRECTION('center_axis',(0.,1.,0.));
#16726=DIRECTION('ref_axis',(1.,0.,0.));
#16727=DIRECTION('',(0.,0.,1.));
#16728=DIRECTION('center_axis',(0.,-1.,0.));
#16729=DIRECTION('ref_axis',(-1.,0.,0.));
#16730=DIRECTION('',(0.,0.,1.));
#16731=DIRECTION('',(-1.,0.,0.));
#16732=DIRECTION('',(0.,0.,-1.));
#16733=DIRECTION('center_axis',(-1.,0.,0.));
#16734=DIRECTION('ref_axis',(0.,1.,0.));
#16735=DIRECTION('',(0.,0.,-1.));
#16736=DIRECTION('',(0.,1.,0.));
#16737=DIRECTION('',(0.,0.,-1.));
#16738=DIRECTION('',(0.,1.,0.));
#16739=DIRECTION('',(0.,0.,1.));
#16740=DIRECTION('',(0.,-1.,0.));
#16741=DIRECTION('',(0.,0.,1.));
#16742=DIRECTION('',(0.,1.,0.));
#16743=DIRECTION('',(0.,0.,-1.));
#16744=DIRECTION('',(0.,-1.,0.));
#16745=DIRECTION('center_axis',(0.,1.,0.));
#16746=DIRECTION('ref_axis',(1.,0.,0.));
#16747=DIRECTION('',(0.,0.,-1.));
#16748=DIRECTION('',(1.,0.,0.));
#16749=DIRECTION('',(1.,0.,0.));
#16750=DIRECTION('center_axis',(0.,0.,-1.));
#16751=DIRECTION('ref_axis',(-1.,0.,0.));
#16752=DIRECTION('center_axis',(0.,0.,-1.));
#16753=DIRECTION('ref_axis',(1.,0.,0.));
#16754=DIRECTION('center_axis',(0.,-1.,0.));
#16755=DIRECTION('ref_axis',(-1.,0.,0.));
#16756=DIRECTION('',(1.,0.,0.));
#16757=DIRECTION('',(-1.,0.,0.));
#16758=DIRECTION('center_axis',(0.,0.,1.));
#16759=DIRECTION('ref_axis',(1.,0.,0.));
#16760=DIRECTION('',(-1.,0.,0.));
#16761=DIRECTION('',(0.,1.,0.));
#16762=DIRECTION('center_axis',(0.,-1.,0.));
#16763=DIRECTION('ref_axis',(-1.,0.,0.));
#16764=DIRECTION('',(0.,0.,-1.));
#16765=DIRECTION('center_axis',(0.,0.,1.));
#16766=DIRECTION('ref_axis',(1.,0.,0.));
#16767=DIRECTION('',(0.,0.,-1.));
#16768=DIRECTION('center_axis',(0.,0.,1.));
#16769=DIRECTION('ref_axis',(1.,0.,0.));
#16770=DIRECTION('center_axis',(0.,0.,1.));
#16771=DIRECTION('ref_axis',(1.,0.,0.));
#16772=DIRECTION('center_axis',(0.,-1.,0.));
#16773=DIRECTION('ref_axis',(-1.,0.,0.));
#16774=DIRECTION('',(-1.,0.,0.));
#16775=DIRECTION('',(0.,0.,-1.));
#16776=DIRECTION('center_axis',(0.,0.,1.));
#16777=DIRECTION('ref_axis',(1.,0.,0.));
#16778=DIRECTION('',(1.,0.,0.));
#16779=DIRECTION('',(0.,-1.,0.));
#16780=DIRECTION('center_axis',(0.,0.,1.));
#16781=DIRECTION('ref_axis',(1.,0.,0.));
#16782=DIRECTION('',(0.,1.,0.));
#16783=DIRECTION('',(1.,0.,0.));
#16784=DIRECTION('center_axis',(0.,-1.,0.));
#16785=DIRECTION('ref_axis',(-1.,0.,0.));
#16786=DIRECTION('',(-1.,0.,0.));
#16787=DIRECTION('center_axis',(0.,0.,-1.));
#16788=DIRECTION('ref_axis',(-1.,0.,0.));
#16789=DIRECTION('',(1.,0.,0.));
#16790=DIRECTION('',(0.,1.,0.));
#16791=DIRECTION('',(0.,1.,0.));
#16792=DIRECTION('center_axis',(0.,1.,0.));
#16793=DIRECTION('ref_axis',(1.,0.,0.));
#16794=DIRECTION('',(-1.,0.,0.));
#16795=DIRECTION('center_axis',(0.,0.,-1.));
#16796=DIRECTION('ref_axis',(-1.,0.,0.));
#16797=DIRECTION('',(0.,-1.,0.));
#16798=DIRECTION('',(0.,-1.,0.));
#16799=DIRECTION('',(1.,0.,0.));
#16800=DIRECTION('center_axis',(0.,0.,1.));
#16801=DIRECTION('ref_axis',(1.,0.,0.));
#16802=DIRECTION('',(-1.,0.,0.));
#16803=DIRECTION('',(0.,1.,0.));
#16804=DIRECTION('',(1.,0.,0.));
#16805=DIRECTION('center_axis',(0.,1.,0.));
#16806=DIRECTION('ref_axis',(1.,0.,0.));
#16807=DIRECTION('center_axis',(0.,0.,1.));
#16808=DIRECTION('ref_axis',(1.,0.,0.));
#16809=DIRECTION('',(1.,0.,0.));
#16810=DIRECTION('',(0.,-1.,0.));
#16811=DIRECTION('center_axis',(1.,0.,0.));
#16812=DIRECTION('ref_axis',(0.,-1.,0.));
#16813=DIRECTION('center_axis',(1.,0.,0.));
#16814=DIRECTION('ref_axis',(0.,-1.,0.));
#16815=DIRECTION('',(0.,0.,-1.));
#16816=DIRECTION('center_axis',(0.,1.,0.));
#16817=DIRECTION('ref_axis',(1.,0.,0.));
#16818=DIRECTION('center_axis',(-1.,0.,0.));
#16819=DIRECTION('ref_axis',(0.,1.,0.));
#16820=DIRECTION('center_axis',(0.,1.,0.));
#16821=DIRECTION('ref_axis',(1.,0.,0.));
#16822=DIRECTION('',(0.,0.,-1.));
#16823=DIRECTION('center_axis',(-1.,0.,0.));
#16824=DIRECTION('ref_axis',(0.,1.,0.));
#16825=DIRECTION('center_axis',(0.,0.,1.));
#16826=DIRECTION('ref_axis',(-1.,0.,0.));
#16827=DIRECTION('center_axis',(0.,0.,1.));
#16828=DIRECTION('ref_axis',(-1.,0.,0.));
#16829=DIRECTION('',(0.,0.,1.));
#16830=DIRECTION('center_axis',(0.,0.,1.));
#16831=DIRECTION('ref_axis',(-1.,0.,0.));
#16832=DIRECTION('center_axis',(0.,0.,1.));
#16833=DIRECTION('ref_axis',(-1.,0.,0.));
#16834=DIRECTION('center_axis',(0.,0.,1.));
#16835=DIRECTION('ref_axis',(1.,0.,0.));
#18710=CARTESIAN_POINT('',(0.,0.,0.));
#18711=CARTESIAN_POINT('Origin',(-92.,-24.,5.));
#18712=CARTESIAN_POINT('',(-94.5134954281454,-23.9997257032743,1.38741669750802));
#18713=CARTESIAN_POINT('',(-94.5156258041287,-24.0035321038279,1.11258330249198));
#18714=CARTESIAN_POINT('',(-94.5175,-24.,5.));
#18715=CARTESIAN_POINT('',(-93.913465996665,-22.364012796625,0.999999999999999));
#18716=CARTESIAN_POINT('Ctrl Pts',(-94.5156258041287,-24.0035321038279,
1.11258330249198));
#18717=CARTESIAN_POINT('Ctrl Pts',(-94.5104632893492,-23.410913677985,1.07505553499465));
#18718=CARTESIAN_POINT('Ctrl Pts',(-94.299221828084,-22.8151964396956,1.03752776749732));
#18719=CARTESIAN_POINT('Ctrl Pts',(-93.913465996665,-22.364012796625,0.999999999999996));
#18720=CARTESIAN_POINT('',(-94.5175,-24.,1.));
#18721=CARTESIAN_POINT('Origin',(-92.,-24.,1.));
#18722=CARTESIAN_POINT('',(-94.5175,-24.,0.));
#18723=CARTESIAN_POINT('',(-94.5175,-24.,5.));
#18724=CARTESIAN_POINT('Origin',(-92.,-24.,0.));
#18725=CARTESIAN_POINT('',(-90.0828967253639,-22.3614656719992,1.));
#18726=CARTESIAN_POINT('Origin',(-92.,-24.,1.));
#18727=CARTESIAN_POINT('Ctrl Pts',(-90.0828882653787,-22.3614597476137,
1.));
#18728=CARTESIAN_POINT('Ctrl Pts',(-90.6060429859409,-21.7523041107177,
1.05098091535882));
#18729=CARTESIAN_POINT('Ctrl Pts',(-91.4465812877835,-21.4121723295192,
1.10196183071765));
#18730=CARTESIAN_POINT('Ctrl Pts',(-92.2457357736239,-21.49051470028,1.15294274607647));
#18731=CARTESIAN_POINT('Ctrl Pts',(-93.0712273934265,-21.5714389416932,
1.20560380115935));
#18732=CARTESIAN_POINT('Ctrl Pts',(-93.8525625390091,-22.0988745222663,
1.25826485624223));
#18733=CARTESIAN_POINT('Ctrl Pts',(-94.2358880111547,-22.8341462678707,
1.31092591132511));
#18734=CARTESIAN_POINT('Ctrl Pts',(-94.4214828919903,-23.1901431476069,
1.33642284005274));
#18735=CARTESIAN_POINT('Ctrl Pts',(-94.5137759227878,-23.5948612017176,
1.36191976878038));
#18736=CARTESIAN_POINT('Ctrl Pts',(-94.5134954281454,-23.9997257032743,
1.38741669750802));
#18737=CARTESIAN_POINT('Origin',(-92.,-24.,5.));
#18738=CARTESIAN_POINT('',(-94.5187355654992,-24.0021096152222,2.38741669750802));
#18739=CARTESIAN_POINT('',(-94.5214126870217,-23.9993544610189,2.11258330249198));
#18740=CARTESIAN_POINT('',(-94.5175,-24.,5.));
#18741=CARTESIAN_POINT('Ctrl Pts',(-94.5214126870217,-23.9993544610189,
2.11258330249198));
#18742=CARTESIAN_POINT('Ctrl Pts',(-94.5215323520691,-23.9641713906795,
2.11034958724147));
#18743=CARTESIAN_POINT('Ctrl Pts',(-94.5208590695048,-23.9289930573579,
2.10811587199095));
#18744=CARTESIAN_POINT('Ctrl Pts',(-94.5193785186672,-23.8938487960073,
2.10588215674044));
#18745=CARTESIAN_POINT('Ctrl Pts',(-94.4844737253228,-23.0653036703884,
2.05322110165756));
#18746=CARTESIAN_POINT('Ctrl Pts',(-94.0008841105951,-22.25569596213,2.00056004657469));
#18747=CARTESIAN_POINT('Ctrl Pts',(-93.2879127216155,-21.8321129915859,
1.94789899149181));
#18748=CARTESIAN_POINT('Ctrl Pts',(-92.5749413326359,-21.4085300210418,
1.89523793640893));
#18749=CARTESIAN_POINT('Ctrl Pts',(-91.6325881694045,-21.3709717882121,
1.84257688132605));
#18750=CARTESIAN_POINT('Ctrl Pts',(-90.8882532181424,-21.7366423255222,
1.78991582624317));
#18751=CARTESIAN_POINT('Ctrl Pts',(-90.1439182668804,-22.1023128628323,
1.73725477116029));
#18752=CARTESIAN_POINT('Ctrl Pts',(-89.5976015275876,-22.8712121702823,
1.68459371607741));
#18753=CARTESIAN_POINT('Ctrl Pts',(-89.4970123488694,-23.6942825335227,
1.63193266099454));
#18754=CARTESIAN_POINT('Ctrl Pts',(-89.3964231701512,-24.5173528967631,
1.57927160591166));
#18755=CARTESIAN_POINT('Ctrl Pts',(-89.7415615520075,-25.3945943157939,
1.52661055082878));
#18756=CARTESIAN_POINT('Ctrl Pts',(-90.3760119861909,-25.9288768514157,
1.4739494957459));
#18757=CARTESIAN_POINT('Ctrl Pts',(-91.0104624203743,-26.4631593870376,
1.42128844066303));
#18758=CARTESIAN_POINT('Ctrl Pts',(-91.9342249068849,-26.6544830392504,
1.36862738558015));
#18759=CARTESIAN_POINT('Ctrl Pts',(-92.7281293260075,-26.4146105531457,
1.31596633049727));
#18760=CARTESIAN_POINT('Ctrl Pts',(-93.52203374513,-26.1747380670411,1.26330527541439));
#18761=CARTESIAN_POINT('Ctrl Pts',(-94.1860800968645,-25.503669442619,1.21064422033151));
#18762=CARTESIAN_POINT('Ctrl Pts',(-94.4192666807451,-24.7092696340464,
1.15798316524863));
#18763=CARTESIAN_POINT('Ctrl Pts',(-94.4862778644254,-24.4809817514334,
1.14284987766308));
#18764=CARTESIAN_POINT('Ctrl Pts',(-94.5177076178372,-24.2425088846187,
1.12771659007753));
#18765=CARTESIAN_POINT('Ctrl Pts',(-94.5156258041287,-24.0035321038279,
1.11258330249198));
#18766=CARTESIAN_POINT('Ctrl Pts',(-94.5134954281454,-23.9997257032743,
1.38741669750802));
#18767=CARTESIAN_POINT('Ctrl Pts',(-94.5131965924704,-24.4310635555512,
1.41458082386326));
#18768=CARTESIAN_POINT('Ctrl Pts',(-94.4078219950606,-24.8625676332891,
1.4417449502185));
#18769=CARTESIAN_POINT('Ctrl Pts',(-94.1982523776868,-25.2354979308672,
1.46890907657374));
#18770=CARTESIAN_POINT('Ctrl Pts',(-93.7919754733646,-25.9584699376238,
1.52157013165662));
#18771=CARTESIAN_POINT('Ctrl Pts',(-92.9941058660117,-26.4613060405014,
1.5742311867395));
#18772=CARTESIAN_POINT('Ctrl Pts',(-92.1666097958722,-26.5160870716528,
1.62689224182237));
#18773=CARTESIAN_POINT('Ctrl Pts',(-91.3391137257328,-26.5708681028041,
1.67955329690525));
#18774=CARTESIAN_POINT('Ctrl Pts',(-90.4819911928069,-26.1775940622292,
1.73221435198813));
#18775=CARTESIAN_POINT('Ctrl Pts',(-89.9839037459974,-25.5145599501885,
1.78487540707101));
#18776=CARTESIAN_POINT('Ctrl Pts',(-89.4858162991878,-24.8515258381478,
1.83753646215389));
#18777=CARTESIAN_POINT('Ctrl Pts',(-89.3467639384946,-23.9187316546413,
1.89019751723676));
#18778=CARTESIAN_POINT('Ctrl Pts',(-89.6298377538243,-23.1392455882325,
1.94285857231964));
#18779=CARTESIAN_POINT('Ctrl Pts',(-89.9129115691541,-22.3597595218238,
1.99551962740252));
#18780=CARTESIAN_POINT('Ctrl Pts',(-90.6181115605066,-21.7335815725127,
2.0481806824854));
#18781=CARTESIAN_POINT('Ctrl Pts',(-91.425603556166,-21.5446793850464,2.10084173756828));
#18782=CARTESIAN_POINT('Ctrl Pts',(-92.2330955518254,-21.35577719758,2.15350279265115));
#18783=CARTESIAN_POINT('Ctrl Pts',(-93.1428795517915,-21.6041507719583,
2.20616384773403));
#18784=CARTESIAN_POINT('Ctrl Pts',(-93.7423598115282,-22.1771656715372,
2.25882490281691));
#18785=CARTESIAN_POINT('Ctrl Pts',(-94.2303120712523,-22.6435762172788,
2.30168883438062));
#18786=CARTESIAN_POINT('Ctrl Pts',(-94.5126791039229,-23.3250710559231,
2.34455276594432));
#18787=CARTESIAN_POINT('Ctrl Pts',(-94.5187355654992,-24.0021096152222,
2.38741669750802));
#18788=CARTESIAN_POINT('Origin',(-92.,-24.,5.));
#18789=CARTESIAN_POINT('',(-94.5197285159004,-23.9981710495135,3.38741669750802));
#18790=CARTESIAN_POINT('',(-94.5145914825341,-23.9984414286209,3.11258330249198));
#18791=CARTESIAN_POINT('',(-94.5175,-24.,5.));
#18792=CARTESIAN_POINT('Ctrl Pts',(-94.5145914825341,-23.9984414286209,
3.11258330249198));
#18793=CARTESIAN_POINT('Ctrl Pts',(-94.5163706169191,-23.687546359978,3.0929825844054));
#18794=CARTESIAN_POINT('Ctrl Pts',(-94.4629229514308,-23.3772412892129,
3.07338186631883));
#18795=CARTESIAN_POINT('Ctrl Pts',(-94.3514583308843,-23.0894032152641,
3.05378114823225));
#18796=CARTESIAN_POINT('Ctrl Pts',(-94.0519874392331,-22.3160715138328,
3.00112009314937));
#18797=CARTESIAN_POINT('Ctrl Pts',(-93.3337325490401,-21.7049134175565,
2.94845903806649));
#18798=CARTESIAN_POINT('Ctrl Pts',(-92.52243433036,-21.5330984014484,2.89579798298361));
#18799=CARTESIAN_POINT('Ctrl Pts',(-91.7111361116799,-21.3612833853403,
2.84313692790073));
#18800=CARTESIAN_POINT('Ctrl Pts',(-90.8067945645125,-21.6288114494004,
2.79047587281786));
#18801=CARTESIAN_POINT('Ctrl Pts',(-90.219544382578,-22.2143564031656,2.73781481773498));
#18802=CARTESIAN_POINT('Ctrl Pts',(-89.6322942006435,-22.7999013569308,
2.6851537626521));
#18803=CARTESIAN_POINT('Ctrl Pts',(-89.3621353839418,-23.703463200401,2.63249270756922));
#18804=CARTESIAN_POINT('Ctrl Pts',(-89.5315888137356,-24.515256413142,2.57983165248635));
#18805=CARTESIAN_POINT('Ctrl Pts',(-89.7010422435293,-25.3270496258829,
2.52717059740347));
#18806=CARTESIAN_POINT('Ctrl Pts',(-90.3101079198185,-26.0470742078947,
2.47450954232059));
#18807=CARTESIAN_POINT('Ctrl Pts',(-91.0825657012674,-26.3487965351803,
2.42184848723771));
#18808=CARTESIAN_POINT('Ctrl Pts',(-91.8550234827163,-26.6505188624658,
2.36918743215483));
#18809=CARTESIAN_POINT('Ctrl Pts',(-92.7908733693248,-26.5339389350252,
2.31652637707195));
#18810=CARTESIAN_POINT('Ctrl Pts',(-93.4656883266487,-26.0519076998153,
2.26386532198908));
#18811=CARTESIAN_POINT('Ctrl Pts',(-94.1118797697061,-25.5903227036642,
2.21343798215671));
#18812=CARTESIAN_POINT('Ctrl Pts',(-94.5187111833227,-24.7936314593702,
2.16301064232435));
#18813=CARTESIAN_POINT('Ctrl Pts',(-94.5214126870217,-23.9993544610189,
2.11258330249198));
#18814=CARTESIAN_POINT('Ctrl Pts',(-94.5187355654992,-24.0021096152222,
2.38741669750802));
#18815=CARTESIAN_POINT('Ctrl Pts',(-94.5201198506077,-24.1568558120997,
2.3972138210272));
#18816=CARTESIAN_POINT('Ctrl Pts',(-94.5070693393431,-24.3113692075874,
2.40701094454637));
#18817=CARTESIAN_POINT('Ctrl Pts',(-94.4787395411231,-24.4630283942082,
2.41680806806555));
#18818=CARTESIAN_POINT('Ctrl Pts',(-94.3264624914741,-25.2782199925207,
2.46946912314842));
#18819=CARTESIAN_POINT('Ctrl Pts',(-93.7327318726689,-26.0109469643662,
2.5221301782313));
#18820=CARTESIAN_POINT('Ctrl Pts',(-92.9668162894688,-26.3289068537565,
2.57479123331418));
#18821=CARTESIAN_POINT('Ctrl Pts',(-92.2009007062687,-26.6468667431468,
2.62745228839706));
#18822=CARTESIAN_POINT('Ctrl Pts',(-91.2628001586737,-26.5500595500819,
2.68011334347994));
#18823=CARTESIAN_POINT('Ctrl Pts',(-90.5779584534227,-26.0823881414071,
2.73277439856282));
#18824=CARTESIAN_POINT('Ctrl Pts',(-89.8931167481717,-25.6147167327323,
2.78543545364569));
#18825=CARTESIAN_POINT('Ctrl Pts',(-89.4615338852647,-24.7761811084476,
2.83809650872857));
#18826=CARTESIAN_POINT('Ctrl Pts',(-89.4789404507956,-23.9470718995605,
2.89075756381145));
#18827=CARTESIAN_POINT('Ctrl Pts',(-89.4963470163265,-23.1179626906734,
2.94341861889433));
#18828=CARTESIAN_POINT('Ctrl Pts',(-89.9627430102955,-22.2982798971839,
2.99607967397721));
#18829=CARTESIAN_POINT('Ctrl Pts',(-90.6666096977841,-21.8597634515608,
3.04874072906008));
#18830=CARTESIAN_POINT('Ctrl Pts',(-91.3704763852727,-21.4212470059377,
3.10140178414296));
#18831=CARTESIAN_POINT('Ctrl Pts',(-92.311813766281,-21.363896908181,3.15406283922584));
#18832=CARTESIAN_POINT('Ctrl Pts',(-93.0637093676529,-21.7137225058316,
3.20672389430872));
#18833=CARTESIAN_POINT('Ctrl Pts',(-93.8156049690249,-22.0635481034822,
3.2593849493916));
#18834=CARTESIAN_POINT('Ctrl Pts',(-94.3780587907605,-22.8205493965401,
3.31204600447447));
#18835=CARTESIAN_POINT('Ctrl Pts',(-94.4959883797686,-23.641413330862,3.36470705955735));
#18836=CARTESIAN_POINT('Ctrl Pts',(-94.5129404282089,-23.7594102245555,
3.37227693887424));
#18837=CARTESIAN_POINT('Ctrl Pts',(-94.5207071577179,-23.8787267284854,
3.37984681819113));
#18838=CARTESIAN_POINT('Ctrl Pts',(-94.5197285159004,-23.9981710495135,
3.38741669750802));
#18839=CARTESIAN_POINT('Origin',(-92.,-24.,5.));
#18840=CARTESIAN_POINT('',(-94.5135839828142,-23.9996457834291,4.38741669750802));
#18841=CARTESIAN_POINT('',(-94.51602550603,-24.0021063693209,4.11258330249198));
#18842=CARTESIAN_POINT('',(-94.5175,-24.,5.));
#18843=CARTESIAN_POINT('Ctrl Pts',(-94.51602550603,-24.0021063693209,4.11258330249198));
#18844=CARTESIAN_POINT('Ctrl Pts',(-94.5113088734142,-23.4165891850021,
4.07561558156934));
#18845=CARTESIAN_POINT('Ctrl Pts',(-94.30740600999,-22.828109419245,4.0386478606467));
#18846=CARTESIAN_POINT('Ctrl Pts',(-93.9337853550358,-22.381662326268,4.00168013972405));
#18847=CARTESIAN_POINT('Ctrl Pts',(-93.4015573085243,-21.7456919616342,
3.94901908464117));
#18848=CARTESIAN_POINT('Ctrl Pts',(-92.5249308580447,-21.3979402061153,
3.8963580295583));
#18849=CARTESIAN_POINT('Ctrl Pts',(-91.7014710569733,-21.4961183997274,
3.84369697447542));
#18850=CARTESIAN_POINT('Ctrl Pts',(-90.8780112559018,-21.5942965933395,
3.79103591939254));
#18851=CARTESIAN_POINT('Ctrl Pts',(-90.1077181042387,-22.1384047360825,
3.73837486430966));
#18852=CARTESIAN_POINT('Ctrl Pts',(-89.7399326972187,-22.8816805318428,
3.68571380922678));
#18853=CARTESIAN_POINT('Ctrl Pts',(-89.3721472901988,-23.624956327603,3.63305275414391));
#18854=CARTESIAN_POINT('Ctrl Pts',(-89.406869627822,-24.5673997763804,3.58039169906103));
#18855=CARTESIAN_POINT('Ctrl Pts',(-89.8283525270324,-25.2815966241557,
3.52773064397815));
#18856=CARTESIAN_POINT('Ctrl Pts',(-90.2498354262427,-25.9957934719311,
3.47506958889527));
#18857=CARTESIAN_POINT('Ctrl Pts',(-91.0580788870401,-26.4817437187043,
3.42240853381239));
#18858=CARTESIAN_POINT('Ctrl Pts',(-91.8865307275916,-26.5190607694894,
3.36974747872952));
#18859=CARTESIAN_POINT('Ctrl Pts',(-92.7149825681431,-26.5563778202744,
3.31708642364664));
#18860=CARTESIAN_POINT('Ctrl Pts',(-93.5636427884488,-26.1450616750713,
3.26442536856376));
#18861=CARTESIAN_POINT('Ctrl Pts',(-94.0476294520469,-25.4716509491765,
3.21176431348088));
#18862=CARTESIAN_POINT('Ctrl Pts',(-94.3514737668842,-25.0488871914059,
3.17870397648458));
#18863=CARTESIAN_POINT('Ctrl Pts',(-94.5115906341944,-24.5228250606093,
3.14564363948828));
#18864=CARTESIAN_POINT('Ctrl Pts',(-94.5145914825341,-23.9984414286209,
3.11258330249198));
#18865=CARTESIAN_POINT('Ctrl Pts',(-94.5197285159004,-23.9981710495135,
3.38741669750802));
#18866=CARTESIAN_POINT('Ctrl Pts',(-94.5138990821199,-24.7096599185249,
3.43250787327401));
#18867=CARTESIAN_POINT('Ctrl Pts',(-94.1977684432012,-25.4256839637041,
3.47759904904));
#18868=CARTESIAN_POINT('Ctrl Pts',(-93.664320715776,-25.8943544806311,3.52269022480599));
#18869=CARTESIAN_POINT('Ctrl Pts',(-93.0413181064947,-26.4417051204924,
3.57535127988887));
#18870=CARTESIAN_POINT('Ctrl Pts',(-92.1219075316514,-26.6516798246292,
3.62801233497174));
#18871=CARTESIAN_POINT('Ctrl Pts',(-91.3230573666226,-26.4290514695956,
3.68067339005462));
#18872=CARTESIAN_POINT('Ctrl Pts',(-90.5242072015938,-26.206423114562,3.7333344451375));
#18873=CARTESIAN_POINT('Ctrl Pts',(-89.8459174463795,-25.5511917003581,
3.78599550022038));
#18874=CARTESIAN_POINT('Ctrl Pts',(-89.5958040861176,-24.7605158612689,
3.83865655530326));
#18875=CARTESIAN_POINT('Ctrl Pts',(-89.3456907258557,-23.9698400221797,
3.89131761038613));
#18876=CARTESIAN_POINT('Ctrl Pts',(-89.5237537605462,-23.0437197582053,
3.94397866546901));
#18877=CARTESIAN_POINT('Ctrl Pts',(-90.0492385624731,-22.4021664114935,
3.99663972055189));
#18878=CARTESIAN_POINT('Ctrl Pts',(-90.5747233644,-21.7606130647817,4.04930077563477));
#18879=CARTESIAN_POINT('Ctrl Pts',(-91.4476299335634,-21.4036266353327,
4.10196183071765));
#18880=CARTESIAN_POINT('Ctrl Pts',(-92.2720802450577,-21.4931065626282,
4.15462288580053));
#18881=CARTESIAN_POINT('Ctrl Pts',(-93.096530556552,-21.5825864899238,4.2072839408834));
#18882=CARTESIAN_POINT('Ctrl Pts',(-93.8725246103771,-22.1185327739639,
4.25994499596628));
#18883=CARTESIAN_POINT('Ctrl Pts',(-94.2481358593184,-22.8578846277675,
4.31260605104916));
#18884=CARTESIAN_POINT('Ctrl Pts',(-94.4260011420294,-23.2079940211105,
4.33754293320211));
#18885=CARTESIAN_POINT('Ctrl Pts',(-94.5140862159014,-23.6037142506574,
4.36247981535507));
#18886=CARTESIAN_POINT('Ctrl Pts',(-94.5135839828142,-23.9996457834291,
4.38741669750802));
#18887=CARTESIAN_POINT('Origin',(-92.,-24.,5.));
#18888=CARTESIAN_POINT('',(-94.5184743499735,-24.0021560918536,5.38741669750802));
#18889=CARTESIAN_POINT('',(-94.5215003759084,-23.999522240299,5.11258330249198));
#18890=CARTESIAN_POINT('',(-94.5175,-24.,5.));
#18891=CARTESIAN_POINT('Ctrl Pts',(-94.5215003759084,-23.999522240299,5.11258330249198));
#18892=CARTESIAN_POINT('Ctrl Pts',(-94.5215696550139,-23.9731625365728,
5.11090963381615));
#18893=CARTESIAN_POINT('Ctrl Pts',(-94.5211916947533,-23.9468048672736,
5.10923596514032));
#18894=CARTESIAN_POINT('Ctrl Pts',(-94.5203603409136,-23.9204615063421,
5.10756229646449));
#18895=CARTESIAN_POINT('Ctrl Pts',(-94.4942022542029,-23.0915822896134,
5.05490124138162));
#18896=CARTESIAN_POINT('Ctrl Pts',(-94.0191794168034,-22.2768685179764,
5.00224018629874));
#18897=CARTESIAN_POINT('Ctrl Pts',(-93.3107227922662,-21.8458067909395,
4.94957913121586));
#18898=CARTESIAN_POINT('Ctrl Pts',(-92.602266167729,-21.4147450639025,4.89691807613299));
#18899=CARTESIAN_POINT('Ctrl Pts',(-91.660375756054,-21.3673353814657,4.84425702105011));
#18900=CARTESIAN_POINT('Ctrl Pts',(-90.9122149332711,-21.7250788434924,
4.79159596596723));
#18901=CARTESIAN_POINT('Ctrl Pts',(-90.1640541104882,-22.0828223055191,
4.73893491088435));
#18902=CARTESIAN_POINT('Ctrl Pts',(-89.6096228765974,-22.8457189120093,
4.68627385580147));
#18903=CARTESIAN_POINT('Ctrl Pts',(-89.5003652582015,-23.667782032718,4.63361280071859));
#18904=CARTESIAN_POINT('Ctrl Pts',(-89.3911076398056,-24.4898451534267,
4.58095174563571));
#18905=CARTESIAN_POINT('Ctrl Pts',(-89.7270236369045,-25.3710747883538,
4.52829069055284));
#18906=CARTESIAN_POINT('Ctrl Pts',(-90.3557696119043,-25.9118182580198,
4.47562963546996));
#18907=CARTESIAN_POINT('Ctrl Pts',(-90.9845155869042,-26.4525617276857,
4.42296858038708));
#18908=CARTESIAN_POINT('Ctrl Pts',(-91.906091539805,-26.6528190320905,4.3703075253042));
#18909=CARTESIAN_POINT('Ctrl Pts',(-92.7025470485768,-26.4217700679435,
4.31764647022132));
#18910=CARTESIAN_POINT('Ctrl Pts',(-93.4990025573485,-26.1907211037965,
4.26498541513844));
#18911=CARTESIAN_POINT('Ctrl Pts',(-94.1703376219912,-25.5283658710978,
4.21232436005557));
#18912=CARTESIAN_POINT('Ctrl Pts',(-94.4120903330409,-24.7350937678741,
4.15966330497269));
#18913=CARTESIAN_POINT('Ctrl Pts',(-94.4841342006139,-24.4986935632772,
4.14396997081245));
#18914=CARTESIAN_POINT('Ctrl Pts',(-94.5180277850427,-24.250666913513,4.12827663665222));
#18915=CARTESIAN_POINT('Ctrl Pts',(-94.51602550603,-24.0021063693209,4.11258330249198));
#18916=CARTESIAN_POINT('Ctrl Pts',(-94.5135839828142,-23.9996457834291,
4.38741669750802));
#18917=CARTESIAN_POINT('Ctrl Pts',(-94.5130256132123,-24.4398320992502,
4.41514087043795));
#18918=CARTESIAN_POINT('Ctrl Pts',(-94.4029696961734,-24.8802795945301,
4.44286504336787));
#18919=CARTESIAN_POINT('Ctrl Pts',(-94.185055515175,-25.2586003180437,4.47058921629779));
#18920=CARTESIAN_POINT('Ctrl Pts',(-93.7711354780326,-25.9772067309494,
4.52325027138067));
#18921=CARTESIAN_POINT('Ctrl Pts',(-92.9680669596902,-26.4716621331935,
4.57591132646355));
#18922=CARTESIAN_POINT('Ctrl Pts',(-92.140055238289,-26.5177225612861,4.62857238154643));
#18923=CARTESIAN_POINT('Ctrl Pts',(-91.3120435168878,-26.5637829893786,
4.68123343662931));
#18924=CARTESIAN_POINT('Ctrl Pts',(-90.4590885924279,-26.1614484433196,
4.73389449171219));
#18925=CARTESIAN_POINT('Ctrl Pts',(-89.9680200798161,-25.493184506096,4.78655554679507));
#18926=CARTESIAN_POINT('Ctrl Pts',(-89.4769515672043,-24.8249205688725,
4.83921660187794));
#18927=CARTESIAN_POINT('Ctrl Pts',(-89.3477694664407,-23.8907272404844,
4.89187765696082));
#18928=CARTESIAN_POINT('Ctrl Pts',(-89.6390600648162,-23.1142771383271,
4.9445387120437));
#18929=CARTESIAN_POINT('Ctrl Pts',(-89.9303506631918,-22.3378270361698,
4.99719976712657));
#18930=CARTESIAN_POINT('Ctrl Pts',(-90.6421139607066,-21.7191201602431,
5.04986082220945));
#18931=CARTESIAN_POINT('Ctrl Pts',(-91.4515531549517,-21.5387506376962,
5.10252187729233));
#18932=CARTESIAN_POINT('Ctrl Pts',(-92.2609923491968,-21.3583811151493,
5.15518293237521));
#18933=CARTESIAN_POINT('Ctrl Pts',(-93.1681074401722,-21.6163489459821,
5.20784398745809));
#18934=CARTESIAN_POINT('Ctrl Pts',(-93.7615062532209,-22.1956613164021,
5.26050504254097));
#18935=CARTESIAN_POINT('Ctrl Pts',(-94.2381977114593,-22.6610367983859,
5.30280892752999));
#18936=CARTESIAN_POINT('Ctrl Pts',(-94.5124388592754,-23.3337853316565,
5.34511281251901));
#18937=CARTESIAN_POINT('Ctrl Pts',(-94.5184743499735,-24.0021560918536,
5.38741669750802));
#18938=CARTESIAN_POINT('Origin',(-92.,-24.,5.));
#18939=CARTESIAN_POINT('',(-94.5199606688991,-23.9982645762516,6.38741669750803));
#18940=CARTESIAN_POINT('',(-94.5147663248015,-23.9983410423439,6.11258330249198));
#18941=CARTESIAN_POINT('',(-94.5175,-24.,5.));
#18942=CARTESIAN_POINT('Ctrl Pts',(-94.5147663248015,-23.9983410423439,
6.11258330249198));
#18943=CARTESIAN_POINT('Ctrl Pts',(-94.5166143414574,-23.6963819206475,
6.09354263098009));
#18944=CARTESIAN_POINT('Ctrl Pts',(-94.4662620027174,-23.3950183934936,
6.0745019594682));
#18945=CARTESIAN_POINT('Ctrl Pts',(-94.3609399824778,-23.1142771205844,
6.0554612879563));
#18946=CARTESIAN_POINT('Ctrl Pts',(-94.0696493782671,-22.3378270028733,
6.00280023287342));
#18947=CARTESIAN_POINT('Ctrl Pts',(-93.3578860664944,-21.7191201145527,
5.95013917779055));
#18948=CARTESIAN_POINT('Ctrl Pts',(-92.5484468560347,-21.5387505883927,
5.89747812270767));
#18949=CARTESIAN_POINT('Ctrl Pts',(-91.739007645575,-21.3583810622326,5.84481706762479));
#18950=CARTESIAN_POINT('Ctrl Pts',(-90.8318925364285,-21.616348898233,5.79215601254191));
#18951=CARTESIAN_POINT('Ctrl Pts',(-90.2384937114928,-22.1956612802578,
5.73949495745903));
#18952=CARTESIAN_POINT('Ctrl Pts',(-89.6450948865571,-22.7749736622827,
5.68683390237615));
#18953=CARTESIAN_POINT('Ctrl Pts',(-89.3654123458324,-23.6756305903319,
5.63417284729328));
#18954=CARTESIAN_POINT('Ctrl Pts',(-89.5262868946163,-24.4891687768701,
5.5815117922104));
#18955=CARTESIAN_POINT('Ctrl Pts',(-89.6871614434003,-25.3027069634083,
5.52885073712752));
#18956=CARTESIAN_POINT('Ctrl Pts',(-90.2885930816928,-26.0291264084354,
5.47618968204464));
#18957=CARTESIAN_POINT('Ctrl Pts',(-91.0578222974529,-26.3389834964905,
5.42352862696176));
#18958=CARTESIAN_POINT('Ctrl Pts',(-91.8270515132129,-26.6488405845455,
5.37086757187889));
#18959=CARTESIAN_POINT('Ctrl Pts',(-92.7640783064405,-26.5421353156285,
5.31820651679601));
#18960=CARTESIAN_POINT('Ctrl Pts',(-93.4439450350434,-26.0672603502598,
5.26554546171313));
#18961=CARTESIAN_POINT('Ctrl Pts',(-94.1022043035296,-25.6074778161617,
5.21455807530608));
#18962=CARTESIAN_POINT('Ctrl Pts',(-94.5193898264468,-24.8025559702574,
5.16357068889903));
#18963=CARTESIAN_POINT('Ctrl Pts',(-94.5215003759084,-23.999522240299,5.11258330249198));
#18964=CARTESIAN_POINT('Ctrl Pts',(-94.5184743499735,-24.0021560918536,
5.38741669750802));
#18965=CARTESIAN_POINT('Ctrl Pts',(-94.5199520063111,-24.1657918820634,
5.39777386760188));
#18966=CARTESIAN_POINT('Ctrl Pts',(-94.5053532314692,-24.3291652655504,
5.40813103769574));
#18967=CARTESIAN_POINT('Ctrl Pts',(-94.4737130558303,-24.4891687670711,
5.4184882077896));
#18968=CARTESIAN_POINT('Ctrl Pts',(-94.3128385102691,-25.3027069373126,
5.47114926287248));
#18969=CARTESIAN_POINT('Ctrl Pts',(-93.7114068840245,-26.0291263677881,
5.52381031795536));
#18970=CARTESIAN_POINT('Ctrl Pts',(-92.9421776836735,-26.3389834496362,
5.57647137303824));
#18971=CARTESIAN_POINT('Ctrl Pts',(-92.1729484833227,-26.6488405314842,
5.62913242812112));
#18972=CARTESIAN_POINT('Ctrl Pts',(-91.2359217088655,-26.5421352647047,
5.68179348320399));
#18973=CARTESIAN_POINT('Ctrl Pts',(-90.5560549938817,-26.0672603088487,
5.73445453828687));
#18974=CARTESIAN_POINT('Ctrl Pts',(-89.8761882788978,-25.5923853529926,
5.78711559336975));
#18975=CARTESIAN_POINT('Ctrl Pts',(-89.4534816233873,-24.7493407080601,
5.83977664845263));
#18976=CARTESIAN_POINT('Ctrl Pts',(-89.479639709574,-23.9204615079354,5.8924377035355));
#18977=CARTESIAN_POINT('Ctrl Pts',(-89.5057977957607,-23.0915823078108,
5.94509875861838));
#18978=CARTESIAN_POINT('Ctrl Pts',(-89.9808206236446,-22.276868552494,5.99775981370126));
#18979=CARTESIAN_POINT('Ctrl Pts',(-90.6892772339901,-21.845806834092,6.05042086878414));
#18980=CARTESIAN_POINT('Ctrl Pts',(-91.3977338443356,-21.4147451156901,
6.10308192386702));
#18981=CARTESIAN_POINT('Ctrl Pts',(-92.3396242371427,-21.3673354342031,
6.15574297894989));
#18982=CARTESIAN_POINT('Ctrl Pts',(-93.0877850449385,-21.7250788890635,
6.20840403403277));
#18983=CARTESIAN_POINT('Ctrl Pts',(-93.8359458527343,-22.0828223439238,
6.26106508911565));
#18984=CARTESIAN_POINT('Ctrl Pts',(-94.3903770755186,-22.8457189351315,
6.31372614419853));
#18985=CARTESIAN_POINT('Ctrl Pts',(-94.499634691726,-23.6677820393728,6.36638719928141));
#18986=CARTESIAN_POINT('Ctrl Pts',(-94.5141782213651,-23.7772087277519,
6.37339703202361));
#18987=CARTESIAN_POINT('Ctrl Pts',(-94.5208337745228,-23.8876837803117,
6.38040686476582));
#18988=CARTESIAN_POINT('Ctrl Pts',(-94.5199606688991,-23.9982645762516,
6.38741669750803));
#18989=CARTESIAN_POINT('Origin',(-92.,-24.,5.));
#18990=CARTESIAN_POINT('',(-94.5136290410546,-23.9995053986546,7.38741669750802));
#18991=CARTESIAN_POINT('',(-94.5157926212741,-24.0020516723221,7.11258330249199));
#18992=CARTESIAN_POINT('',(-94.5175,-24.,5.));
#18993=CARTESIAN_POINT('Ctrl Pts',(-94.5157926212741,-24.0020516723221,
7.11258330249199));
#18994=CARTESIAN_POINT('Ctrl Pts',(-94.511298858366,-23.4252696399995,7.07617562814403));
#18995=CARTESIAN_POINT('Ctrl Pts',(-94.3140599311548,-22.8457098245431,
7.03976795379607));
#18996=CARTESIAN_POINT('Ctrl Pts',(-93.9507614766045,-22.4021663794855,
7.00336027944811));
#18997=CARTESIAN_POINT('Ctrl Pts',(-93.4252766641513,-21.7606130199219,
6.95069922436523));
#18998=CARTESIAN_POINT('Ctrl Pts',(-92.5523700775016,-21.4036265833224,
6.89803816928235));
#18999=CARTESIAN_POINT('Ctrl Pts',(-91.7279197494919,-21.4931065124105,
6.84537711419947));
#19000=CARTESIAN_POINT('Ctrl Pts',(-90.9034694214823,-21.5825864414987,
6.7927160591166));
#19001=CARTESIAN_POINT('Ctrl Pts',(-90.1274753521127,-22.1185327362746,
6.74005500403372));
#19002=CARTESIAN_POINT('Ctrl Pts',(-89.7518640956472,-22.8578846048887,
6.68739394895084));
#19003=CARTESIAN_POINT('Ctrl Pts',(-89.3762528391816,-23.5972364735029,
6.63473289386796));
#19004=CARTESIAN_POINT('Ctrl Pts',(-89.4010243956202,-24.5399939159553,
6.58207183878508));
#19005=CARTESIAN_POINT('Ctrl Pts',(-89.8149444410542,-25.258600343256,6.52941078370221));
#19006=CARTESIAN_POINT('Ctrl Pts',(-90.2288644864881,-25.9772067705567,
6.47674972861933));
#19007=CARTESIAN_POINT('Ctrl Pts',(-91.0319330209175,-26.4716621827057,
6.42408867353645));
#19008=CARTESIAN_POINT('Ctrl Pts',(-91.8599447589054,-26.5177226117209,
6.37142761845357));
#19009=CARTESIAN_POINT('Ctrl Pts',(-92.6879564968933,-26.5637830407361,
6.31876656337069));
#19010=CARTESIAN_POINT('Ctrl Pts',(-93.5409114384396,-26.1614484866175,
6.26610550828782));
#19011=CARTESIAN_POINT('Ctrl Pts',(-94.0319799608884,-25.4931845360073,
6.21344445320494));
#19012=CARTESIAN_POINT('Ctrl Pts',(-94.3454927087508,-25.0665449574646,
6.17982406963395));
#19013=CARTESIAN_POINT('Ctrl Pts',(-94.5115032555984,-24.531514543491,6.14620368606297));
#19014=CARTESIAN_POINT('Ctrl Pts',(-94.5147663248015,-23.9983410423439,
6.11258330249198));
#19015=CARTESIAN_POINT('Ctrl Pts',(-94.5199606688991,-23.9982645762516,
6.38741669750803));
#19016=CARTESIAN_POINT('Ctrl Pts',(-94.5142746075592,-24.7184170660063,
6.4330679198487));
#19017=CARTESIAN_POINT('Ctrl Pts',(-94.1892825133498,-25.44305435182,6.47871914218937));
#19018=CARTESIAN_POINT('Ctrl Pts',(-93.6442303551587,-25.9118182197226,
6.52437036453004));
#19019=CARTESIAN_POINT('Ctrl Pts',(-93.0154843927538,-26.4525616785562,
6.57703141961292));
#19020=CARTESIAN_POINT('Ctrl Pts',(-92.0939084583139,-26.6528189789487,
6.6296924746958));
#19021=CARTESIAN_POINT('Ctrl Pts',(-91.2974529654966,-26.4217700194305,
6.68235352977868));
#19022=CARTESIAN_POINT('Ctrl Pts',(-90.5009974726793,-26.1907210599122,
6.73501458486156));
#19023=CARTESIAN_POINT('Ctrl Pts',(-89.8296624214848,-25.5283658404831,
6.78767563994443));
#19024=CARTESIAN_POINT('Ctrl Pts',(-89.5879097152778,-24.7350937531495,
6.84033669502731));
#19025=CARTESIAN_POINT('Ctrl Pts',(-89.3461570090709,-23.941821665816,6.89299775011019));
#19026=CARTESIAN_POINT('Ctrl Pts',(-89.5339866478515,-23.0176327105779,
6.94565880519307));
#19027=CARTESIAN_POINT('Ctrl Pts',(-90.0662146837015,-22.3816623586851,
6.99831986027595));
#19028=CARTESIAN_POINT('Ctrl Pts',(-90.5984427195515,-21.7456920067922,
7.05098091535882));
#19029=CARTESIAN_POINT('Ctrl Pts',(-91.4750691524708,-21.3979402582445,
7.1036419704417));
#19030=CARTESIAN_POINT('Ctrl Pts',(-92.2985289370466,-21.4961184498875,
7.15630302552458));
#19031=CARTESIAN_POINT('Ctrl Pts',(-93.1219887216224,-21.5942966415305,
7.20896408060745));
#19032=CARTESIAN_POINT('Ctrl Pts',(-93.8922818578547,-22.1384047733641,
7.26162513569033));
#19033=CARTESIAN_POINT('Ctrl Pts',(-94.2600672575076,-22.8816805542397,
7.31428619077321));
#19034=CARTESIAN_POINT('Ctrl Pts',(-94.4303153507392,-23.2257433815264,
7.33866302635148));
#19035=CARTESIAN_POINT('Ctrl Pts',(-94.5143152963871,-23.6124832538171,
7.36303986192975));
#19036=CARTESIAN_POINT('Ctrl Pts',(-94.5136290410546,-23.9995053986546,
7.38741669750802));
#19037=CARTESIAN_POINT('Origin',(-92.,-24.,5.));
#19038=CARTESIAN_POINT('',(-94.5182106813093,-24.0021944371302,8.38741669750803));
#19039=CARTESIAN_POINT('',(-94.5215633824187,-23.9996804087645,8.11258330249198));
#19040=CARTESIAN_POINT('',(-94.5175,-24.,5.));
#19041=CARTESIAN_POINT('Ctrl Pts',(-94.5215633824187,-23.9996804087645,
8.11258330249198));
#19042=CARTESIAN_POINT('Ctrl Pts',(-94.5215950065109,-23.9821424208032,
8.11146968039084));
#19043=CARTESIAN_POINT('Ctrl Pts',(-94.5214276959298,-23.9646050519463,
8.11035605828969));
#19044=CARTESIAN_POINT('Ctrl Pts',(-94.5210595996876,-23.9470718985317,
8.10924243618855));
#19045=CARTESIAN_POINT('Ctrl Pts',(-94.5036530337929,-23.1179626730646,
8.05658138110567));
#19046=CARTESIAN_POINT('Ctrl Pts',(-94.0372570305162,-22.2982798630938,
8.0039203260228));
#19047=CARTESIAN_POINT('Ctrl Pts',(-93.3333903289359,-21.8597634086716,
7.95125927093992));
#19048=CARTESIAN_POINT('Ctrl Pts',(-92.6295236273557,-21.4212469542493,
7.89859821585704));
#19049=CARTESIAN_POINT('Ctrl Pts',(-91.688186227472,-21.3638968553754,7.84593716077416));
#19050=CARTESIAN_POINT('Ctrl Pts',(-90.9362906110337,-21.7137224600414,
7.79327610569128));
#19051=CARTESIAN_POINT('Ctrl Pts',(-90.1843949945955,-22.0635480647074,
7.7406150506084));
#19052=CARTESIAN_POINT('Ctrl Pts',(-89.6219411616028,-22.8205493729132,
7.68795399552553));
#19053=CARTESIAN_POINT('Ctrl Pts',(-89.5040115702347,-23.6414133236746,
7.63529294044265));
#19054=CARTESIAN_POINT('Ctrl Pts',(-89.3860819788666,-24.4622772744359,
7.58263188535977));
#19055=CARTESIAN_POINT('Ctrl Pts',(-89.7126766291231,-25.3470038677529,
7.52997083027689));
#19056=CARTESIAN_POINT('Ctrl Pts',(-90.3356792508831,-25.8943545185808,
7.47730977519401));
#19057=CARTESIAN_POINT('Ctrl Pts',(-90.9586818726431,-26.4417051694086,
7.42464872011113));
#19058=CARTESIAN_POINT('Ctrl Pts',(-91.8780924659066,-26.6516798777473,
7.37198766502825));
#19059=CARTESIAN_POINT('Ctrl Pts',(-92.6769426469386,-26.429051518253,7.31932660994538));
#19060=CARTESIAN_POINT('Ctrl Pts',(-93.4757928279705,-26.2064231587587,
7.2666655548625));
#19061=CARTESIAN_POINT('Ctrl Pts',(-94.1540825967709,-25.5511917314315,
7.21400449977962));
#19062=CARTESIAN_POINT('Ctrl Pts',(-94.4041959620427,-24.760515876504,7.16134344469674));
#19063=CARTESIAN_POINT('Ctrl Pts',(-94.4813912963606,-24.516480589178,7.14509006396182));
#19064=CARTESIAN_POINT('Ctrl Pts',(-94.5177987598365,-24.2595429331701,
7.1288366832269));
#19065=CARTESIAN_POINT('Ctrl Pts',(-94.5157926212741,-24.0020516723221,
7.11258330249199));
#19066=CARTESIAN_POINT('Ctrl Pts',(-94.5136290410546,-23.9995053986546,
7.38741669750802));
#19067=CARTESIAN_POINT('Ctrl Pts',(-94.5128327852651,-24.4485636557274,
7.41570091701263));
#19068=CARTESIAN_POINT('Ctrl Pts',(-94.3980256245316,-24.8980019292388,
7.44398513651724));
#19069=CARTESIAN_POINT('Ctrl Pts',(-94.1716474294659,-25.2815965984927,
7.47226935602185));
#19070=CARTESIAN_POINT('Ctrl Pts',(-93.7501645386979,-25.9957934319524,
7.52493041110473));
#19071=CARTESIAN_POINT('Ctrl Pts',(-92.9419210940886,-26.4817436689545,
7.5775914661876));
#19072=CARTESIAN_POINT('Ctrl Pts',(-92.1134692701342,-26.5190607190089,
7.63025252127048));
#19073=CARTESIAN_POINT('Ctrl Pts',(-91.2850174461799,-26.5563777690633,
7.68291357635336));
#19074=CARTESIAN_POINT('Ctrl Pts',(-90.4363572428804,-26.1450616321701,
7.73557463143624));
#19075=CARTESIAN_POINT('Ctrl Pts',(-89.9523705889737,-25.4716509197329,
7.78823568651912));
#19076=CARTESIAN_POINT('Ctrl Pts',(-89.468383935067,-24.7982402072957,7.840896741602));
#19077=CARTESIAN_POINT('Ctrl Pts',(-89.3490708305531,-23.8627349193145,
7.89355779668488));
#19078=CARTESIAN_POINT('Ctrl Pts',(-89.6485417162137,-23.0894032334354,
7.94621885176776));
#19079=CARTESIAN_POINT('Ctrl Pts',(-89.9480126018744,-22.3160715475563,
7.99887990685064));
#19080=CARTESIAN_POINT('Ctrl Pts',(-90.6662674777097,-21.7049134637795,
8.05154096193351));
#19081=CARTESIAN_POINT('Ctrl Pts',(-91.4775656801192,-21.5330984509984,
8.10420201701639));
#19082=CARTESIAN_POINT('Ctrl Pts',(-92.2888638825287,-21.3612834382173,
8.15686307209926));
#19083=CARTESIAN_POINT('Ctrl Pts',(-93.1932054115124,-21.628811496432,8.20952412718214));
#19084=CARTESIAN_POINT('Ctrl Pts',(-93.7804555817247,-22.2143564386821,
8.26218518226502));
#19085=CARTESIAN_POINT('Ctrl Pts',(-94.2459623243365,-22.6785114658678,
8.30392902067935));
#19086=CARTESIAN_POINT('Ctrl Pts',(-94.5122228629259,-23.3424942562717,
8.34567285909369));
#19087=CARTESIAN_POINT('Ctrl Pts',(-94.5182106813093,-24.0021944371302,
8.38741669750803));
#19088=CARTESIAN_POINT('Origin',(-92.,-24.,5.));
#19089=CARTESIAN_POINT('',(-94.5201759878003,-23.9984131478585,9.38741669750803));
#19090=CARTESIAN_POINT('',(-94.5149492652116,-23.9982505980887,9.11258330249199));
#19091=CARTESIAN_POINT('',(-94.5175,-24.,5.));
#19092=CARTESIAN_POINT('',(-90.0865340033349,-22.3640127966251,10.));
#19093=CARTESIAN_POINT('Ctrl Pts',(-94.5201759878003,-23.9984131478585,
9.38741669750803));
#19094=CARTESIAN_POINT('Ctrl Pts',(-94.5146936217042,-24.7270926513296,
9.43362796642338));
#19095=CARTESIAN_POINT('Ctrl Pts',(-94.1807325653029,-25.4600317456745,
9.47983923533874));
#19096=CARTESIAN_POINT('Ctrl Pts',(-93.6239879633604,-25.9288767806186,
9.5260505042541));
#19097=CARTESIAN_POINT('Ctrl Pts',(-92.9895375611503,-26.4631593223022,
9.57871155933697));
#19098=CARTESIAN_POINT('Ctrl Pts',(-92.0657751669118,-26.6544830596339,
9.63137261441985));
#19099=CARTESIAN_POINT('Ctrl Pts',(-91.2718706971314,-26.4146105241973,
9.68403366950273));
#19100=CARTESIAN_POINT('Ctrl Pts',(-90.4779662273509,-26.1747379887606,
9.73669472458561));
#19101=CARTESIAN_POINT('Ctrl Pts',(-89.8139196820286,-25.5036691805558,
9.78935577966849));
#19102=CARTESIAN_POINT('Ctrl Pts',(-89.5807331050278,-24.7092693915533,
9.84201683475137));
#19103=CARTESIAN_POINT('Ctrl Pts',(-89.347546528027,-23.9148696025509,9.89467788983425));
#19104=CARTESIAN_POINT('Ctrl Pts',(-89.5452199193478,-22.9971388327508,
9.94733894491712));
#19105=CARTESIAN_POINT('Ctrl Pts',(-90.0865340033349,-22.3640127966251,
10.));
#19106=CARTESIAN_POINT('',(-93.9171033105362,-22.361465667796,10.));
#19107=CARTESIAN_POINT('Origin',(-92.,-24.,10.));
#19108=CARTESIAN_POINT('Ctrl Pts',(-93.9171117712833,-22.3614597429257,
10.));
#19109=CARTESIAN_POINT('Ctrl Pts',(-93.3939570615584,-21.7523041616072,
9.94901908464118));
#19110=CARTESIAN_POINT('Ctrl Pts',(-92.5534187329286,-21.4121722649682,
9.89803816928236));
#19111=CARTESIAN_POINT('Ctrl Pts',(-91.7542642249036,-21.4905146133598,
9.84705725392353));
#19112=CARTESIAN_POINT('Ctrl Pts',(-90.9287725821855,-21.5714388316664,
9.79439619884065));
#19113=CARTESIAN_POINT('Ctrl Pts',(-90.1474374185984,-22.0988744884398,
9.74173514375777));
#19114=CARTESIAN_POINT('Ctrl Pts',(-89.7641119401365,-22.8341462635555,
9.68907408867489));
#19115=CARTESIAN_POINT('Ctrl Pts',(-89.3807864616747,-23.5694180386713,
9.63641303359201));
#19116=CARTESIAN_POINT('Ctrl Pts',(-89.3954706683381,-24.5125259321295,
9.58375197850913));
#19117=CARTESIAN_POINT('Ctrl Pts',(-89.8017475811355,-25.2354979451803,
9.53109092342626));
#19118=CARTESIAN_POINT('Ctrl Pts',(-90.2080244939329,-25.9584699582311,
9.47842986834338));
#19119=CARTESIAN_POINT('Ctrl Pts',(-91.0058941128642,-26.4613060908746,
9.4257688132605));
#19120=CARTESIAN_POINT('Ctrl Pts',(-91.8333901989263,-26.5160871276519,
9.37310775817762));
#19121=CARTESIAN_POINT('Ctrl Pts',(-92.6608862849884,-26.5708681644292,
9.32044670309475));
#19122=CARTESIAN_POINT('Ctrl Pts',(-93.5180088381812,-26.1775941053403,
9.26778564801187));
#19123=CARTESIAN_POINT('Ctrl Pts',(-94.0160962955284,-25.5145599775471,
9.21512459292899));
#19124=CARTESIAN_POINT('Ctrl Pts',(-94.339387264832,-25.0842079526291,9.18094416278332));
#19125=CARTESIAN_POINT('Ctrl Pts',(-94.5114221549398,-24.5402100730638,
9.14676373263765));
#19126=CARTESIAN_POINT('Ctrl Pts',(-94.5149492652116,-23.9982505980887,
9.11258330249199));
#19127=CARTESIAN_POINT('Origin',(-92.,-24.,12.2084234471775));
#19128=CARTESIAN_POINT('',(-95.0782768196867,-23.9992118911386,1.79157655282254));
#19129=CARTESIAN_POINT('',(-95.0686110023456,-23.9996651237392,1.70842344717745));
#19130=CARTESIAN_POINT('',(-95.0735,-23.9999999999999,12.2084234471775));
#19131=CARTESIAN_POINT('',(-91.2062007174672,-26.9692229537457,0.999999999999999));
#19132=CARTESIAN_POINT('Ctrl Pts',(-95.0686110023456,-23.9996651237392,
1.70842344717745));
#19133=CARTESIAN_POINT('Ctrl Pts',(-95.0689534453578,-23.5053846687107,
1.68292651844982));
#19134=CARTESIAN_POINT('Ctrl Pts',(-94.7235567931003,-21.9907712706008,
1.6047685346393));
#19135=CARTESIAN_POINT('Ctrl Pts',(-92.3539161166825,-20.3911596148569,
1.4739494957459));
#19136=CARTESIAN_POINT('Ctrl Pts',(-89.1687759971456,-21.7301450507159,
1.31596633049727));
#19137=CARTESIAN_POINT('Ctrl Pts',(-88.5566856051374,-25.1332975040883,
1.15798316524863));
#19138=CARTESIAN_POINT('Ctrl Pts',(-90.2237466982397,-26.7065713079336,
1.05266105508288));
#19139=CARTESIAN_POINT('Ctrl Pts',(-91.2062007174672,-26.9692229537457,
0.999999999999999));
#19140=CARTESIAN_POINT('',(-92.7937992825329,-26.9692229537457,1.));
#19141=CARTESIAN_POINT('Origin',(-92.,-24.,0.999999999999999));
#19142=CARTESIAN_POINT('Ctrl Pts',(-95.0782768196867,-23.9992118911386,
1.79157655282254));
#19143=CARTESIAN_POINT('Ctrl Pts',(-95.0784229132411,-23.9562584982139,
1.78934283757203));
#19144=CARTESIAN_POINT('Ctrl Pts',(-95.058222313234,-22.9007975699364,1.73444806723864));
#19145=CARTESIAN_POINT('Ctrl Pts',(-93.8523950876059,-20.8820465732966,
1.62689224182237));
#19146=CARTESIAN_POINT('Ctrl Pts',(-90.400968139612,-20.7444872144857,1.46890907657374));
#19147=CARTESIAN_POINT('Ctrl Pts',(-88.4000491745082,-23.5606286501727,
1.31092591132511));
#19148=CARTESIAN_POINT('Ctrl Pts',(-89.6506964041097,-26.7394102869818,
1.15462288580053));
#19149=CARTESIAN_POINT('Ctrl Pts',(-91.8480946426715,-27.2254055619768,
1.05098091535883));
#19150=CARTESIAN_POINT('Ctrl Pts',(-92.7957017813267,-26.9743128096467,
1.));
#19151=CARTESIAN_POINT('Origin',(-92.,-24.,12.2084234471775));
#19152=CARTESIAN_POINT('',(-95.0699491247542,-23.9980972118633,2.79157655282254));
#19153=CARTESIAN_POINT('',(-95.075008445109,-24.0025755322285,2.70842344717745));
#19154=CARTESIAN_POINT('',(-95.0735,-23.9999999999999,12.2084234471775));
#19155=CARTESIAN_POINT('Ctrl Pts',(-95.075008445109,-24.0025755322285,2.70842344717745));
#19156=CARTESIAN_POINT('Ctrl Pts',(-95.0676143896354,-23.1760102841626,
2.66555951561375));
#19157=CARTESIAN_POINT('Ctrl Pts',(-94.2993641383816,-21.3218328468575,
2.57003452896717));
#19158=CARTESIAN_POINT('Ctrl Pts',(-91.1738621865499,-20.4685620798055,
2.42184848723771));
#19159=CARTESIAN_POINT('Ctrl Pts',(-88.5910234496018,-22.7619776832305,
2.26386532198907));
#19160=CARTESIAN_POINT('Ctrl Pts',(-89.1003113510008,-26.1783942746989,
2.10588215674044));
#19161=CARTESIAN_POINT('Ctrl Pts',(-92.2395758256157,-27.6187848570707,
1.94789899149181));
#19162=CARTESIAN_POINT('Ctrl Pts',(-94.690200871183,-26.074343589762,1.81541275497081));
#19163=CARTESIAN_POINT('Ctrl Pts',(-95.0682461676098,-24.5262656754664,
1.73558757353269));
#19164=CARTESIAN_POINT('Ctrl Pts',(-95.0686110023456,-23.9996651237392,
1.70842344717745));
#19165=CARTESIAN_POINT('Ctrl Pts',(-95.0699491247542,-23.9980972118633,
2.79157655282254));
#19166=CARTESIAN_POINT('Ctrl Pts',(-95.0721211881234,-23.6185397169383,
2.77197583473597));
#19167=CARTESIAN_POINT('Ctrl Pts',(-94.8315580332634,-22.2218843885843,
2.69971406156651));
#19168=CARTESIAN_POINT('Ctrl Pts',(-92.7514083751607,-20.4518994955132,
2.57479123331418));
#19169=CARTESIAN_POINT('Ctrl Pts',(-89.4392013302128,-21.4317376344076,
2.41680806806554));
#19170=CARTESIAN_POINT('Ctrl Pts',(-88.4497278964895,-24.7410889661721,
2.25882490281691));
#19171=CARTESIAN_POINT('Ctrl Pts',(-90.6804687378896,-27.3782236865054,
2.10084173756828));
#19172=CARTESIAN_POINT('Ctrl Pts',(-94.0596142672113,-26.9572795305498,
1.94509228757015));
#19173=CARTESIAN_POINT('Ctrl Pts',(-95.0749786780308,-24.9689081590363,
1.84200389265491));
#19174=CARTESIAN_POINT('Ctrl Pts',(-95.0782768196867,-23.9992118911386,
1.79157655282254));
#19175=CARTESIAN_POINT('Origin',(-92.,-24.,12.2084234471775));
#19176=CARTESIAN_POINT('',(-95.0716998581065,-24.0025715694568,3.79157655282254));
#19177=CARTESIAN_POINT('',(-95.0762206925999,-23.9977671184427,3.70842344717745));
#19178=CARTESIAN_POINT('',(-95.0735,-23.9999999999999,12.2084234471775));
#19179=CARTESIAN_POINT('Ctrl Pts',(-95.0762206925998,-23.9977671184427,
3.70842344717745));
#19180=CARTESIAN_POINT('Ctrl Pts',(-95.0774154713987,-23.8519430387288,
3.70085356786056));
#19181=CARTESIAN_POINT('Ctrl Pts',(-95.0019701064919,-22.6929124367374,
3.6406226334608));
#19182=CARTESIAN_POINT('Ctrl Pts',(-93.5299146181504,-20.7116868408496,
3.52773064397815));
#19183=CARTESIAN_POINT('Ctrl Pts',(-90.0822080355936,-20.9217351333484,
3.36974747872952));
#19184=CARTESIAN_POINT('Ctrl Pts',(-88.3740037605625,-23.92387423856,3.21176431348088));
#19185=CARTESIAN_POINT('Ctrl Pts',(-89.9547027823836,-26.99506300667,3.05378114823225));
#19186=CARTESIAN_POINT('Ctrl Pts',(-93.3905542616683,-27.349625359661,2.89579798298362));
#19187=CARTESIAN_POINT('Ctrl Pts',(-94.9751245860296,-25.3940964065108,
2.78067874929868));
#19188=CARTESIAN_POINT('Ctrl Pts',(-95.076698455151,-24.1914980490519,2.71822057069663));
#19189=CARTESIAN_POINT('Ctrl Pts',(-95.075008445109,-24.0025755322285,2.70842344717745));
#19190=CARTESIAN_POINT('Ctrl Pts',(-95.0716998581065,-24.0025715694568,
3.79157655282254));
#19191=CARTESIAN_POINT('Ctrl Pts',(-95.0659415382079,-23.2877405601207,
3.7546088318999));
#19192=CARTESIAN_POINT('Ctrl Pts',(-94.4623934875611,-21.5458532246353,
3.66498005589439));
#19193=CARTESIAN_POINT('Ctrl Pts',(-91.5706310215098,-20.3987107062197,
3.52269022480599));
#19194=CARTESIAN_POINT('Ctrl Pts',(-88.7493845448822,-22.3915405493825,
3.36470705955735));
#19195=CARTESIAN_POINT('Ctrl Pts',(-88.8765572614881,-25.8432981737925,
3.20672389430872));
#19196=CARTESIAN_POINT('Ctrl Pts',(-91.8367991007263,-27.6231211133645,
3.04874072906008));
#19197=CARTESIAN_POINT('Ctrl Pts',(-94.5594316628929,-26.3035556341772,
2.91035828189803));
#19198=CARTESIAN_POINT('Ctrl Pts',(-95.0662855269897,-24.6382930779672,
2.82463688981884));
#19199=CARTESIAN_POINT('Ctrl Pts',(-95.0699491247542,-23.9980972118633,
2.79157655282254));
#19200=CARTESIAN_POINT('Origin',(-92.,-24.,12.2084234471775));
#19201=CARTESIAN_POINT('',(-95.0783838750166,-23.9994167251475,4.79157655282254));
#19202=CARTESIAN_POINT('',(-95.0687191146691,-23.9995675532748,4.70842344717746));
#19203=CARTESIAN_POINT('',(-95.0735,-23.9999999999999,12.2084234471775));
#19204=CARTESIAN_POINT('Ctrl Pts',(-95.0687191146691,-23.9995675532748,
4.70842344717746));
#19205=CARTESIAN_POINT('Ctrl Pts',(-95.0693322679534,-23.5161929491143,
4.6834865650245));
#19206=CARTESIAN_POINT('Ctrl Pts',(-94.7346951702921,-22.0128432522753,
4.60588862778867));
#19207=CARTESIAN_POINT('Ctrl Pts',(-92.3913282785029,-20.3943788173916,
4.47562963546995));
#19208=CARTESIAN_POINT('Ctrl Pts',(-89.1942537915232,-21.7018637718047,
4.31764647022133));
#19209=CARTESIAN_POINT('Ctrl Pts',(-88.5420868753907,-25.0938367187666,
4.15966330497269));
#19210=CARTESIAN_POINT('Ctrl Pts',(-91.0263652022841,-27.4936624405808,
4.00168013972406));
#19211=CARTESIAN_POINT('Ctrl Pts',(-94.2324121355514,-26.7614664286127,
3.85126685379231));
#19212=CARTESIAN_POINT('Ctrl Pts',(-95.0691038049237,-24.8663911656747,
3.75351462294344));
#19213=CARTESIAN_POINT('Ctrl Pts',(-95.0762206925998,-23.9977671184427,
3.70842344717745));
#19214=CARTESIAN_POINT('Ctrl Pts',(-95.0783838750166,-23.9994167251475,
4.79157655282255));
#19215=CARTESIAN_POINT('Ctrl Pts',(-95.0784684546912,-23.9672353748386,
4.78990288414672));
#19216=CARTESIAN_POINT('Ctrl Pts',(-95.0634882463523,-22.9225663485135,
4.73556816038801));
#19217=CARTESIAN_POINT('Ctrl Pts',(-93.885189770327,-20.9016614152429,4.62857238154643));
#19218=CARTESIAN_POINT('Ctrl Pts',(-90.435457678629,-20.7280205108105,4.47058921629779));
#19219=CARTESIAN_POINT('Ctrl Pts',(-88.4048188734298,-23.5221766816715,
4.31260605104916));
#19220=CARTESIAN_POINT('Ctrl Pts',(-89.6351320616122,-26.7497349135866,
4.15462288580052));
#19221=CARTESIAN_POINT('Ctrl Pts',(-93.0104611872221,-27.4831897200468,
3.99663972055189));
#19222=CARTESIAN_POINT('Ctrl Pts',(-94.8939121321551,-25.6249319667866,
3.8756242762259));
#19223=CARTESIAN_POINT('Ctrl Pts',(-95.0741443484921,-24.3060277095063,
3.80726988698278));
#19224=CARTESIAN_POINT('Ctrl Pts',(-95.0716998581065,-24.0025715694568,
3.79157655282254));
#19225=CARTESIAN_POINT('Origin',(-92.,-24.,12.2084234471775));
#19226=CARTESIAN_POINT('',(-95.0701625816395,-23.9979746548734,5.79157655282255));
#19227=CARTESIAN_POINT('',(-95.0746895390838,-24.0026322734109,5.70842344717746));
#19228=CARTESIAN_POINT('',(-95.0735,-23.9999999999999,12.2084234471775));
#19229=CARTESIAN_POINT('Ctrl Pts',(-95.0746895390839,-24.0026322734109,
5.70842344717746));
#19230=CARTESIAN_POINT('Ctrl Pts',(-95.0673210859913,-23.1866491427393,
5.66611956218844));
#19231=CARTESIAN_POINT('Ctrl Pts',(-94.3157338396919,-21.3429097126816,
5.57115462211654));
#19232=CARTESIAN_POINT('Ctrl Pts',(-91.2111784520928,-20.4600278964634,
5.42352862696177));
#19233=CARTESIAN_POINT('Ctrl Pts',(-88.6043011989707,-22.7260802299219,
5.26554546171313));
#19234=CARTESIAN_POINT('Ctrl Pts',(-89.0774386607742,-26.1476212763575,
5.1075622964645));
#19235=CARTESIAN_POINT('Ctrl Pts',(-92.201439010718,-27.6211965224103,4.94957913121586));
#19236=CARTESIAN_POINT('Ctrl Pts',(-94.6784591036876,-26.0960763882475,
4.81653284812018));
#19237=CARTESIAN_POINT('Ctrl Pts',(-95.068037426895,-24.536970787307,4.73614762010738));
#19238=CARTESIAN_POINT('Ctrl Pts',(-95.0687191146691,-23.9995675532748,
4.70842344717746));
#19239=CARTESIAN_POINT('Ctrl Pts',(-95.0701625816395,-23.9979746548734,
5.79157655282255));
#19240=CARTESIAN_POINT('Ctrl Pts',(-95.0724187402062,-23.629326646717,5.77253588131065));
#19241=CARTESIAN_POINT('Ctrl Pts',(-94.8409295378372,-22.2438417959684,
5.70083415471588));
#19242=CARTESIAN_POINT('Ctrl Pts',(-92.7888215637087,-20.460027825551,5.57647137303824));
#19243=CARTESIAN_POINT('Ctrl Pts',(-89.4664561758693,-21.4048510358159,
5.4184882077896));
#19244=CARTESIAN_POINT('Ctrl Pts',(-88.4421015118167,-24.7035629345559,
5.26050504254097));
#19245=CARTESIAN_POINT('Ctrl Pts',(-90.6448822152433,-27.3641192375838,
5.10252187729233));
#19246=CARTESIAN_POINT('Ctrl Pts',(-94.0404433629951,-26.9774448457588,
4.94621238071953));
#19247=CARTESIAN_POINT('Ctrl Pts',(-95.0758072022182,-24.9798036840461,
4.8425639392296));
#19248=CARTESIAN_POINT('Ctrl Pts',(-95.0783838750166,-23.9994167251475,
4.79157655282255));
#19249=CARTESIAN_POINT('Origin',(-92.,-24.,12.2084234471775));
#19250=CARTESIAN_POINT('',(-95.0714155398157,-24.0025047924058,6.79157655282255));
#19251=CARTESIAN_POINT('',(-95.0765041175219,-23.9978813009372,6.70842344717745));
#19252=CARTESIAN_POINT('',(-95.0735,-23.9999999999999,12.2084234471775));
#19253=CARTESIAN_POINT('Ctrl Pts',(-95.0765041175219,-23.9978813009372,
6.70842344717746));
#19254=CARTESIAN_POINT('Ctrl Pts',(-95.077570052034,-23.8628782914748,6.70141361443525));
#19255=CARTESIAN_POINT('Ctrl Pts',(-95.008402446927,-22.7147701434973,6.64174272661016));
#19256=CARTESIAN_POINT('Ctrl Pts',(-93.5645422900301,-20.7280205763547,
6.52941078370221));
#19257=CARTESIAN_POINT('Ctrl Pts',(-90.1148102674372,-20.9016614773084,
6.37142761845357));
#19258=CARTESIAN_POINT('Ctrl Pts',(-88.3750096777633,-23.8856011718064,
6.21344445320494));
#19259=CARTESIAN_POINT('Ctrl Pts',(-89.9231990390881,-26.973304507894,6.0554612879563));
#19260=CARTESIAN_POINT('Ctrl Pts',(-93.3551177576112,-27.364119170194,5.89747812270767));
#19261=CARTESIAN_POINT('Ctrl Pts',(-94.9680496218174,-25.4159924088721,
5.78179884244805));
#19262=CARTESIAN_POINT('Ctrl Pts',(-95.0764935417666,-24.2024076860067,
5.71878061727132));
#19263=CARTESIAN_POINT('Ctrl Pts',(-95.0746895390839,-24.0026322734109,
5.70842344717746));
#19264=CARTESIAN_POINT('Ctrl Pts',(-95.0714155398157,-24.0025047924058,
6.79157655282255));
#19265=CARTESIAN_POINT('Ctrl Pts',(-95.0659293112961,-23.2983381285158,
6.75516887847459));
#19266=CARTESIAN_POINT('Ctrl Pts',(-94.4768297637754,-21.5673490693386,
6.66610014904376));
#19267=CARTESIAN_POINT('Ctrl Pts',(-91.6086717136577,-20.3943787451648,
6.52437036453004));
#19268=CARTESIAN_POINT('Ctrl Pts',(-88.7665452720996,-22.3573153135784,
6.36638719928141));
#19269=CARTESIAN_POINT('Ctrl Pts',(-88.8572726350159,-25.8102229593112,
6.20840403403277));
#19270=CARTESIAN_POINT('Ctrl Pts',(-91.7985609852469,-27.6211965949497,
6.05042086878414));
#19271=CARTESIAN_POINT('Ctrl Pts',(-94.5460461813276,-26.3252216524648,
5.9114783750474));
#19272=CARTESIAN_POINT('Ctrl Pts',(-95.0661788504793,-24.6489016680912,
5.82519693639353));
#19273=CARTESIAN_POINT('Ctrl Pts',(-95.0701625816395,-23.9979746548734,
5.79157655282255));
#19274=CARTESIAN_POINT('Origin',(-92.,-24.,12.2084234471775));
#19275=CARTESIAN_POINT('',(-95.0784607967682,-23.9996098257547,7.79157655282255));
#19276=CARTESIAN_POINT('',(-95.0687741242031,-23.9993961639582,7.70842344717745));
#19277=CARTESIAN_POINT('',(-95.0735,-23.9999999999999,12.2084234471775));
#19278=CARTESIAN_POINT('Ctrl Pts',(-95.0687741242031,-23.9993961639582,
7.70842344717745));
#19279=CARTESIAN_POINT('Ctrl Pts',(-95.0696119417857,-23.5268986218895,
7.68404661159918));
#19280=CARTESIAN_POINT('Ctrl Pts',(-94.7455188317854,-22.034758037689,7.60700872093803));
#19281=CARTESIAN_POINT('Ctrl Pts',(-92.4293689698895,-20.3987107783727,
7.47730977519402));
#19282=CARTESIAN_POINT('Ctrl Pts',(-89.2186702510282,-21.6723731408291,
7.31932660994537));
#19283=CARTESIAN_POINT('Ctrl Pts',(-88.5307325412461,-25.0572725496761,
7.16134344469675));
#19284=CARTESIAN_POINT('Ctrl Pts',(-90.9895388330194,-27.4831896502702,
7.0033602794481));
#19285=CARTESIAN_POINT('Ctrl Pts',(-94.2151019833044,-26.782278803337,6.85238694694169));
#19286=CARTESIAN_POINT('Ctrl Pts',(-95.0695622666666,-24.8770823643973,
6.75407466951813));
#19287=CARTESIAN_POINT('Ctrl Pts',(-95.0765041175219,-23.9978813009372,
6.70842344717746));
#19288=CARTESIAN_POINT('Ctrl Pts',(-95.0784607967682,-23.9996098257547,
7.79157655282255));
#19289=CARTESIAN_POINT('Ctrl Pts',(-95.0784994051683,-23.978198502617,7.7904629307214));
#19290=CARTESIAN_POINT('Ctrl Pts',(-95.0686359944837,-22.944323237583,7.73668825353738));
#19291=CARTESIAN_POINT('Ctrl Pts',(-93.9177920028682,-20.9217350716083,
7.63025252127049));
#19292=CARTESIAN_POINT('Ctrl Pts',(-90.4700853511787,-20.7116867750179,
7.47226935602185));
#19293=CARTESIAN_POINT('Ctrl Pts',(-88.4100632788413,-23.4842510500175,
7.31428619077322));
#19294=CARTESIAN_POINT('Ctrl Pts',(-89.6062364556796,-26.7246171090759,
7.15630302552458));
#19295=CARTESIAN_POINT('Ctrl Pts',(-92.9736348172232,-27.4936625105602,
6.99831986027594));
#19296=CARTESIAN_POINT('Ctrl Pts',(-94.8854041041608,-25.6468834845165,
6.87674436937527));
#19297=CARTESIAN_POINT('Ctrl Pts',(-95.073864742148,-24.3168640338026,6.80782993355747));
#19298=CARTESIAN_POINT('Ctrl Pts',(-95.0714155398157,-24.0025047924058,
6.79157655282255));
#19299=CARTESIAN_POINT('Origin',(-92.,-24.,12.2084234471775));
#19300=CARTESIAN_POINT('',(-95.0703859251749,-23.9978642356407,8.79157655282255));
#19301=CARTESIAN_POINT('',(-95.0743676381347,-24.0026790873961,8.70842344717746));
#19302=CARTESIAN_POINT('',(-95.0735,-23.9999999999999,12.2084234471775));
#19303=CARTESIAN_POINT('Ctrl Pts',(-95.0743676381347,-24.0026790873961,
8.70842344717746));
#19304=CARTESIAN_POINT('Ctrl Pts',(-95.0670573859793,-23.1972814683818,
8.66667960876313));
#19305=CARTESIAN_POINT('Ctrl Pts',(-94.3319129571347,-21.3640272738251,
8.57227471526591));
#19306=CARTESIAN_POINT('Ctrl Pts',(-91.2485916399685,-20.4518995672047,
8.42520876668582));
#19307=CARTESIAN_POINT('Ctrl Pts',(-88.6179385783441,-22.6903039808949,
8.26722560143718));
#19308=CARTESIAN_POINT('Ctrl Pts',(-89.0549302288588,-26.1166501607681,
8.10924243618856));
#19309=CARTESIAN_POINT('Ctrl Pts',(-92.1632008959979,-27.623121040698,7.95125927093991));
#19310=CARTESIAN_POINT('Ctrl Pts',(-94.6666767475757,-26.1179251847747,
7.81765294126956));
#19311=CARTESIAN_POINT('Ctrl Pts',(-95.0678020121201,-24.5476307431492,
7.73670766668206));
#19312=CARTESIAN_POINT('Ctrl Pts',(-95.0687741242031,-23.9993961639582,
7.70842344717745));
#19313=CARTESIAN_POINT('Ctrl Pts',(-95.0703859251749,-23.9978642356407,
8.79157655282255));
#19314=CARTESIAN_POINT('Ctrl Pts',(-95.0727141338614,-23.6401224413272,
8.77309592788534));
#19315=CARTESIAN_POINT('Ctrl Pts',(-94.8501668180301,-22.265785975548,8.70195424786526));
#19316=CARTESIAN_POINT('Ctrl Pts',(-92.8261378316182,-20.4685620052276,
8.57815151276229));
#19317=CARTESIAN_POINT('Ctrl Pts',(-89.493997396212,-21.3782456609066,8.42016834751365));
#19318=CARTESIAN_POINT('Ctrl Pts',(-88.4348704258472,-24.6659673604642,
8.26218518226502));
#19319=CARTESIAN_POINT('Ctrl Pts',(-90.6094457101907,-27.3496254273118,
8.10420201701639));
#19320=CARTESIAN_POINT('Ctrl Pts',(-94.0210779679427,-26.9975623737005,
7.94733247386889));
#19321=CARTESIAN_POINT('Ctrl Pts',(-95.0766736879126,-24.9906989423899,
7.84312398580428));
#19322=CARTESIAN_POINT('Ctrl Pts',(-95.0784607967682,-23.9996098257547,
7.79157655282255));
#19323=CARTESIAN_POINT('Origin',(-92.,-24.,12.2084234471775));
#19324=CARTESIAN_POINT('',(-95.0702887490762,-24.0031018432153,9.79157655282255));
#19325=CARTESIAN_POINT('',(-95.0767669904684,-23.998062685181,9.70842344717746));
#19326=CARTESIAN_POINT('',(-95.0735,-23.9999999999999,12.2084234471775));
#19327=CARTESIAN_POINT('',(-92.7937992825329,-26.9692229537457,10.));
#19328=CARTESIAN_POINT('Ctrl Pts',(-92.7937992825329,-26.9692229537457,
10.));
#19329=CARTESIAN_POINT('Ctrl Pts',(-93.7762533017603,-26.7065713079336,
9.94733894491712));
#19330=CARTESIAN_POINT('Ctrl Pts',(-94.875910333047,-25.6687793941585,9.87786446252464));
#19331=CARTESIAN_POINT('Ctrl Pts',(-95.0726354893275,-24.3283627763233,
9.80838998013215));
#19332=CARTESIAN_POINT('Ctrl Pts',(-95.0702887490763,-24.0031018432153,
9.79157655282255));
#19333=CARTESIAN_POINT('',(-91.2043026670138,-26.9743009685655,10.));
#19334=CARTESIAN_POINT('Origin',(-92.,-24.,10.));
#19335=CARTESIAN_POINT('Ctrl Pts',(-91.2042982523172,-26.9743127795766,
10.));
#19336=CARTESIAN_POINT('Ctrl Pts',(-92.1519054403102,-27.2254055803294,
9.94901908464118));
#19337=CARTESIAN_POINT('Ctrl Pts',(-94.2125562800898,-26.7696542914347,
9.851826900367));
#19338=CARTESIAN_POINT('Ctrl Pts',(-95.0700738217707,-24.8876739876312,
9.75463471609281));
#19339=CARTESIAN_POINT('Ctrl Pts',(-95.0767669904684,-23.998062685181,9.70842344717746));
#19340=CARTESIAN_POINT('Origin',(92.,24.,5.));
#19341=CARTESIAN_POINT('',(89.4865042982783,24.0002742229179,1.38741669750802));
#19342=CARTESIAN_POINT('',(89.4843731420168,23.9964690566784,1.11258330249198));
#19343=CARTESIAN_POINT('',(89.4825,24.,5.));
#19344=CARTESIAN_POINT('',(90.086534003335,25.635987203375,0.999999999999999));
#19345=CARTESIAN_POINT('Ctrl Pts',(89.4843731420168,23.9964690566784,1.11258330249198));
#19346=CARTESIAN_POINT('Ctrl Pts',(89.4895360512898,24.5890870308543,1.07505553499465));
#19347=CARTESIAN_POINT('Ctrl Pts',(89.7007781719159,25.1848035603044,1.03752776749733));
#19348=CARTESIAN_POINT('Ctrl Pts',(90.0865340033349,25.635987203375,0.999999999999998));
#19349=CARTESIAN_POINT('',(89.4825,24.,1.));
#19350=CARTESIAN_POINT('Origin',(92.,24.,1.));
#19351=CARTESIAN_POINT('',(89.4825,24.,0.));
#19352=CARTESIAN_POINT('',(89.4825,24.,5.));
#19353=CARTESIAN_POINT('Origin',(92.,24.,0.));
#19354=CARTESIAN_POINT('',(93.9171034684659,25.6385343514563,0.999999999999999));
#19355=CARTESIAN_POINT('Origin',(92.,24.,1.));
#19356=CARTESIAN_POINT('Ctrl Pts',(93.9171119325403,25.6385402784441,0.999999999999999));
#19357=CARTESIAN_POINT('Ctrl Pts',(93.3939572704879,26.2476956151711,1.05098091535882));
#19358=CARTESIAN_POINT('Ctrl Pts',(92.5534188240449,26.5878280192362,1.10196183071765));
#19359=CARTESIAN_POINT('Ctrl Pts',(91.7542642184068,26.50948576913,1.15294274607647));
#19360=CARTESIAN_POINT('Ctrl Pts',(90.9287724748586,26.4285616523478,1.20560380115935));
#19361=CARTESIAN_POINT('Ctrl Pts',(90.1474372319947,25.9011256605461,1.25826485624223));
#19362=CARTESIAN_POINT('Ctrl Pts',(89.7641117257107,25.1658537555941,1.31092591132511));
#19363=CARTESIAN_POINT('Ctrl Pts',(89.5785168283464,24.8098567987064,1.33642284005274));
#19364=CARTESIAN_POINT('Ctrl Pts',(89.4862237958222,24.4051387264905,1.36191976878038));
#19365=CARTESIAN_POINT('Ctrl Pts',(89.4865042982783,24.0002742229179,1.38741669750802));
#19366=CARTESIAN_POINT('Origin',(92.,24.,5.));
#19367=CARTESIAN_POINT('',(89.4812641621455,23.9978903848741,2.38741669750802));
#19368=CARTESIAN_POINT('',(89.4785876236681,24.0006455599548,2.11258330249198));
#19369=CARTESIAN_POINT('',(89.4825,24.,5.));
#19370=CARTESIAN_POINT('Ctrl Pts',(89.4785876236681,24.0006455599548,2.11258330249198));
#19371=CARTESIAN_POINT('Ctrl Pts',(89.4784679588298,24.0358286254365,2.11034958724147));
#19372=CARTESIAN_POINT('Ctrl Pts',(89.4791412415306,24.071006953815,2.10811587199096));
#19373=CARTESIAN_POINT('Ctrl Pts',(89.480621792432,24.1061512101346,2.10588215674044));
#19374=CARTESIAN_POINT('Ctrl Pts',(89.5155265872823,24.9346962171462,2.05322110165756));
#19375=CARTESIAN_POINT('Ctrl Pts',(89.9991161631697,25.7443037579803,2.00056004657469));
#19376=CARTESIAN_POINT('Ctrl Pts',(90.7120874500747,26.1678867011383,1.94789899149181));
#19377=CARTESIAN_POINT('Ctrl Pts',(91.4250587369798,26.5914696442962,1.89523793640893));
#19378=CARTESIAN_POINT('Ctrl Pts',(92.3674117349025,26.6290279897781,1.84257688132605));
#19379=CARTESIAN_POINT('Ctrl Pts',(93.1117466201966,26.2633574548232,1.78991582624318));
#19380=CARTESIAN_POINT('Ctrl Pts',(93.8560815054908,25.8976869198683,1.7372547711603));
#19381=CARTESIAN_POINT('Ctrl Pts',(94.4023982781564,25.1287875044768,1.68459371607742));
#19382=CARTESIAN_POINT('Ctrl Pts',(94.5029873847571,24.3057173158974,1.63193266099454));
#19383=CARTESIAN_POINT('Ctrl Pts',(94.6035764913578,23.4826471273179,1.57927160591166));
#19384=CARTESIAN_POINT('Ctrl Pts',(94.2584379318934,22.6054061655506,1.52661055082878));
#19385=CARTESIAN_POINT('Ctrl Pts',(93.6239876980049,22.0711235918099,1.4739494957459));
#19386=CARTESIAN_POINT('Ctrl Pts',(92.9895374641164,21.5368410180693,1.42128844066303));
#19387=CARTESIAN_POINT('Ctrl Pts',(92.0657755558037,21.3455168323553,1.36862738558015));
#19388=CARTESIAN_POINT('Ctrl Pts',(91.2718708195105,21.5853896272901,1.31596633049727));
#19389=CARTESIAN_POINT('Ctrl Pts',(90.4779660832174,21.8252624222249,1.26330527541439));
#19390=CARTESIAN_POINT('Ctrl Pts',(89.8139185189439,22.4963321978085,1.21064422033151));
#19391=CARTESIAN_POINT('Ctrl Pts',(89.5807319779765,23.2907318840645,1.15798316524864));
#19392=CARTESIAN_POINT('Ctrl Pts',(89.5137208066282,23.5190197315272,1.14284987766308));
#19393=CARTESIAN_POINT('Ctrl Pts',(89.4822911692266,23.7574924580249,1.12771659007753));
#19394=CARTESIAN_POINT('Ctrl Pts',(89.4843731420168,23.9964690566784,1.11258330249198));
#19395=CARTESIAN_POINT('Ctrl Pts',(89.4865042982783,24.0002742229179,1.38741669750802));
#19396=CARTESIAN_POINT('Ctrl Pts',(89.4868031422779,23.5689363684933,1.41458082386326));
#19397=CARTESIAN_POINT('Ctrl Pts',(89.5921777588412,23.1374323068698,1.4417449502185));
#19398=CARTESIAN_POINT('Ctrl Pts',(89.8017473998347,22.764501991722,1.46890907657374));
#19399=CARTESIAN_POINT('Ctrl Pts',(90.2080243499466,22.0415299509043,1.52157013165662));
#19400=CARTESIAN_POINT('Ctrl Pts',(91.0058940198741,21.5386936873713,1.57423118673949));
#19401=CARTESIAN_POINT('Ctrl Pts',(91.833390176038,21.4839126258589,1.62689224182237));
#19402=CARTESIAN_POINT('Ctrl Pts',(92.6608863322019,21.4291315643466,1.67955329690525));
#19403=CARTESIAN_POINT('Ctrl Pts',(93.5180089746021,21.8224057048548,1.73221435198813));
#19404=CARTESIAN_POINT('Ctrl Pts',(94.0160964783391,22.4854399019793,1.78487540707101));
#19405=CARTESIAN_POINT('Ctrl Pts',(94.5141839820761,23.1484740991037,1.83753646215389));
#19406=CARTESIAN_POINT('Ctrl Pts',(94.65323634715,24.0812683528445,1.89019751723676));
#19407=CARTESIAN_POINT('Ctrl Pts',(94.3701624990711,24.8607544964156,1.94285857231964));
#19408=CARTESIAN_POINT('Ctrl Pts',(94.0870886509922,25.6402406399868,1.99551962740252));
#19409=CARTESIAN_POINT('Ctrl Pts',(93.3818885897606,26.2664186733884,2.0481806824854));
#19410=CARTESIAN_POINT('Ctrl Pts',(92.5743965080578,26.4553208851494,2.10084173756828));
#19411=CARTESIAN_POINT('Ctrl Pts',(91.766904426355,26.6442230969105,2.15350279265116));
#19412=CARTESIAN_POINT('Ctrl Pts',(90.857120324181,26.3958494870309,2.20616384773403));
#19413=CARTESIAN_POINT('Ctrl Pts',(90.2576399987561,25.8228345233925,2.25882490281691));
#19414=CARTESIAN_POINT('Ctrl Pts',(89.7696876855645,25.3564239255092,2.30168883438061));
#19415=CARTESIAN_POINT('Ctrl Pts',(89.4873206236216,24.6749290158026,2.34455276594432));
#19416=CARTESIAN_POINT('Ctrl Pts',(89.4812641621455,23.9978903848741,2.38741669750802));
#19417=CARTESIAN_POINT('Origin',(92.,24.,5.));
#19418=CARTESIAN_POINT('',(89.4802712114252,24.0018289507128,3.38741669750802));
#19419=CARTESIAN_POINT('',(89.4854088326162,24.0015585716341,3.11258330249198));
#19420=CARTESIAN_POINT('',(89.4825,24.,5.));
#19421=CARTESIAN_POINT('Ctrl Pts',(89.4854088326162,24.0015585716341,3.11258330249198));
#19422=CARTESIAN_POINT('Ctrl Pts',(89.4836296984461,24.3124536014081,3.09298258440541));
#19423=CARTESIAN_POINT('Ctrl Pts',(89.5370773572355,24.6227586333045,3.07338186631883));
#19424=CARTESIAN_POINT('Ctrl Pts',(89.6485419638298,24.9105966710309,3.05378114823225));
#19425=CARTESIAN_POINT('Ctrl Pts',(89.9480128179958,25.6839282751438,3.00112009314937));
#19426=CARTESIAN_POINT('Ctrl Pts',(90.6662676183469,26.2950862932019,2.94845903806649));
#19427=CARTESIAN_POINT('Ctrl Pts',(91.4775657352138,26.466901288493,2.89579798298361));
#19428=CARTESIAN_POINT('Ctrl Pts',(92.2888638520807,26.638716283784,2.84313692790074));
#19429=CARTESIAN_POINT('Ctrl Pts',(93.1932052854633,26.371188256308,2.79047587281786));
#19430=CARTESIAN_POINT('Ctrl Pts',(93.7804553940471,25.7856433745947,2.73781481773498));
#19431=CARTESIAN_POINT('Ctrl Pts',(94.3677055026309,25.2000984928813,2.6851537626521));
#19432=CARTESIAN_POINT('Ctrl Pts',(94.6378642864158,24.2965367569306,2.63249270756922));
#19433=CARTESIAN_POINT('Ctrl Pts',(94.4684108772915,23.4847436484408,2.57983165248635));
#19434=CARTESIAN_POINT('Ctrl Pts',(94.2989574681671,22.672950539951,2.52717059740347));
#19435=CARTESIAN_POINT('Ctrl Pts',(93.6898918661335,21.952926058922,2.47450954232059));
#19436=CARTESIAN_POINT('Ctrl Pts',(92.9174341827593,21.6512037648828,2.42184848723771));
#19437=CARTESIAN_POINT('Ctrl Pts',(92.1449764993851,21.3494814708436,2.36918743215483));
#19438=CARTESIAN_POINT('Ctrl Pts',(91.2091267346702,21.4660613637942,2.31652637707196));
#19439=CARTESIAN_POINT('Ctrl Pts',(90.5343118592194,21.9480925468641,2.26386532198908));
#19440=CARTESIAN_POINT('Ctrl Pts',(89.8881204945621,22.4096774930868,2.21343798215671));
#19441=CARTESIAN_POINT('Ctrl Pts',(89.4812891226481,23.2063686712678,2.16301064232435));
#19442=CARTESIAN_POINT('Ctrl Pts',(89.4785876236681,24.0006455599548,2.11258330249198));
#19443=CARTESIAN_POINT('Ctrl Pts',(89.4812641621455,23.9978903848741,2.38741669750802));
#19444=CARTESIAN_POINT('Ctrl Pts',(89.47987987706,23.8431441716248,2.3972138210272));
#19445=CARTESIAN_POINT('Ctrl Pts',(89.4929303898819,23.6886307597355,2.40701094454637));
#19446=CARTESIAN_POINT('Ctrl Pts',(89.5212601912555,23.5369715569028,2.41680806806555));
#19447=CARTESIAN_POINT('Ctrl Pts',(89.6735372578558,22.7217798714484,2.46946912314842));
#19448=CARTESIAN_POINT('Ctrl Pts',(90.2672679397321,21.9890528179368,2.5221301782313));
#19449=CARTESIAN_POINT('Ctrl Pts',(91.0331836055545,21.6710928935685,2.57479123331418));
#19450=CARTESIAN_POINT('Ctrl Pts',(91.7990992713769,21.3531329692002,2.62745228839706));
#19451=CARTESIAN_POINT('Ctrl Pts',(92.7371999211453,21.4499401739753,2.68011334347994));
#19452=CARTESIAN_POINT('Ctrl Pts',(93.4220417006604,21.9176116335595,2.73277439856282));
#19453=CARTESIAN_POINT('Ctrl Pts',(94.1068834801755,22.3852830931437,2.78543545364569));
#19454=CARTESIAN_POINT('Ctrl Pts',(94.5384663894373,23.2238188075369,2.83809650872857));
#19455=CARTESIAN_POINT('Ctrl Pts',(94.5210598219411,24.052928105998,2.89075756381145));
#19456=CARTESIAN_POINT('Ctrl Pts',(94.5036532544448,24.8820374044591,2.94341861889433));
#19457=CARTESIAN_POINT('Ctrl Pts',(94.0372572101906,25.701720286988,2.99607967397721));
#19458=CARTESIAN_POINT('Ctrl Pts',(93.3333904465718,26.1402367801488,3.04874072906008));
#19459=CARTESIAN_POINT('Ctrl Pts',(92.629523682953,26.5787532733095,3.10140178414296));
#19460=CARTESIAN_POINT('Ctrl Pts',(91.6881861999696,26.636103377102,3.15406283922584));
#19461=CARTESIAN_POINT('Ctrl Pts',(90.9362905172017,26.2862777415508,3.20672389430872));
#19462=CARTESIAN_POINT('Ctrl Pts',(90.1843948344338,25.9364521059997,3.2593849493916));
#19463=CARTESIAN_POINT('Ctrl Pts',(89.6219409518814,25.1794507311049,3.31204600447447));
#19464=CARTESIAN_POINT('Ctrl Pts',(89.5040113501232,24.3585867079682,3.36470705955735));
#19465=CARTESIAN_POINT('Ctrl Pts',(89.4870592998501,24.2405898015078,3.37227693887424));
#19466=CARTESIAN_POINT('Ctrl Pts',(89.4792925695015,24.1212732846669,3.37984681819113));
#19467=CARTESIAN_POINT('Ctrl Pts',(89.4802712114252,24.0018289507128,3.38741669750802));
#19468=CARTESIAN_POINT('Origin',(92.,24.,5.));
#19469=CARTESIAN_POINT('',(89.4864157451591,24.0003542166096,4.38741669750802));
#19470=CARTESIAN_POINT('',(89.4839748093507,23.9978936309447,4.11258330249198));
#19471=CARTESIAN_POINT('',(89.4825,24.,5.));
#19472=CARTESIAN_POINT('Ctrl Pts',(89.4839748093507,23.9978936309447,4.11258330249198));
#19473=CARTESIAN_POINT('Ctrl Pts',(89.4886914413751,24.5834107418753,4.07561558156934));
#19474=CARTESIAN_POINT('Ctrl Pts',(89.6925942792401,25.1718904338737,4.0386478606467));
#19475=CARTESIAN_POINT('Ctrl Pts',(90.0662148873616,25.6183374708836,4.00168013972405));
#19476=CARTESIAN_POINT('Ctrl Pts',(90.5984428671593,26.2543077557916,3.94901908464118));
#19477=CARTESIAN_POINT('Ctrl Pts',(91.475069207756,26.6020594676883,3.8963580295583));
#19478=CARTESIAN_POINT('Ctrl Pts',(92.2985289056069,26.5038812863978,3.84369697447542));
#19479=CARTESIAN_POINT('Ctrl Pts',(93.1219886034578,26.4057031051072,3.79103591939255));
#19480=CARTESIAN_POINT('Ctrl Pts',(93.8922816585628,25.8615950306292,3.73837486430966));
#19481=CARTESIAN_POINT('Ctrl Pts',(94.2600670194833,25.1183193280089,3.68571380922678));
#19482=CARTESIAN_POINT('Ctrl Pts',(94.6278523804038,24.3750436253885,3.63305275414391));
#19483=CARTESIAN_POINT('Ctrl Pts',(94.5931300471397,23.4326002946258,3.58039169906103));
#19484=CARTESIAN_POINT('Ctrl Pts',(94.1716472007572,22.7184035364296,3.52773064397815));
#19485=CARTESIAN_POINT('Ctrl Pts',(93.7501643543746,22.0042067782334,3.47506958889527));
#19486=CARTESIAN_POINT('Ctrl Pts',(92.9419209948736,21.5182565926037,3.4224085338124));
#19487=CARTESIAN_POINT('Ctrl Pts',(92.113469258178,21.4809395463903,3.36974747872952));
#19488=CARTESIAN_POINT('Ctrl Pts',(91.2850175214825,21.4436225001769,3.31708642364664));
#19489=CARTESIAN_POINT('Ctrl Pts',(90.4363574075924,21.8549385933799,3.26442536856376));
#19490=CARTESIAN_POINT('Ctrl Pts',(89.9523708046377,22.5283492350652,3.21176431348088));
#19491=CARTESIAN_POINT('Ctrl Pts',(89.648526527872,22.9511129399696,3.17870397648458));
#19492=CARTESIAN_POINT('Ctrl Pts',(89.4884096805934,23.4771750052054,3.14564363948828));
#19493=CARTESIAN_POINT('Ctrl Pts',(89.4854088326162,24.0015585716341,3.11258330249198));
#19494=CARTESIAN_POINT('Ctrl Pts',(89.4802712114252,24.0018289507128,3.38741669750802));
#19495=CARTESIAN_POINT('Ctrl Pts',(89.4861006458386,23.2903400047058,3.43250787327401));
#19496=CARTESIAN_POINT('Ctrl Pts',(89.8022313189484,22.5743158820022,3.47759904904));
#19497=CARTESIAN_POINT('Ctrl Pts',(90.335679104099,22.105645314345,3.52269022480599));
#19498=CARTESIAN_POINT('Ctrl Pts',(90.9586817807967,21.5582946152368,3.57535127988887));
#19499=CARTESIAN_POINT('Ctrl Pts',(91.8780924551559,21.3483198883991,3.62801233497174));
#19500=CARTESIAN_POINT('Ctrl Pts',(92.6769427066419,21.5709482675317,3.68067339005462));
#19501=CARTESIAN_POINT('Ctrl Pts',(93.475792958128,21.7935766466644,3.7333344451375));
#19502=CARTESIAN_POINT('Ctrl Pts',(94.1540827867411,22.4488081317675,3.78599550022038));
#19503=CARTESIAN_POINT('Ctrl Pts',(94.4041961740691,23.2394840564229,3.83865655530326));
#19504=CARTESIAN_POINT('Ctrl Pts',(94.6543095613971,24.0301599810783,3.89131761038613));
#19505=CARTESIAN_POINT('Ctrl Pts',(94.4762465074402,24.9562803452861,3.94397866546901));
#19506=CARTESIAN_POINT('Ctrl Pts',(93.9507616486448,25.59783376143,3.99663972055189));
#19507=CARTESIAN_POINT('Ctrl Pts',(93.4252767898494,26.2393871775739,4.04930077563477));
#19508=CARTESIAN_POINT('Ctrl Pts',(92.5523701262155,26.596373645654,4.10196183071765));
#19509=CARTESIAN_POINT('Ctrl Pts',(91.7279197254964,26.5068937086739,4.15462288580053));
#19510=CARTESIAN_POINT('Ctrl Pts',(90.9034693247774,26.4174137716938,4.2072839408834));
#19511=CARTESIAN_POINT('Ctrl Pts',(90.1274751869731,25.8814674296536,4.25994499596628));
#19512=CARTESIAN_POINT('Ctrl Pts',(89.7518638973824,25.1421154958357,4.31260605104916));
#19513=CARTESIAN_POINT('Ctrl Pts',(89.5739985954225,24.7920060646031,4.33754293320211));
#19514=CARTESIAN_POINT('Ctrl Pts',(89.4859135120177,24.3962857922303,4.36247981535507));
#19515=CARTESIAN_POINT('Ctrl Pts',(89.4864157451591,24.0003542166096,4.38741669750802));
#19516=CARTESIAN_POINT('Origin',(92.,24.,5.));
#19517=CARTESIAN_POINT('',(89.4815253774702,23.997843907913,5.38741669750803));
#19518=CARTESIAN_POINT('',(89.4784999401586,24.000477759641,5.11258330249198));
#19519=CARTESIAN_POINT('',(89.4825,24.,5.));
#19520=CARTESIAN_POINT('Ctrl Pts',(89.4784999401586,24.000477759641,5.11258330249198));
#19521=CARTESIAN_POINT('Ctrl Pts',(89.4784306610618,24.0268374600631,5.11090963381615));
#19522=CARTESIAN_POINT('Ctrl Pts',(89.478808621275,24.0531951260583,5.10923596514032));
#19523=CARTESIAN_POINT('Ctrl Pts',(89.4796399750106,24.0795384836878,5.1075622964645));
#19524=CARTESIAN_POINT('Ctrl Pts',(89.5057980584424,24.9084175965175,5.05490124138162));
#19525=CARTESIAN_POINT('Ctrl Pts',(89.9808208362983,25.7231312660314,5.00224018629874));
#19526=CARTESIAN_POINT('Ctrl Pts',(90.6892773720313,26.1541929390351,4.94957913121586));
#19527=CARTESIAN_POINT('Ctrl Pts',(91.3977339077644,26.5852546120388,4.89691807613298));
#19528=CARTESIAN_POINT('Ctrl Pts',(92.3396242013746,26.6326642885323,4.84425702105011));
#19529=CARTESIAN_POINT('Ctrl Pts',(93.0877849303764,26.2749208713486,4.79159596596723));
#19530=CARTESIAN_POINT('Ctrl Pts',(93.8359456593782,25.9171774541649,4.73893491088435));
#19531=CARTESIAN_POINT('Ctrl Pts',(94.3903768237715,25.1542809433041,4.68627385580147));
#19532=CARTESIAN_POINT('Ctrl Pts',(94.4996344284721,24.3322179256395,4.63361280071859));
#19533=CARTESIAN_POINT('Ctrl Pts',(94.6088920331728,23.5101549079749,4.58095174563571));
#19534=CARTESIAN_POINT('Ctrl Pts',(94.2729760781807,22.6289253835066,4.52829069055284));
#19535=CARTESIAN_POINT('Ctrl Pts',(93.6442301819934,22.0881819816233,4.47562963546996));
#19536=CARTESIAN_POINT('Ctrl Pts',(93.0154842858062,21.5474385797399,4.42296858038708));
#19537=CARTESIAN_POINT('Ctrl Pts',(92.0939084484237,21.3471813004415,4.3703075253042));
#19538=CARTESIAN_POINT('Ctrl Pts',(91.2974530394867,21.5782302356247,4.31764647022133));
#19539=CARTESIAN_POINT('Ctrl Pts',(90.5009976305497,21.8092791708079,4.26498541513845));
#19540=CARTESIAN_POINT('Ctrl Pts',(89.8296626500582,22.4716343204727,4.21232436005557));
#19541=CARTESIAN_POINT('Ctrl Pts',(89.5879099693118,23.2649063242647,4.15966330497269));
#19542=CARTESIAN_POINT('Ctrl Pts',(89.5158661107693,23.5013064992303,4.14396997081245));
#19543=CARTESIAN_POINT('Ctrl Pts',(89.481972530589,23.749333117907,4.12827663665222));
#19544=CARTESIAN_POINT('Ctrl Pts',(89.4839748093507,23.9978936309447,4.11258330249198));
#19545=CARTESIAN_POINT('Ctrl Pts',(89.4864157451591,24.0003542166096,4.38741669750802));
#19546=CARTESIAN_POINT('Ctrl Pts',(89.4869741148213,23.5601678531502,4.41514087043795));
#19547=CARTESIAN_POINT('Ctrl Pts',(89.5970300437706,23.1197203102035,4.44286504336787));
#19548=CARTESIAN_POINT('Ctrl Pts',(89.8149442483522,22.7413995457469,4.47058921629779));
#19549=CARTESIAN_POINT('Ctrl Pts',(90.22886433029,22.0227930550715,4.52325027138067));
#19550=CARTESIAN_POINT('Ctrl Pts',(91.0319329355429,21.5283375993164,4.57591132646355));
#19551=CARTESIAN_POINT('Ctrl Pts',(91.8599447465539,21.4822771662391,4.62857238154643));
#19552=CARTESIAN_POINT('Ctrl Pts',(92.6879565575648,21.4362167331619,4.68123343662931));
#19553=CARTESIAN_POINT('Ctrl Pts',(93.5409115743339,21.8385513227625,4.73389449171218));
#19554=CARTESIAN_POINT('Ctrl Pts',(94.0319801400905,22.5068153323074,4.78655554679506));
#19555=CARTESIAN_POINT('Ctrl Pts',(94.523048705847,23.1750793418523,4.83921660187794));
#19556=CARTESIAN_POINT('Ctrl Pts',(94.652230820591,24.1092727713413,4.89187765696082));
#19557=CARTESIAN_POINT('Ctrl Pts',(94.3609401906911,24.8857229575283,4.9445387120437));
#19558=CARTESIAN_POINT('Ctrl Pts',(94.0696495607912,25.6621731437152,4.99719976712658));
#19559=CARTESIAN_POINT('Ctrl Pts',(93.3578861862475,26.2808800866,5.04986082220945));
#19560=CARTESIAN_POINT('Ctrl Pts',(92.5484469044027,26.461249628667,5.10252187729233));
#19561=CARTESIAN_POINT('Ctrl Pts',(91.7390076225579,26.641619170734,5.15518293237521));
#19562=CARTESIAN_POINT('Ctrl Pts',(90.8318924334121,26.3836513119832,5.20784398745809));
#19563=CARTESIAN_POINT('Ctrl Pts',(90.2384935561441,25.8043388788684,5.26050504254097));
#19564=CARTESIAN_POINT('Ctrl Pts',(89.7618020463167,25.3389633465204,5.30280892752999));
#19565=CARTESIAN_POINT('Ctrl Pts',(89.4875608688215,24.6662147404431,5.34511281251901));
#19566=CARTESIAN_POINT('Ctrl Pts',(89.4815253774702,23.997843907913,5.38741669750803));
#19567=CARTESIAN_POINT('Origin',(92.,24.,5.));
#19568=CARTESIAN_POINT('',(89.4800390583838,24.0017354239359,6.38741669750802));
#19569=CARTESIAN_POINT('',(89.4852339904214,24.0016589574482,6.11258330249198));
#19570=CARTESIAN_POINT('',(89.4825,24.,5.));
#19571=CARTESIAN_POINT('Ctrl Pts',(89.4852339904214,24.0016589574482,6.11258330249198));
#19572=CARTESIAN_POINT('Ctrl Pts',(89.4833859739972,24.3036180412943,6.09354263098009));
#19573=CARTESIAN_POINT('Ctrl Pts',(89.5337383064255,24.6049815306727,6.0745019594682));
#19574=CARTESIAN_POINT('Ctrl Pts',(89.6390603134631,24.8857227683913,6.05546128795631));
#19575=CARTESIAN_POINT('Ctrl Pts',(89.9303508811609,25.6621727887753,6.00280023287343));
#19576=CARTESIAN_POINT('Ctrl Pts',(90.642114103715,26.2808795995417,5.95013917779054));
#19577=CARTESIAN_POINT('Ctrl Pts',(91.4515532127125,26.4612491030927,5.89747812270766));
#19578=CARTESIAN_POINT('Ctrl Pts',(92.2609923217099,26.6416186066436,5.84481706762479));
#19579=CARTESIAN_POINT('Ctrl Pts',(93.1681073171506,26.3836508029792,5.79215601254192));
#19580=CARTESIAN_POINT('Ctrl Pts',(93.7615060677044,25.8043384935705,5.73949495745904));
#19581=CARTESIAN_POINT('Ctrl Pts',(94.3549048182582,25.2250261841617,5.68683390237616));
#19582=CARTESIAN_POINT('Ctrl Pts',(94.6345873239251,24.3243693690088,5.63417284729328));
#19583=CARTESIAN_POINT('Ctrl Pts',(94.4737127953066,23.5108312844466,5.5815117922104));
#19584=CARTESIAN_POINT('Ctrl Pts',(94.3128382666882,22.6972931998845,5.52885073712752));
#19585=CARTESIAN_POINT('Ctrl Pts',(93.7114067037844,21.9708738459131,5.47618968204464));
#19586=CARTESIAN_POINT('Ctrl Pts',(92.9421775844463,21.6610167966983,5.42352862696176));
#19587=CARTESIAN_POINT('Ctrl Pts',(92.1729484651082,21.3511597474835,5.37086757187889));
#19588=CARTESIAN_POINT('Ctrl Pts',(91.2359217893358,21.4578650030252,5.31820651679601));
#19589=CARTESIAN_POINT('Ctrl Pts',(90.5560551459534,21.9327399088688,5.26554546171313));
#19590=CARTESIAN_POINT('Ctrl Pts',(89.8977959599792,22.3925223853337,5.21455807530608));
#19591=CARTESIAN_POINT('Ctrl Pts',(89.4806104893556,23.1974441303418,5.16357068889903));
#19592=CARTESIAN_POINT('Ctrl Pts',(89.4784999401586,24.000477759641,5.11258330249198));
#19593=CARTESIAN_POINT('Ctrl Pts',(89.4815253774702,23.997843907913,5.38741669750803));
#19594=CARTESIAN_POINT('Ctrl Pts',(89.4800477209726,23.8342080999941,5.39777386760188));
#19595=CARTESIAN_POINT('Ctrl Pts',(89.4946464973945,23.6708346988265,5.40813103769574));
#19596=CARTESIAN_POINT('Ctrl Pts',(89.5262866764575,23.5108311799897,5.4184882077896));
#19597=CARTESIAN_POINT('Ctrl Pts',(89.6871612394291,22.6972929217049,5.47114926287248));
#19598=CARTESIAN_POINT('Ctrl Pts',(90.2885929307624,21.9708734126142,5.52381031795536));
#19599=CARTESIAN_POINT('Ctrl Pts',(91.0578222143614,21.6610162972326,5.57647137303823));
#19600=CARTESIAN_POINT('Ctrl Pts',(91.8270514979604,21.351159181851,5.62913242812111));
#19601=CARTESIAN_POINT('Ctrl Pts',(92.7640783738252,21.4578644601784,5.68179348320399));
#19602=CARTESIAN_POINT('Ctrl Pts',(93.4439451623861,21.9327394674267,5.73445453828687));
#19603=CARTESIAN_POINT('Ctrl Pts',(94.123811950947,22.407614474675,5.78711559336975));
#19604=CARTESIAN_POINT('Ctrl Pts',(94.5465186522039,23.2506592108443,5.83977664845263));
#19605=CARTESIAN_POINT('Ctrl Pts',(94.5203605631863,24.0795385006725,5.8924377035355));
#19606=CARTESIAN_POINT('Ctrl Pts',(94.4942024741687,24.9084177905007,5.94509875861838));
#19607=CARTESIAN_POINT('Ctrl Pts',(94.0191795948766,25.7231316339878,5.99775981370126));
#19608=CARTESIAN_POINT('Ctrl Pts',(93.3107229078599,26.1541933990406,6.05042086878414));
#19609=CARTESIAN_POINT('Ctrl Pts',(92.6022662208433,26.5852551640933,6.10308192386702));
#19610=CARTESIAN_POINT('Ctrl Pts',(91.6603757261022,26.6326648507116,6.1557429789499));
#19611=CARTESIAN_POINT('Ctrl Pts',(90.9122148373384,26.274921357135,6.20840403403277));
#19612=CARTESIAN_POINT('Ctrl Pts',(90.1640539485746,25.9171778635584,6.26106508911565));
#19613=CARTESIAN_POINT('Ctrl Pts',(89.6096226657881,25.154281189787,6.31372614419853));
#19614=CARTESIAN_POINT('Ctrl Pts',(89.5003650377567,24.3322179965802,6.36638719928141));
#19615=CARTESIAN_POINT('Ctrl Pts',(89.4858215065436,24.2227912963587,6.37339703202361));
#19616=CARTESIAN_POINT('Ctrl Pts',(89.4791659526656,24.1123162318431,6.38040686476582));
#19617=CARTESIAN_POINT('Ctrl Pts',(89.4800390583838,24.0017354239359,6.38741669750802));
#19618=CARTESIAN_POINT('Origin',(92.,24.,5.));
#19619=CARTESIAN_POINT('',(89.4863706869161,24.0004946014336,7.38741669750802));
#19620=CARTESIAN_POINT('',(89.4842076940747,23.9979483279393,7.11258330249198));
#19621=CARTESIAN_POINT('',(89.4825,24.,5.));
#19622=CARTESIAN_POINT('Ctrl Pts',(89.4842076940747,23.9979483279393,7.11258330249198));
#19623=CARTESIAN_POINT('Ctrl Pts',(89.4887014564202,24.5747302879618,7.07617562814402));
#19624=CARTESIAN_POINT('Ctrl Pts',(89.6859403589103,25.1542900307673,7.03976795379607));
#19625=CARTESIAN_POINT('Ctrl Pts',(90.0492387679223,25.5978334202261,7.00336027944811));
#19626=CARTESIAN_POINT('Ctrl Pts',(90.5747235145078,26.23938669937,6.95069922436523));
#19627=CARTESIAN_POINT('Ctrl Pts',(91.4476299917373,26.5963730912254,6.89803816928235));
#19628=CARTESIAN_POINT('Ctrl Pts',(92.2720802164025,26.5068931733543,6.84537711419947));
#19629=CARTESIAN_POINT('Ctrl Pts',(93.0965304410677,26.4174132554832,6.79271605911659));
#19630=CARTESIAN_POINT('Ctrl Pts',(93.8725244131686,25.8814670278857,6.74005500403372));
#19631=CARTESIAN_POINT('Ctrl Pts',(94.248135622552,25.142115251948,6.68739394895084));
#19632=CARTESIAN_POINT('Ctrl Pts',(94.6237468319354,24.4027634760103,6.63473289386796));
#19633=CARTESIAN_POINT('Ctrl Pts',(94.5989752786014,23.4600061517323,6.58207183878508));
#19634=CARTESIAN_POINT('Ctrl Pts',(94.1850552850516,22.7413998145083,6.52941078370221));
#19635=CARTESIAN_POINT('Ctrl Pts',(93.7711352915018,22.0227934772843,6.47674972861933));
#19636=CARTESIAN_POINT('Ctrl Pts',(92.9680668577363,21.5283381271142,6.42408867353645));
#19637=CARTESIAN_POINT('Ctrl Pts',(92.1400552235388,21.4822777038725,6.37142761845357));
#19638=CARTESIAN_POINT('Ctrl Pts',(91.3120435893413,21.4362172806308,6.31876656337069));
#19639=CARTESIAN_POINT('Ctrl Pts',(90.4590887547119,21.8385517843175,6.26610550828781));
#19640=CARTESIAN_POINT('Ctrl Pts',(89.9680202938179,22.5068156511616,6.21344445320493));
#19641=CARTESIAN_POINT('Ctrl Pts',(89.6545075852539,22.9334551762256,6.17982406963395));
#19642=CARTESIAN_POINT('Ctrl Pts',(89.4884970592155,23.4684855231337,6.14620368606297));
#19643=CARTESIAN_POINT('Ctrl Pts',(89.4852339904214,24.0016589574482,6.11258330249198));
#19644=CARTESIAN_POINT('Ctrl Pts',(89.4800390583838,24.0017354239359,6.38741669750802));
#19645=CARTESIAN_POINT('Ctrl Pts',(89.4857251203391,23.2815828562451,6.4330679198487));
#19646=CARTESIAN_POINT('Ctrl Pts',(89.81071724972,22.5569454920104,6.47871914218937));
#19647=CARTESIAN_POINT('Ctrl Pts',(90.3557694668982,22.0881815733762,6.52437036453004));
#19648=CARTESIAN_POINT('Ctrl Pts',(90.9845154973476,21.5474380560208,6.57703141961292));
#19649=CARTESIAN_POINT('Ctrl Pts',(91.906091531523,21.3471807339522,6.6296924746958));
#19650=CARTESIAN_POINT('Ctrl Pts',(92.7025471105349,21.578229718477,6.68235352977867));
#19651=CARTESIAN_POINT('Ctrl Pts',(93.4990026895468,21.8092787030019,6.73501458486155));
#19652=CARTESIAN_POINT('Ctrl Pts',(94.1703378133953,22.4716339941201,6.78767563994444));
#19653=CARTESIAN_POINT('Ctrl Pts',(94.4120905457653,23.2649061673003,6.84033669502731));
#19654=CARTESIAN_POINT('Ctrl Pts',(94.6538432781353,24.0581783404805,6.89299775011019));
#19655=CARTESIAN_POINT('Ctrl Pts',(94.4660136190268,24.9823673957227,6.94565880519307));
#19656=CARTESIAN_POINT('Ctrl Pts',(93.9337855255779,25.6183378164487,6.99831986027595));
#19657=CARTESIAN_POINT('Ctrl Pts',(93.401557432129,26.2543082371747,7.05098091535882));
#19658=CARTESIAN_POINT('Ctrl Pts',(92.5249309043398,26.6020600233844,7.1036419704417));
#19659=CARTESIAN_POINT('Ctrl Pts',(91.7014710306461,26.5038818211034,7.15630302552458));
#19660=CARTESIAN_POINT('Ctrl Pts',(90.8780111569526,26.4057036188225,7.20896408060746));
#19661=CARTESIAN_POINT('Ctrl Pts',(90.1077179373546,25.8615954280509,7.26162513569034));
#19662=CARTESIAN_POINT('Ctrl Pts',(89.7399324979007,25.1183195667607,7.31428619077322));
#19663=CARTESIAN_POINT('Ctrl Pts',(89.5696843862451,24.7742567022501,7.33866302635148));
#19664=CARTESIAN_POINT('Ctrl Pts',(89.4856844315082,24.3875167881334,7.36303986192975));
#19665=CARTESIAN_POINT('Ctrl Pts',(89.4863706869161,24.0004946014336,7.38741669750802));
#19666=CARTESIAN_POINT('Origin',(92.,24.,5.));
#19667=CARTESIAN_POINT('',(89.481789046694,23.9978055657336,8.38741669750803));
#19668=CARTESIAN_POINT('',(89.4784369335473,24.0003195913806,8.11258330249199));
#19669=CARTESIAN_POINT('',(89.4825,24.,5.));
#19670=CARTESIAN_POINT('Ctrl Pts',(89.4784369335473,24.0003195913806,8.11258330249199));
#19671=CARTESIAN_POINT('Ctrl Pts',(89.4784053094568,24.0178575771478,8.11146968039084));
#19672=CARTESIAN_POINT('Ctrl Pts',(89.4785726200148,24.0353949438105,8.1103560582897));
#19673=CARTESIAN_POINT('Ctrl Pts',(89.4789407162088,24.0529280950311,8.10924243618855));
#19674=CARTESIAN_POINT('Ctrl Pts',(89.4963472798269,24.8820372167501,8.05658138110567));
#19675=CARTESIAN_POINT('Ctrl Pts',(89.9627432248613,25.7017199235892,8.00392032602279));
#19676=CARTESIAN_POINT('Ctrl Pts',(90.6666098382641,26.1402363229507,7.95125927093991));
#19677=CARTESIAN_POINT('Ctrl Pts',(91.3704764516668,26.5787527223122,7.89859821585703));
#19678=CARTESIAN_POINT('Ctrl Pts',(92.3118137334378,26.6361028141961,7.84593716077416));
#19679=CARTESIAN_POINT('Ctrl Pts',(93.0637092555993,26.2862772534286,7.79327610569129));
#19680=CARTESIAN_POINT('Ctrl Pts',(93.8156047777607,25.9364516926611,7.74061505060841));
#19681=CARTESIAN_POINT('Ctrl Pts',(94.3780585403126,25.1794504792422,7.68795399552552));
#19682=CARTESIAN_POINT('Ctrl Pts',(94.495988116913,24.3585866313503,7.63529294044264));
#19683=CARTESIAN_POINT('Ctrl Pts',(94.6139176935135,23.5377227834583,7.58263188535976));
#19684=CARTESIAN_POINT('Ctrl Pts',(94.2873230841625,22.6529963010933,7.52997083027689));
#19685=CARTESIAN_POINT('Ctrl Pts',(93.6643205404874,22.105645718888,7.47730977519401));
#19686=CARTESIAN_POINT('Ctrl Pts',(93.0413179968122,21.5582951366827,7.42464872011114));
#19687=CARTESIAN_POINT('Ctrl Pts',(92.1219075188129,21.3483204546372,7.37198766502826));
#19688=CARTESIAN_POINT('Ctrl Pts',(91.32305743792,21.5709487862187,7.31932660994538));
#19689=CARTESIAN_POINT('Ctrl Pts',(90.524207357027,21.7935771178002,7.2666655548625));
#19690=CARTESIAN_POINT('Ctrl Pts',(89.8459176732405,22.4488084630088,7.21400449977962));
#19691=CARTESIAN_POINT('Ctrl Pts',(89.595804339318,23.2394842188293,7.16134344469674));
#19692=CARTESIAN_POINT('Ctrl Pts',(89.5186090146758,23.4835194755668,7.14509006396182));
#19693=CARTESIAN_POINT('Ctrl Pts',(89.4822015557634,23.740457099368,7.1288366832269));
#19694=CARTESIAN_POINT('Ctrl Pts',(89.4842076940747,23.9979483279393,7.11258330249198));
#19695=CARTESIAN_POINT('Ctrl Pts',(89.4863706869161,24.0004946014336,7.38741669750802));
#19696=CARTESIAN_POINT('Ctrl Pts',(89.4871669427931,23.5514362957882,7.41570091701263));
#19697=CARTESIAN_POINT('Ctrl Pts',(89.6019741159521,23.1019979736551,7.44398513651724));
#19698=CARTESIAN_POINT('Ctrl Pts',(89.828352335515,22.7184032628621,7.47226935602185));
#19699=CARTESIAN_POINT('Ctrl Pts',(90.249835271893,22.0042063520624,7.52493041110472));
#19700=CARTESIAN_POINT('Ctrl Pts',(91.058078803959,21.5182560622716,7.5775914661876));
#19701=CARTESIAN_POINT('Ctrl Pts',(91.8865307175797,21.4809390082697,7.63025252127048));
#19702=CARTESIAN_POINT('Ctrl Pts',(92.7149826312004,21.4436219542678,7.68291357635336));
#19703=CARTESIAN_POINT('Ctrl Pts',(93.5636429263759,21.8549381360548,7.73557463143624));
#19704=CARTESIAN_POINT('Ctrl Pts',(94.0476296326406,22.5283489211969,7.78823568651912));
#19705=CARTESIAN_POINT('Ctrl Pts',(94.5316163389053,23.2017597063389,7.840896741602));
#19706=CARTESIAN_POINT('Ctrl Pts',(94.6509294562594,24.1372650948361,7.89355779668487));
#19707=CARTESIAN_POINT('Ctrl Pts',(94.3514585382347,24.910596864736,7.94621885176775));
#19708=CARTESIAN_POINT('Ctrl Pts',(94.05198762021,25.6839286346359,7.99887990685063));
#19709=CARTESIAN_POINT('Ctrl Pts',(93.3337326668065,26.2950867859384,8.05154096193351));
#19710=CARTESIAN_POINT('Ctrl Pts',(92.5224343764949,26.4669018166948,8.10420201701639));
#19711=CARTESIAN_POINT('Ctrl Pts',(91.7111360861833,26.6387168474511,8.15686307209927));
#19712=CARTESIAN_POINT('Ctrl Pts',(90.8067944589634,26.3711887576613,8.20952412718214));
#19713=CARTESIAN_POINT('Ctrl Pts',(90.2195442254209,25.7856437531992,8.26218518226502));
#19714=CARTESIAN_POINT('Ctrl Pts',(89.7540374326078,25.3214886766988,8.30392902067936));
#19715=CARTESIAN_POINT('Ctrl Pts',(89.4877768657504,24.6575058177296,8.34567285909369));
#19716=CARTESIAN_POINT('Ctrl Pts',(89.481789046694,23.9978055657336,8.38741669750803));
#19717=CARTESIAN_POINT('Origin',(92.,24.,5.));
#19718=CARTESIAN_POINT('',(89.4798237559162,24.0015869167785,9.38741669750802));
#19719=CARTESIAN_POINT('',(89.4850510509789,24.0017493960693,9.11258330249199));
#19720=CARTESIAN_POINT('',(89.4825,24.,5.));
#19721=CARTESIAN_POINT('',(93.9134659966651,25.6359872033749,10.));
#19722=CARTESIAN_POINT('Ctrl Pts',(89.4798237559162,24.0015869167785,9.38741669750802));
#19723=CARTESIAN_POINT('Ctrl Pts',(89.4853060534862,23.272907237615,9.43362796642338));
#19724=CARTESIAN_POINT('Ctrl Pts',(89.8192670107975,22.5399678433785,9.47983923533874));
#19725=CARTESIAN_POINT('Ctrl Pts',(90.3760117641787,22.0711228370539,9.5260505042541));
#19726=CARTESIAN_POINT('Ctrl Pts',(91.0104623389641,21.5368403279841,9.57871155933698));
#19727=CARTESIAN_POINT('Ctrl Pts',(91.9342252311205,21.3455170498785,9.63137261441985));
#19728=CARTESIAN_POINT('Ctrl Pts',(92.7281294273515,21.5853893188973,9.68403366950273));
#19729=CARTESIAN_POINT('Ctrl Pts',(93.5220336235825,21.8252615879162,9.73669472458561));
#19730=CARTESIAN_POINT('Ctrl Pts',(94.1860791238883,22.4963294040593,9.78935577966849));
#19731=CARTESIAN_POINT('Ctrl Pts',(94.4192657381557,23.2907292988926,9.84201683475137));
#19732=CARTESIAN_POINT('Ctrl Pts',(94.6524523524231,24.0851291937258,9.89467788983425));
#19733=CARTESIAN_POINT('Ctrl Pts',(94.4547800806522,25.0028611672492,9.94733894491712));
#19734=CARTESIAN_POINT('Ctrl Pts',(93.9134659966651,25.6359872033749,10.));
#19735=CARTESIAN_POINT('',(90.0828969142745,25.6385343069379,10.));
#19736=CARTESIAN_POINT('Origin',(92.,24.,10.));
#19737=CARTESIAN_POINT('Ctrl Pts',(90.0828884583321,25.6385402287508,10.));
#19738=CARTESIAN_POINT('Ctrl Pts',(90.6060432359258,26.2476961579692,9.94901908464118));
#19739=CARTESIAN_POINT('Ctrl Pts',(91.4465813967719,26.5878273311312,9.89803816928235));
#19740=CARTESIAN_POINT('Ctrl Pts',(92.2457357659029,26.5094848424925,9.84705725392353));
#19741=CARTESIAN_POINT('Ctrl Pts',(93.0712272651497,26.4285604793168,9.79439619884065));
#19742=CARTESIAN_POINT('Ctrl Pts',(93.8525623160909,25.9011252999797,9.74173514375777));
#19743=CARTESIAN_POINT('Ctrl Pts',(94.2358877550497,25.1658537096528,9.68907408867489));
#19744=CARTESIAN_POINT('Ctrl Pts',(94.6192131940086,24.4305821193258,9.63641303359201));
#19745=CARTESIAN_POINT('Ctrl Pts',(94.6045290209851,23.487474118009,9.58375197850914));
#19746=CARTESIAN_POINT('Ctrl Pts',(94.1982521612179,22.7645021442661,9.53109092342626));
#19747=CARTESIAN_POINT('Ctrl Pts',(93.7919753014507,22.0415301705231,9.47842986834338));
#19748=CARTESIAN_POINT('Ctrl Pts',(92.9941057549398,21.5386942243541,9.4257688132605));
#19749=CARTESIAN_POINT('Ctrl Pts',(92.1666097685102,21.4839132228271,9.37310775817762));
#19750=CARTESIAN_POINT('Ctrl Pts',(91.3391137820805,21.4291322213001,9.32044670309475));
#19751=CARTESIAN_POINT('Ctrl Pts',(90.4819913557323,21.8224061644151,9.26778564801188));
#19752=CARTESIAN_POINT('Ctrl Pts',(89.983903964328,22.4854401936109,9.215124592929));
#19753=CARTESIAN_POINT('Ctrl Pts',(89.6606130378258,22.9157921545326,9.18094416278333));
#19754=CARTESIAN_POINT('Ctrl Pts',(89.4885781648624,23.4597899774222,9.14676373263766));
#19755=CARTESIAN_POINT('Ctrl Pts',(89.4850510509789,24.0017493960693,9.11258330249199));
#19756=CARTESIAN_POINT('Origin',(92.,24.,12.2084234471775));
#19757=CARTESIAN_POINT('',(88.9217235596202,24.0007881344672,1.79157655282254));
#19758=CARTESIAN_POINT('',(88.9313886636577,24.0003347861522,1.70842344717745));
#19759=CARTESIAN_POINT('',(88.9265,24.0000000000001,12.2084234471775));
#19760=CARTESIAN_POINT('',(92.7937992825328,21.0307770462543,0.999999999999999));
#19761=CARTESIAN_POINT('Ctrl Pts',(88.9313886636577,24.0003347861522,1.70842344717745));
#19762=CARTESIAN_POINT('Ctrl Pts',(88.9310462111061,24.4946152436419,1.68292651844981));
#19763=CARTESIAN_POINT('Ctrl Pts',(89.2764428698256,26.0092287095088,1.6047685346393));
#19764=CARTESIAN_POINT('Ctrl Pts',(91.6460838412789,27.6088416124303,1.47394949574591));
#19765=CARTESIAN_POINT('Ctrl Pts',(94.8312245109702,26.2698537574842,1.31596633049727));
#19766=CARTESIAN_POINT('Ctrl Pts',(95.4433138069375,22.8667064664957,1.15798316524863));
#19767=CARTESIAN_POINT('Ctrl Pts',(93.7762533017603,21.2934286920664,1.05266105508288));
#19768=CARTESIAN_POINT('Ctrl Pts',(92.7937992825328,21.0307770462543,0.999999999999999));
#19769=CARTESIAN_POINT('',(91.2062007174671,21.0307770462543,1.));
#19770=CARTESIAN_POINT('Origin',(92.,24.,0.999999999999999));
#19771=CARTESIAN_POINT('Ctrl Pts',(88.9217235596202,24.0007881344672,1.79157655282254));
#19772=CARTESIAN_POINT('Ctrl Pts',(88.921577466321,24.0437415214614,1.78934283757203));
#19773=CARTESIAN_POINT('Ctrl Pts',(88.9417780704225,25.0992023014299,1.73444806723864));
#19774=CARTESIAN_POINT('Ctrl Pts',(90.1476051992024,27.1179528805983,1.62689224182238));
#19775=CARTESIAN_POINT('Ctrl Pts',(93.5990315417431,27.2555126520044,1.46890907657374));
#19776=CARTESIAN_POINT('Ctrl Pts',(95.5999506290772,24.4393708209746,1.3109259113251));
#19777=CARTESIAN_POINT('Ctrl Pts',(94.349302755893,21.2605908411106,1.15462288580053));
#19778=CARTESIAN_POINT('Ctrl Pts',(92.1519058776305,20.7745943222177,1.05098091535883));
#19779=CARTESIAN_POINT('Ctrl Pts',(91.2042984301044,21.0256873776386,1.));
#19780=CARTESIAN_POINT('Origin',(92.,24.,12.2084234471775));
#19781=CARTESIAN_POINT('',(88.9300512599983,24.0019027884479,2.79157655282254));
#19782=CARTESIAN_POINT('',(88.924991222385,23.997424467889,2.70842344717745));
#19783=CARTESIAN_POINT('',(88.9265,24.0000000000001,12.2084234471775));
#19784=CARTESIAN_POINT('Ctrl Pts',(88.924991222385,23.997424467889,2.70842344717745));
#19785=CARTESIAN_POINT('Ctrl Pts',(88.9323852777363,24.823989803404,2.66555951561375));
#19786=CARTESIAN_POINT('Ctrl Pts',(89.7006356086327,26.6781674340519,2.57003452896717));
#19787=CARTESIAN_POINT('Ctrl Pts',(92.8261379115921,27.5314383230663,2.42184848723771));
#19788=CARTESIAN_POINT('Ctrl Pts',(95.4089769044768,25.2380224116542,2.26386532198907));
#19789=CARTESIAN_POINT('Ctrl Pts',(94.8996889870333,21.8216055629487,2.10588215674044));
#19790=CARTESIAN_POINT('Ctrl Pts',(91.760424111462,20.3812146145649,1.94789899149181));
#19791=CARTESIAN_POINT('Ctrl Pts',(89.3097988736992,21.9256563753203,1.81541275497081));
#19792=CARTESIAN_POINT('Ctrl Pts',(88.9317535085566,23.473734231803,1.73558757353269));
#19793=CARTESIAN_POINT('Ctrl Pts',(88.9313886636577,24.0003347861522,1.70842344717745));
#19794=CARTESIAN_POINT('Ctrl Pts',(88.9300512599983,24.0019027884479,2.79157655282254));
#19795=CARTESIAN_POINT('Ctrl Pts',(88.9278791968914,24.3814602359197,2.77197583473597));
#19796=CARTESIAN_POINT('Ctrl Pts',(89.1684423216005,25.77811538933,2.69971406156651));
#19797=CARTESIAN_POINT('Ctrl Pts',(91.2485917195107,27.5481000558719,2.57479123331418));
#19798=CARTESIAN_POINT('Ctrl Pts',(94.5607983477153,26.5682620509694,2.41680806806555));
#19799=CARTESIAN_POINT('Ctrl Pts',(95.5502716608786,23.2589111130017,2.25882490281691));
#19800=CARTESIAN_POINT('Ctrl Pts',(93.3195310914442,20.621776762524,2.10084173756828));
#19801=CARTESIAN_POINT('Ctrl Pts',(89.9403860022537,21.0427207939439,1.94509228757016));
#19802=CARTESIAN_POINT('Ctrl Pts',(88.9250216955149,23.0310920004536,1.84200389265491));
#19803=CARTESIAN_POINT('Ctrl Pts',(88.9217235596202,24.0007881344672,1.79157655282254));
#19804=CARTESIAN_POINT('Origin',(92.,24.,12.2084234471775));
#19805=CARTESIAN_POINT('',(88.9283005269272,23.9974284308675,3.79157655282254));
#19806=CARTESIAN_POINT('',(88.9237789745047,24.0022328818336,3.70842344717745));
#19807=CARTESIAN_POINT('',(88.9265,24.0000000000001,12.2084234471775));
#19808=CARTESIAN_POINT('Ctrl Pts',(88.9237789745047,24.0022328818336,3.70842344717745));
#19809=CARTESIAN_POINT('Ctrl Pts',(88.9225841955761,24.1480569773282,3.70085356786056));
#19810=CARTESIAN_POINT('Ctrl Pts',(88.9980295686384,25.3070877047366,3.6406226334608));
#19811=CARTESIAN_POINT('Ctrl Pts',(90.47008521615,27.2883135148081,3.52773064397815));
#19812=CARTESIAN_POINT('Ctrl Pts',(93.9177921721967,27.0782652002028,3.36974747872952));
#19813=CARTESIAN_POINT('Ctrl Pts',(95.6259966314009,24.0761257688788,3.21176431348088));
#19814=CARTESIAN_POINT('Ctrl Pts',(94.0452974398027,21.0049366707405,3.05378114823225));
#19815=CARTESIAN_POINT('Ctrl Pts',(90.6094455863014,20.6503742748602,2.89579798298361));
#19816=CARTESIAN_POINT('Ctrl Pts',(89.0248750936135,22.6059034459642,2.78067874929868));
#19817=CARTESIAN_POINT('Ctrl Pts',(88.923301212371,23.808501931078,2.71822057069663));
#19818=CARTESIAN_POINT('Ctrl Pts',(88.924991222385,23.997424467889,2.70842344717745));
#19819=CARTESIAN_POINT('Ctrl Pts',(88.9283005269272,23.9974284308675,3.79157655282254));
#19820=CARTESIAN_POINT('Ctrl Pts',(88.9340588461039,24.7122593506074,3.7546088318999));
#19821=CARTESIAN_POINT('Ctrl Pts',(89.5376068210962,26.4541464677684,3.66498005589439));
#19822=CARTESIAN_POINT('Ctrl Pts',(92.4293689246723,27.6012888422859,3.52269022480599));
#19823=CARTESIAN_POINT('Ctrl Pts',(95.2506150476497,25.6084592491483,3.36470705955735));
#19824=CARTESIAN_POINT('Ctrl Pts',(95.1234423470095,22.1567020569745,3.20672389430872));
#19825=CARTESIAN_POINT('Ctrl Pts',(92.1632008787758,20.3768793413443,3.04874072906008));
#19826=CARTESIAN_POINT('Ctrl Pts',(89.4405686580063,21.6964446537072,2.91035828189803));
#19827=CARTESIAN_POINT('Ctrl Pts',(88.9337148573203,23.3617070023829,2.82463688981885));
#19828=CARTESIAN_POINT('Ctrl Pts',(88.9300512599983,24.0019027884479,2.79157655282254));
#19829=CARTESIAN_POINT('Origin',(92.,24.,12.2084234471775));
#19830=CARTESIAN_POINT('',(88.921616510855,24.0005832747793,4.79157655282255));
#19831=CARTESIAN_POINT('',(88.931280553226,24.0004324467725,4.70842344717745));
#19832=CARTESIAN_POINT('',(88.9265,24.0000000000001,12.2084234471775));
#19833=CARTESIAN_POINT('Ctrl Pts',(88.931280553226,24.0004324467725,4.70842344717745));
#19834=CARTESIAN_POINT('Ctrl Pts',(88.9306673998754,24.4838071032452,4.6834865650245));
#19835=CARTESIAN_POINT('Ctrl Pts',(89.2653045337522,25.9871569627812,4.60588862778867));
#19836=CARTESIAN_POINT('Ctrl Pts',(91.608671679144,27.6056215728149,4.47562963546996));
#19837=CARTESIAN_POINT('Ctrl Pts',(94.8057465121273,26.2981364769134,4.31764647022132));
#19838=CARTESIAN_POINT('Ctrl Pts',(95.4579134988245,22.9061631628408,4.15966330497269));
#19839=CARTESIAN_POINT('Ctrl Pts',(92.973634903104,20.506337181354,4.00168013972405));
#19840=CARTESIAN_POINT('Ctrl Pts',(89.7675876228179,21.2385332724819,3.85126685379231));
#19841=CARTESIAN_POINT('Ctrl Pts',(88.9308958629533,23.1336087406012,3.75351462294344));
#19842=CARTESIAN_POINT('Ctrl Pts',(88.9237789745047,24.0022328818336,3.70842344717745));
#19843=CARTESIAN_POINT('Ctrl Pts',(88.921616510855,24.0005832747793,4.79157655282255));
#19844=CARTESIAN_POINT('Ctrl Pts',(88.9215319311911,24.0327646210542,4.78990288414672));
#19845=CARTESIAN_POINT('Ctrl Pts',(88.9365121376522,25.0774335164314,4.73556816038801));
#19846=CARTESIAN_POINT('Ctrl Pts',(90.1148104659794,27.0983381963848,4.62857238154643));
#19847=CARTESIAN_POINT('Ctrl Pts',(93.5645421252575,27.2719790790494,4.4705892162978));
#19848=CARTESIAN_POINT('Ctrl Pts',(95.5951806759186,24.4778232584366,4.31260605104916));
#19849=CARTESIAN_POINT('Ctrl Pts',(94.3648676419543,21.2502654310841,4.15462288580052));
#19850=CARTESIAN_POINT('Ctrl Pts',(90.9895389394379,20.5168107165773,3.99663972055189));
#19851=CARTESIAN_POINT('Ctrl Pts',(89.1060882305935,22.3750682368835,3.8756242762259));
#19852=CARTESIAN_POINT('Ctrl Pts',(88.9258560368481,23.6939723288529,3.80726988698278));
#19853=CARTESIAN_POINT('Ctrl Pts',(88.9283005269272,23.9974284308675,3.79157655282254));
#19854=CARTESIAN_POINT('Origin',(92.,24.,12.2084234471775));
#19855=CARTESIAN_POINT('',(88.9298378032017,24.0020253448727,5.79157655282255));
#19856=CARTESIAN_POINT('',(88.9253101281647,23.9973677263042,5.70842344717746));
#19857=CARTESIAN_POINT('',(88.9265,24.0000000000001,12.2084234471775));
#19858=CARTESIAN_POINT('Ctrl Pts',(88.9253101281647,23.9973677263042,5.70842344717746));
#19859=CARTESIAN_POINT('Ctrl Pts',(88.9326785820548,24.8133509452838,5.66611956218844));
#19860=CARTESIAN_POINT('Ctrl Pts',(89.6842659096931,26.6570905748761,5.57115462211654));
#19861=CARTESIAN_POINT('Ctrl Pts',(92.7888216332755,27.5399724866421,5.42352862696176));
#19862=CARTESIAN_POINT('Ctrl Pts',(95.3956991685213,25.2739199079453,5.26554546171313));
#19863=CARTESIAN_POINT('Ctrl Pts',(94.9225616555133,21.8523784912208,5.1075622964645));
#19864=CARTESIAN_POINT('Ctrl Pts',(91.798560967482,20.3788030856943,4.94957913121586));
#19865=CARTESIAN_POINT('Ctrl Pts',(89.3215406064417,21.9039233849086,4.81653284812018));
#19866=CARTESIAN_POINT('Ctrl Pts',(88.9319622410737,23.4630291545808,4.73614762010738));
#19867=CARTESIAN_POINT('Ctrl Pts',(88.931280553226,24.0004324467725,4.70842344717745));
#19868=CARTESIAN_POINT('Ctrl Pts',(88.9298378032017,24.0020253448727,5.79157655282255));
#19869=CARTESIAN_POINT('Ctrl Pts',(88.9275816449177,24.3706733068195,5.77253588131065));
#19870=CARTESIAN_POINT('Ctrl Pts',(89.15907081827,25.7561579838992,5.70083415471588));
#19871=CARTESIAN_POINT('Ctrl Pts',(91.2111785351691,27.5399717307178,5.57647137303823));
#19872=CARTESIAN_POINT('Ctrl Pts',(94.533543506554,26.5951486388853,5.41848820778961));
#19873=CARTESIAN_POINT('Ctrl Pts',(95.5578980422049,23.2964371536349,5.26050504254096));
#19874=CARTESIAN_POINT('Ctrl Pts',(93.3551176148942,20.6358811841045,5.10252187729233));
#19875=CARTESIAN_POINT('Ctrl Pts',(89.9595568927723,21.0225555274606,4.94621238071953));
#19876=CARTESIAN_POINT('Ctrl Pts',(88.9241931833305,23.0201964387709,4.8425639392296));
#19877=CARTESIAN_POINT('Ctrl Pts',(88.921616510855,24.0005832747793,4.79157655282255));
#19878=CARTESIAN_POINT('Origin',(92.,24.,12.2084234471775));
#19879=CARTESIAN_POINT('',(88.9285848451792,23.9974952079132,6.79157655282255));
#19880=CARTESIAN_POINT('',(88.9234955495304,24.0021186992918,6.70842344717746));
#19881=CARTESIAN_POINT('',(88.9265,24.0000000000001,12.2084234471775));
#19882=CARTESIAN_POINT('Ctrl Pts',(88.9234955495304,24.0021186992919,6.70842344717746));
#19883=CARTESIAN_POINT('Ctrl Pts',(88.9224296149029,24.1371217233644,6.70141361443525));
#19884=CARTESIAN_POINT('Ctrl Pts',(88.9915972274955,25.2852299955925,6.64174272661017));
#19885=CARTESIAN_POINT('Ctrl Pts',(90.4354575406507,27.2719797777491,6.5294107837022));
#19886=CARTESIAN_POINT('Ctrl Pts',(93.8851899365835,27.0983388580017,6.37142761845357));
#19887=CARTESIAN_POINT('Ctrl Pts',(95.624990714543,24.1143988405745,6.21344445320494));
#19888=CARTESIAN_POINT('Ctrl Pts',(94.0768011856692,21.0266951703267,6.0554612879563));
#19889=CARTESIAN_POINT('Ctrl Pts',(90.6448820957342,20.6358804657318,5.89747812270767));
#19890=CARTESIAN_POINT('Ctrl Pts',(89.031950056972,22.5840074378852,5.78179884244805));
#19891=CARTESIAN_POINT('Ctrl Pts',(88.9235061252867,23.7975922920882,5.71878061727132));
#19892=CARTESIAN_POINT('Ctrl Pts',(88.9253101281647,23.9973677263042,5.70842344717746));
#19893=CARTESIAN_POINT('Ctrl Pts',(88.9285848451792,23.9974952079132,6.79157655282255));
#19894=CARTESIAN_POINT('Ctrl Pts',(88.934071073012,24.7016617835355,6.75516887847459));
#19895=CARTESIAN_POINT('Ctrl Pts',(89.523170546697,26.4326506257241,6.66610014904376));
#19896=CARTESIAN_POINT('Ctrl Pts',(92.3913282372869,27.6056208028793,6.52437036453004));
#19897=CARTESIAN_POINT('Ctrl Pts',(95.2334543225921,25.6426844805108,6.36638719928141));
#19898=CARTESIAN_POINT('Ctrl Pts',(95.1427269710462,22.1897772675992,6.20840403403277));
#19899=CARTESIAN_POINT('Ctrl Pts',(92.2014389895034,20.3788038589624,6.05042086878414));
#19900=CARTESIAN_POINT('Ctrl Pts',(89.453954137816,21.6747786389991,5.9114783750474));
#19901=CARTESIAN_POINT('Ctrl Pts',(88.9338215338625,23.3510984132479,5.82519693639353));
#19902=CARTESIAN_POINT('Ctrl Pts',(88.9298378032017,24.0020253448727,5.79157655282255));
#19903=CARTESIAN_POINT('Origin',(92.,24.,12.2084234471775));
#19904=CARTESIAN_POINT('',(88.9215395889802,24.0003901744224,7.79157655282255));
#19905=CARTESIAN_POINT('',(88.9312255436889,24.0006038361494,7.70842344717745));
#19906=CARTESIAN_POINT('',(88.9265,24.0000000000001,12.2084234471775));
#19907=CARTESIAN_POINT('Ctrl Pts',(88.9312255436888,24.0006038361494,7.70842344717745));
#19908=CARTESIAN_POINT('Ctrl Pts',(88.9303877260141,24.473101429326,7.68404661159919));
#19909=CARTESIAN_POINT('Ctrl Pts',(89.2544808710823,25.9652421749014,7.60700872093804));
#19910=CARTESIAN_POINT('Ctrl Pts',(91.5706309836454,27.601289611435,7.47730977519401));
#19911=CARTESIAN_POINT('Ctrl Pts',(94.781330049974,26.327627111039,7.31932660994538));
#19912=CARTESIAN_POINT('Ctrl Pts',(95.4692678342078,22.9427273359205,7.16134344469674));
#19913=CARTESIAN_POINT('Ctrl Pts',(93.0104612763355,20.5168099727604,7.00336027944811));
#19914=CARTESIAN_POINT('Ctrl Pts',(89.7848977769711,21.2177208955611,6.85238694694168));
#19915=CARTESIAN_POINT('Ctrl Pts',(88.9304374011369,23.122917540683,6.75407466951813));
#19916=CARTESIAN_POINT('Ctrl Pts',(88.9234955495304,24.0021186992919,6.70842344717746));
#19917=CARTESIAN_POINT('Ctrl Pts',(88.9215395889802,24.0003901744224,7.79157655282255));
#19918=CARTESIAN_POINT('Ctrl Pts',(88.9215009805821,24.0218014948814,7.79046293072141));
#19919=CARTESIAN_POINT('Ctrl Pts',(88.931364389904,25.0556766305594,7.73668825353739));
#19920=CARTESIAN_POINT('Ctrl Pts',(90.0822082378052,27.0782645420543,7.63025252127047));
#19921=CARTESIAN_POINT('Ctrl Pts',(93.5299144568995,27.2883128130434,7.47226935602186));
#19922=CARTESIAN_POINT('Ctrl Pts',(95.5899362712428,24.5157488852068,7.31428619077321));
#19923=CARTESIAN_POINT('Ctrl Pts',(94.3937632442239,21.2753832325168,7.15630302552458));
#19924=CARTESIAN_POINT('Ctrl Pts',(91.0263653048422,20.5063379273329,6.99831986027594));
#19925=CARTESIAN_POINT('Ctrl Pts',(89.1145962575176,22.3531167219238,6.87674436937527));
#19926=CARTESIAN_POINT('Ctrl Pts',(88.9261356431535,23.6831360059216,6.80782993355747));
#19927=CARTESIAN_POINT('Ctrl Pts',(88.9285848451792,23.9974952079132,6.79157655282255));
#19928=CARTESIAN_POINT('Origin',(92.,24.,12.2084234471775));
#19929=CARTESIAN_POINT('',(88.9296144608475,24.002135757227,8.79157655282255));
#19930=CARTESIAN_POINT('',(88.925632029797,23.9973209161002,8.70842344717745));
#19931=CARTESIAN_POINT('',(88.9265,24.0000000000001,12.2084234471775));
#19932=CARTESIAN_POINT('Ctrl Pts',(88.925632029797,23.9973209161002,8.70842344717745));
#19933=CARTESIAN_POINT('Ctrl Pts',(88.9329422827741,24.802718621963,8.66667960876312));
#19934=CARTESIAN_POINT('Ctrl Pts',(89.6680867896663,26.6359730058285,8.57227471526591));
#19935=CARTESIAN_POINT('Ctrl Pts',(92.7514084417654,27.5481008201034,8.42520876668582));
#19936=CARTESIAN_POINT('Ctrl Pts',(95.382061787488,25.3096961590962,8.26722560143718));
#19937=CARTESIAN_POINT('Ctrl Pts',(94.9450700899456,21.8833496110771,8.10924243618856));
#19938=CARTESIAN_POINT('Ctrl Pts',(91.8367990863051,20.3768785667209,7.95125927093992));
#19939=CARTESIAN_POINT('Ctrl Pts',(89.3333229638364,21.8820745861535,7.81765294126955));
#19940=CARTESIAN_POINT('Ctrl Pts',(88.9321976558787,23.4523691976585,7.73670766668206));
#19941=CARTESIAN_POINT('Ctrl Pts',(88.9312255436888,24.0006038361494,7.70842344717745));
#19942=CARTESIAN_POINT('Ctrl Pts',(88.9296144608475,24.002135757227,8.79157655282255));
#19943=CARTESIAN_POINT('Ctrl Pts',(88.927286249777,24.3598775143588,8.77309592788534));
#19944=CARTESIAN_POINT('Ctrl Pts',(89.1498335279143,25.734213837484,8.70195424786525));
#19945=CARTESIAN_POINT('Ctrl Pts',(91.1738622820844,27.531437528054,8.57815151276229));
#19946=CARTESIAN_POINT('Ctrl Pts',(94.5060022838614,26.6217540231211,8.42016834751365));
#19947=CARTESIAN_POINT('Ctrl Pts',(95.5651291305171,23.3340327163824,8.26218518226502));
#19948=CARTESIAN_POINT('Ctrl Pts',(93.3905541137143,20.6503749960184,8.10420201701639));
#19949=CARTESIAN_POINT('Ctrl Pts',(89.9789222863521,21.0024380002803,7.94733247386889));
#19950=CARTESIAN_POINT('Ctrl Pts',(88.9233266977404,23.0093011817766,7.84312398580429));
#19951=CARTESIAN_POINT('Ctrl Pts',(88.9215395889802,24.0003901744224,7.79157655282255));
#19952=CARTESIAN_POINT('Origin',(92.,24.,12.2084234471775));
#19953=CARTESIAN_POINT('',(88.929711085108,23.9968960951897,9.79157655282255));
#19954=CARTESIAN_POINT('',(88.9232326966468,24.0019373937314,9.70842344717745));
#19955=CARTESIAN_POINT('',(88.9265,24.0000000000001,12.2084234471775));
#19956=CARTESIAN_POINT('',(91.2062007174671,21.0307770462543,10.));
#19957=CARTESIAN_POINT('Ctrl Pts',(91.2062007174671,21.0307770462543,10.));
#19958=CARTESIAN_POINT('Ctrl Pts',(90.2237466982397,21.2934286920664,9.94733894491712));
#19959=CARTESIAN_POINT('Ctrl Pts',(89.1240892170206,22.3312175686104,9.87786446252464));
#19960=CARTESIAN_POINT('Ctrl Pts',(88.9273642764696,23.6716348903192,9.80838998013216));
#19961=CARTESIAN_POINT('Ctrl Pts',(88.929711085108,23.9968960951897,9.79157655282255));
#19962=CARTESIAN_POINT('',(92.7956975117795,21.0256988737941,10.));
#19963=CARTESIAN_POINT('Origin',(92.,24.,10.));
#19964=CARTESIAN_POINT('Ctrl Pts',(92.7957019287907,21.0256870573369,10.));
#19965=CARTESIAN_POINT('Ctrl Pts',(91.8480950072444,20.7745945181247,9.94901908464118));
#19966=CARTESIAN_POINT('Ctrl Pts',(89.7874430689301,21.2303448029462,9.851826900367));
#19967=CARTESIAN_POINT('Ctrl Pts',(88.9299257816843,23.1123258767864,9.75463471609281));
#19968=CARTESIAN_POINT('Ctrl Pts',(88.9232326966468,24.0019373937314,9.70842344717745));
#19969=CARTESIAN_POINT('Origin',(-24.,92.,5.));
#19970=CARTESIAN_POINT('',(-26.5134952662833,92.0002743405047,1.38741669750802));
#19971=CARTESIAN_POINT('',(-26.515626303127,91.9964684456989,1.11258330249198));
#19972=CARTESIAN_POINT('',(-26.5175,92.,5.));
#19973=CARTESIAN_POINT('',(-25.913465996665,93.635987203375,0.999999999999999));
#19974=CARTESIAN_POINT('Ctrl Pts',(-26.515626303127,91.9964684456989,1.11258330249198));
#19975=CARTESIAN_POINT('Ctrl Pts',(-26.5104636015443,92.5890866576526,1.07505553499465));
#19976=CARTESIAN_POINT('Ctrl Pts',(-26.299221828084,93.1848035603044,1.03752776749732));
#19977=CARTESIAN_POINT('Ctrl Pts',(-25.913465996665,93.635987203375,0.999999999999993));
#19978=CARTESIAN_POINT('',(-26.5175,92.,1.));
#19979=CARTESIAN_POINT('Origin',(-24.,92.,1.));
#19980=CARTESIAN_POINT('',(-26.5175,92.,0.));
#19981=CARTESIAN_POINT('',(-26.5175,92.,5.));
#19982=CARTESIAN_POINT('Origin',(-24.,92.,0.));
#19983=CARTESIAN_POINT('',(-22.0828968401885,93.6385343149869,1.));
#19984=CARTESIAN_POINT('Origin',(-24.,92.,1.));
#19985=CARTESIAN_POINT('Ctrl Pts',(-22.0828883826538,93.638540237813,1.));
#19986=CARTESIAN_POINT('Ctrl Pts',(-22.6060431378804,94.2476960524167,1.05098091535882));
#19987=CARTESIAN_POINT('Ctrl Pts',(-23.4465813540296,94.5878274641506,1.10196183071764));
#19988=CARTESIAN_POINT('Ctrl Pts',(-24.2457357689255,94.5094850217743,1.15294274607647));
#19989=CARTESIAN_POINT('Ctrl Pts',(-25.0712273154455,94.4285607063855,1.20560380115935));
#19990=CARTESIAN_POINT('Ctrl Pts',(-25.8525624034826,93.9011253696412,1.25826485624223));
#19991=CARTESIAN_POINT('Ctrl Pts',(-26.2358878554464,93.1658537184213,1.3109259113251));
#19992=CARTESIAN_POINT('Ctrl Pts',(-26.4214827265107,92.8098568843833,1.33642284005274));
#19993=CARTESIAN_POINT('Ctrl Pts',(-26.5137757562956,92.4051388409379,1.36191976878038));
#19994=CARTESIAN_POINT('Ctrl Pts',(-26.5134952662833,92.0002743405047,1.38741669750802));
#19995=CARTESIAN_POINT('Origin',(-24.,92.,5.));
#19996=CARTESIAN_POINT('',(-26.5187354043533,91.9978903847198,2.38741669750802));
#19997=CARTESIAN_POINT('',(-26.521412539848,92.0006455489043,2.11258330249198));
#19998=CARTESIAN_POINT('',(-26.5175,92.,5.));
#19999=CARTESIAN_POINT('Ctrl Pts',(-26.521412539848,92.0006455489043,2.11258330249198));
#20000=CARTESIAN_POINT('Ctrl Pts',(-26.5215322047965,92.0358286169429,2.11034958724147));
#20001=CARTESIAN_POINT('Ctrl Pts',(-26.5208589221676,92.0710069479233,2.10811587199095));
#20002=CARTESIAN_POINT('Ctrl Pts',(-26.5193783713,92.1061512068912,2.10588215674044));
#20003=CARTESIAN_POINT('Ctrl Pts',(-26.4844735772459,92.9346962763346,2.05322110165756));
#20004=CARTESIAN_POINT('Ctrl Pts',(-26.0008839809308,93.7443039053208,2.00056004657468));
#20005=CARTESIAN_POINT('Ctrl Pts',(-25.2879126402955,94.1678868628806,1.9478989914918));
#20006=CARTESIAN_POINT('Ctrl Pts',(-24.5749412996602,94.5914698204405,1.89523793640892));
#20007=CARTESIAN_POINT('Ctrl Pts',(-23.6325882147045,94.629028106574,1.84257688132604));
#20008=CARTESIAN_POINT('Ctrl Pts',(-22.8882532947045,94.2633575703981,1.78991582624317));
#20009=CARTESIAN_POINT('Ctrl Pts',(-22.1439183747044,93.8976870342222,1.73725477116029));
#20010=CARTESIAN_POINT('Ctrl Pts',(-21.59760161966,93.1287876757369,1.68459371607741));
#20011=CARTESIAN_POINT('Ctrl Pts',(-21.4970124750773,92.3057173952046,1.63193266099453));
#20012=CARTESIAN_POINT('Ctrl Pts',(-21.3964233304946,91.4826471146722,1.57927160591165));
#20013=CARTESIAN_POINT('Ctrl Pts',(-21.7415617963736,90.6054059120928,1.52661055082878));
#20014=CARTESIAN_POINT('Ctrl Pts',(-22.3760121357463,90.0711233584702,1.4739494957459));
#20015=CARTESIAN_POINT('Ctrl Pts',(-23.010462475119,89.5368408048476,1.42128844066302));
#20016=CARTESIAN_POINT('Ctrl Pts',(-23.9342246879853,89.3455169001818,1.36862738558014));
#20017=CARTESIAN_POINT('Ctrl Pts',(-24.7281292572936,89.5853895325345,1.31596633049726));
#20018=CARTESIAN_POINT('Ctrl Pts',(-25.5220338266019,89.8252621648871,1.26330527541438));
#20019=CARTESIAN_POINT('Ctrl Pts',(-26.1860807523522,90.4963313342582,1.21064422033151));
#20020=CARTESIAN_POINT('Ctrl Pts',(-26.4192673158648,91.2907310848487,1.15798316524863));
#20021=CARTESIAN_POINT('Ctrl Pts',(-26.4862784936919,91.5190189507993,1.14284987766308));
#20022=CARTESIAN_POINT('Ctrl Pts',(-26.5177081921649,91.7574917511602,1.12771659007753));
#20023=CARTESIAN_POINT('Ctrl Pts',(-26.515626303127,91.9964684456989,1.11258330249198));
#20024=CARTESIAN_POINT('Ctrl Pts',(-26.5134952662833,92.0002743405047,1.38741669750802));
#20025=CARTESIAN_POINT('Ctrl Pts',(-26.5131964355411,91.5689364894248,1.41458082386326));
#20026=CARTESIAN_POINT('Ctrl Pts',(-26.4078218494689,91.1374324020536,1.4417449502185));
#20027=CARTESIAN_POINT('Ctrl Pts',(-26.1982522460689,90.7645021148374,1.46890907657374));
#20028=CARTESIAN_POINT('Ctrl Pts',(-25.7919753688369,90.0415301281689,1.52157013165661));
#20029=CARTESIAN_POINT('Ctrl Pts',(-24.9941057984822,89.5386941205273,1.57423118673949));
#20030=CARTESIAN_POINT('Ctrl Pts',(-24.1666097792392,89.4839131073783,1.62689224182237));
#20031=CARTESIAN_POINT('Ctrl Pts',(-23.3391137599961,89.4291320942294,1.67955329690525));
#20032=CARTESIAN_POINT('Ctrl Pts',(-22.4819912918646,89.8224060755732,1.73221435198813));
#20033=CARTESIAN_POINT('Ctrl Pts',(-21.9839038787409,90.4854401372494,1.78487540707101));
#20034=CARTESIAN_POINT('Ctrl Pts',(-21.4858164656172,91.1484741989255,1.83753646215388));
#20035=CARTESIAN_POINT('Ctrl Pts',(-21.3467641075012,92.081268340934,1.89019751723676));
#20036=CARTESIAN_POINT('Ctrl Pts',(-21.6298379034514,92.8607543617003,1.94285857231964));
#20037=CARTESIAN_POINT('Ctrl Pts',(-21.9129116994015,93.6402403824667,1.99551962740252));
#20038=CARTESIAN_POINT('Ctrl Pts',(-22.6181116494178,94.2664182819908,2.04818068248539));
#20039=CARTESIAN_POINT('Ctrl Pts',(-23.425603594169,94.4553204550754,2.10084173756827));
#20040=CARTESIAN_POINT('Ctrl Pts',(-24.2330955389203,94.6442226281599,2.15350279265115));
#20041=CARTESIAN_POINT('Ctrl Pts',(-25.1428794784065,94.3958490748049,2.20616384773403));
#20042=CARTESIAN_POINT('Ctrl Pts',(-25.7423596992758,93.8228342131325,2.25882490281691));
#20043=CARTESIAN_POINT('Ctrl Pts',(-26.2303119273634,93.3564236982452,2.30168883438061));
#20044=CARTESIAN_POINT('Ctrl Pts',(-26.5126789427165,92.674928901641,2.34455276594432));
#20045=CARTESIAN_POINT('Ctrl Pts',(-26.5187354043533,91.9978903847198,2.38741669750802));
#20046=CARTESIAN_POINT('Origin',(-24.,92.,5.));
#20047=CARTESIAN_POINT('',(-26.5197283545653,92.0018289503525,3.38741669750802));
#20048=CARTESIAN_POINT('',(-26.5145913332516,92.0015585714996,3.11258330249198));
#20049=CARTESIAN_POINT('',(-26.5175,92.,5.));
#20050=CARTESIAN_POINT('Ctrl Pts',(-26.5145913332516,92.0015585714996,3.11258330249198));
#20051=CARTESIAN_POINT('Ctrl Pts',(-26.5163704675347,92.3124536217307,3.0929825844054));
#20052=CARTESIAN_POINT('Ctrl Pts',(-26.4629228052196,92.6227586740843,3.07338186631882));
#20053=CARTESIAN_POINT('Ctrl Pts',(-26.3514581912821,92.9105967308751,3.05378114823224));
#20054=CARTESIAN_POINT('Ctrl Pts',(-26.0519873173872,93.6839283862082,3.00112009314936));
#20055=CARTESIAN_POINT('Ctrl Pts',(-25.3337324697513,94.2950864454347,2.94845903806649));
#20056=CARTESIAN_POINT('Ctrl Pts',(-24.5224342992986,94.4669014516816,2.89579798298361));
#20057=CARTESIAN_POINT('Ctrl Pts',(-23.711136128846,94.6387164579284,2.84313692790073));
#20058=CARTESIAN_POINT('Ctrl Pts',(-22.8067946355765,94.3711884111957,2.79047587281785));
#20059=CARTESIAN_POINT('Ctrl Pts',(-22.2195444883875,93.7856434915613,2.73781481773497));
#20060=CARTESIAN_POINT('Ctrl Pts',(-21.6322943411984,93.2000985719269,2.68515376265209));
#20061=CARTESIAN_POINT('Ctrl Pts',(-21.3621355400899,92.2965367793909,2.63249270756922));
#20062=CARTESIAN_POINT('Ctrl Pts',(-21.5315889600923,91.4847436160309,2.57983165248634));
#20063=CARTESIAN_POINT('Ctrl Pts',(-21.7010423800948,90.6729504526708,2.52717059740346));
#20064=CARTESIAN_POINT('Ctrl Pts',(-22.3101080212084,89.9529259184868,2.47450954232058));
#20065=CARTESIAN_POINT('Ctrl Pts',(-23.0825657562016,89.6512036069521,2.4218484872377));
#20066=CARTESIAN_POINT('Ctrl Pts',(-23.8550234911947,89.3494812954174,2.36918743215482));
#20067=CARTESIAN_POINT('Ctrl Pts',(-24.7908733200675,89.466061206532,2.31652637707195));
#20068=CARTESIAN_POINT('Ctrl Pts',(-25.4656882386074,89.9480924170396,2.26386532198907));
#20069=CARTESIAN_POINT('Ctrl Pts',(-26.1118796445259,90.4096773895362,2.21343798215671));
#20070=CARTESIAN_POINT('Ctrl Pts',(-26.5187110383817,91.2063686024949,2.16301064232434));
#20071=CARTESIAN_POINT('Ctrl Pts',(-26.521412539848,92.0006455489043,2.11258330249198));
#20072=CARTESIAN_POINT('Ctrl Pts',(-26.5187354043533,91.9978903847198,2.38741669750802));
#20073=CARTESIAN_POINT('Ctrl Pts',(-26.5201196894756,91.8431441975284,2.39721382102719));
#20074=CARTESIAN_POINT('Ctrl Pts',(-26.5070691791327,91.6886308117444,2.40701094454637));
#20075=CARTESIAN_POINT('Ctrl Pts',(-26.4787393827788,91.5369716347155,2.41680806806554));
#20076=CARTESIAN_POINT('Ctrl Pts',(-26.3264623431602,90.7217800879606,2.46946912314842));
#20077=CARTESIAN_POINT('Ctrl Pts',(-25.7327317616706,89.9890531644404,2.5221301782313));
#20078=CARTESIAN_POINT('Ctrl Pts',(-24.9668162273558,89.6710932957471,2.57479123331418));
#20079=CARTESIAN_POINT('Ctrl Pts',(-24.2009006930409,89.3531334270537,2.62745228839706));
#20080=CARTESIAN_POINT('Ctrl Pts',(-23.2628002059009,89.4499406131871,2.68011334347994));
#20081=CARTESIAN_POINT('Ctrl Pts',(-22.5779585445906,89.9176119917392,2.73277439856281));
#20082=CARTESIAN_POINT('Ctrl Pts',(-21.8931168832803,90.3852833702914,2.78543545364569));
#20083=CARTESIAN_POINT('Ctrl Pts',(-21.4615340477996,91.2238189412625,2.83809650872857));
#20084=CARTESIAN_POINT('Ctrl Pts',(-21.4789406121676,92.052928097151,2.89075756381144));
#20085=CARTESIAN_POINT('Ctrl Pts',(-21.4963471765355,92.8820372530396,2.94341861889432));
#20086=CARTESIAN_POINT('Ctrl Pts',(-21.9627431407521,93.7017199938457,2.9960796739772));
#20087=CARTESIAN_POINT('Ctrl Pts',(-22.6666097831963,94.1402364113417,3.04874072906008));
#20088=CARTESIAN_POINT('Ctrl Pts',(-23.3704764256404,94.5787528288377,3.10140178414296));
#20089=CARTESIAN_POINT('Ctrl Pts',(-24.3118137463123,94.6361029230236,3.15406283922584));
#20090=CARTESIAN_POINT('Ctrl Pts',(-25.063709299524,94.286277347798,3.20672389430872));
#20091=CARTESIAN_POINT('Ctrl Pts',(-25.8156048527358,93.9364517725723,3.25938494939159));
#20092=CARTESIAN_POINT('Ctrl Pts',(-26.3780586384875,93.1794505279352,3.31204600447447));
#20093=CARTESIAN_POINT('Ctrl Pts',(-26.4959882199517,92.358586646163,3.36470705955735));
#20094=CARTESIAN_POINT('Ctrl Pts',(-26.5129402673076,92.2405897600233,3.37227693887424));
#20095=CARTESIAN_POINT('Ctrl Pts',(-26.5207069963199,92.1212732637326,3.37984681819113));
#20096=CARTESIAN_POINT('Ctrl Pts',(-26.5197283545653,92.0018289503525,3.38741669750802));
#20097=CARTESIAN_POINT('Origin',(-24.,92.,5.));
#20098=CARTESIAN_POINT('',(-26.5135838218621,92.000354216548,4.38741669750802));
#20099=CARTESIAN_POINT('',(-26.5160253566384,91.9978936308049,4.11258330249198));
#20100=CARTESIAN_POINT('',(-26.5175,92.,5.));
#20101=CARTESIAN_POINT('Ctrl Pts',(-26.5160253566384,91.9978936308049,4.11258330249198));
#20102=CARTESIAN_POINT('Ctrl Pts',(-26.5113087243027,92.5834107803607,4.07561558156934));
#20103=CARTESIAN_POINT('Ctrl Pts',(-26.3074058729855,93.1718905111793,4.03864786064669));
#20104=CARTESIAN_POINT('Ctrl Pts',(-25.9337852402154,93.6183375776454,4.00168013972405));
#20105=CARTESIAN_POINT('Ctrl Pts',(-25.4015572253053,94.2543079045141,3.94901908464117));
#20106=CARTESIAN_POINT('Ctrl Pts',(-24.5249308268757,94.6020596393698,3.8963580295583));
#20107=CARTESIAN_POINT('Ctrl Pts',(-23.7014710746985,94.5038814515943,3.84369697447542));
#20108=CARTESIAN_POINT('Ctrl Pts',(-22.8780113225213,94.4057032638187,3.79103591939254));
#20109=CARTESIAN_POINT('Ctrl Pts',(-22.1077182165964,93.8615951534119,3.73837486430966));
#20110=CARTESIAN_POINT('Ctrl Pts',(-21.7399328314132,93.1183194017708,3.68571380922678));
#20111=CARTESIAN_POINT('Ctrl Pts',(-21.3721474462299,92.3750436501297,3.6330527541439));
#20112=CARTESIAN_POINT('Ctrl Pts',(-21.4068697817883,91.4326002572543,3.58039169906102));
#20113=CARTESIAN_POINT('Ctrl Pts',(-21.8283526559748,90.7184034519114,3.52773064397815));
#20114=CARTESIAN_POINT('Ctrl Pts',(-22.2498355301614,90.0042066465684,3.47506958889527));
#20115=CARTESIAN_POINT('Ctrl Pts',(-23.058078942976,89.5182564287579,3.42240853381239));
#20116=CARTESIAN_POINT('Ctrl Pts',(-23.8865307343324,89.4809393801385,3.36974747872951));
#20117=CARTESIAN_POINT('Ctrl Pts',(-24.7149825256888,89.4436223315191,3.31708642364663));
#20118=CARTESIAN_POINT('Ctrl Pts',(-25.5636426955868,89.8549384520908,3.26442536856376));
#20119=CARTESIAN_POINT('Ctrl Pts',(-26.0476293304589,90.5283491380965,3.21176431348088));
#20120=CARTESIAN_POINT('Ctrl Pts',(-26.3514736272622,90.951112870825,3.17870397648458));
#20121=CARTESIAN_POINT('Ctrl Pts',(-26.5115904850836,91.4771749705661,3.14564363948828));
#20122=CARTESIAN_POINT('Ctrl Pts',(-26.5145913332516,92.0015585714996,3.11258330249198));
#20123=CARTESIAN_POINT('Ctrl Pts',(-26.5197283545653,92.0018289503525,3.38741669750802));
#20124=CARTESIAN_POINT('Ctrl Pts',(-26.5138989211591,91.2903401268976,3.43250787327401));
#20125=CARTESIAN_POINT('Ctrl Pts',(-26.1977683024704,90.5743161275881,3.47759904904));
#20126=CARTESIAN_POINT('Ctrl Pts',(-25.6643206092001,90.105645640677,3.52269022480598));
#20127=CARTESIAN_POINT('Ctrl Pts',(-25.0413180398075,89.5582950358707,3.57535127988886));
#20128=CARTESIAN_POINT('Ctrl Pts',(-24.1219075238456,89.3483203451655,3.62801233497174));
#20129=CARTESIAN_POINT('Ctrl Pts',(-23.3230574099716,89.5709486859401,3.68067339005462));
#20130=CARTESIAN_POINT('Ctrl Pts',(-22.5242072960976,89.7935770267148,3.7333344451375));
#20131=CARTESIAN_POINT('Ctrl Pts',(-21.8459175843117,90.4488083989693,3.78599550022037));
#20132=CARTESIAN_POINT('Ctrl Pts',(-21.5958042400641,91.239484187431,3.83865655530325));
#20133=CARTESIAN_POINT('Ctrl Pts',(-21.3456908958166,92.0301599758926,3.89131761038613));
#20134=CARTESIAN_POINT('Ctrl Pts',(-21.5237539191076,92.9562801805612,3.94397866546901));
#20135=CARTESIAN_POINT('Ctrl Pts',(-22.0492386873867,93.5978334861916,3.99663972055189));
#20136=CARTESIAN_POINT('Ctrl Pts',(-22.5747234556659,94.2393867918219,4.04930077563476));
#20137=CARTESIAN_POINT('Ctrl Pts',(-23.4476299689333,94.5963731984139,4.10196183071764));
#20138=CARTESIAN_POINT('Ctrl Pts',(-24.2720802276353,94.5068932768484,4.15462288580052));
#20139=CARTESIAN_POINT('Ctrl Pts',(-25.0965304863373,94.417413355283,4.2072839408834));
#20140=CARTESIAN_POINT('Ctrl Pts',(-25.8725244904738,93.8814671055602,4.25994499596628));
#20141=CARTESIAN_POINT('Ctrl Pts',(-26.2481357153638,93.1421152990992,4.31260605104916));
#20142=CARTESIAN_POINT('Ctrl Pts',(-26.4260009866856,92.7920059281747,4.33754293320211));
#20143=CARTESIAN_POINT('Ctrl Pts',(-26.5140860549172,92.396285723967,4.36247981535506));
#20144=CARTESIAN_POINT('Ctrl Pts',(-26.5135838218621,92.000354216548,4.38741669750802));
#20145=CARTESIAN_POINT('Origin',(-24.,92.,5.));
#20146=CARTESIAN_POINT('',(-26.5184741887082,91.9978439082844,5.38741669750802));
#20147=CARTESIAN_POINT('',(-26.5215002261917,92.0004777596725,5.11258330249198));
#20148=CARTESIAN_POINT('',(-26.5175,92.,5.));
#20149=CARTESIAN_POINT('Ctrl Pts',(-26.5215002261917,92.0004777596725,5.11258330249198));
#20150=CARTESIAN_POINT('Ctrl Pts',(-26.5215695052931,92.0268374618337,5.11090963381615));
#20151=CARTESIAN_POINT('Ctrl Pts',(-26.5211915450549,92.0531951295678,5.10923596514032));
#20152=CARTESIAN_POINT('Ctrl Pts',(-26.5203601912646,92.0795384889352,5.10756229646449));
#20153=CARTESIAN_POINT('Ctrl Pts',(-26.494202106107,92.9084176564484,5.05490124138161));
#20154=CARTESIAN_POINT('Ctrl Pts',(-26.0191792969125,93.723131379711,5.00224018629873));
#20155=CARTESIAN_POINT('Ctrl Pts',(-25.3107227144406,94.1541930811531,4.94957913121586));
#20156=CARTESIAN_POINT('Ctrl Pts',(-24.6022661319687,94.5852547825952,4.89691807613298));
#20157=CARTESIAN_POINT('Ctrl Pts',(-23.6603757762194,94.6326644622167,4.8442570210501));
#20158=CARTESIAN_POINT('Ctrl Pts',(-22.9122149978594,94.2749210214316,4.79159596596722));
#20159=CARTESIAN_POINT('Ctrl Pts',(-22.1640542194994,93.9171775806464,4.73893491088435));
#20160=CARTESIAN_POINT('Ctrl Pts',(-21.6096230185287,93.1542810194546,4.68627385580146));
#20161=CARTESIAN_POINT('Ctrl Pts',(-21.50036540662,92.3322179475565,4.63361280071859));
#20162=CARTESIAN_POINT('Ctrl Pts',(-21.3911077947114,91.5101548756584,4.58095174563571));
#20163=CARTESIAN_POINT('Ctrl Pts',(-21.7270237718648,90.6289252930541,4.52829069055283));
#20164=CARTESIAN_POINT('Ctrl Pts',(-22.3557697095322,90.0881818554959,4.47562963546995));
#20165=CARTESIAN_POINT('Ctrl Pts',(-22.9845156471996,89.5474384179376,4.42296858038708));
#20166=CARTESIAN_POINT('Ctrl Pts',(-23.906091545381,89.3471811254255,4.3703075253042));
#20167=CARTESIAN_POINT('Ctrl Pts',(-24.7025470068623,89.5782300758527,4.31764647022132));
#20168=CARTESIAN_POINT('Ctrl Pts',(-25.4990024683437,89.80927902628,4.26498541513844));
#20169=CARTESIAN_POINT('Ctrl Pts',(-26.1703374931251,90.4716342196466,4.21232436005556));
#20170=CARTESIAN_POINT('Ctrl Pts',(-26.4120901898205,91.2649062757708,4.15966330497269));
#20171=CARTESIAN_POINT('Ctrl Pts',(-26.4841340531159,91.5013064663318,4.14396997081245));
#20172=CARTESIAN_POINT('Ctrl Pts',(-26.5180276355322,91.7493331013702,4.12827663665222));
#20173=CARTESIAN_POINT('Ctrl Pts',(-26.5160253566384,91.9978936308049,4.11258330249198));
#20174=CARTESIAN_POINT('Ctrl Pts',(-26.5135838218621,92.000354216548,4.38741669750802));
#20175=CARTESIAN_POINT('Ctrl Pts',(-26.5130254522959,91.5601679289134,4.41514087043794));
#20176=CARTESIAN_POINT('Ctrl Pts',(-26.4029695423041,91.1197204618368,4.44286504336787));
#20177=CARTESIAN_POINT('Ctrl Pts',(-26.1850553752594,90.7413997625482,4.47058921629779));
#20178=CARTESIAN_POINT('Ctrl Pts',(-25.7711353646214,90.0227933956572,4.52325027138067));
#20179=CARTESIAN_POINT('Ctrl Pts',(-24.9680668977021,89.5283380250743,4.57591132646355));
#20180=CARTESIAN_POINT('Ctrl Pts',(-24.1400552293209,89.4822775999311,4.62857238154643));
#20181=CARTESIAN_POINT('Ctrl Pts',(-23.3120435609398,89.4362171747879,4.68123343662931));
#20182=CARTESIAN_POINT('Ctrl Pts',(-22.4590886910969,89.8385516950844,4.73389449171218));
#20183=CARTESIAN_POINT('Ctrl Pts',(-21.9680202099297,90.506815589517,4.78655554679506));
#20184=CARTESIAN_POINT('Ctrl Pts',(-21.4769517287624,91.1750794839497,4.83921660187794));
#20185=CARTESIAN_POINT('Ctrl Pts',(-21.3477696362708,92.1092727525185,4.89187765696082));
#20186=CARTESIAN_POINT('Ctrl Pts',(-21.6390602159943,92.8857228049574,4.94453871204369));
#20187=CARTESIAN_POINT('Ctrl Pts',(-21.9303507957177,93.6621728573964,4.99719976712657));
#20188=CARTESIAN_POINT('Ctrl Pts',(-22.6421140476561,94.2808796937054,5.04986082220945));
#20189=CARTESIAN_POINT('Ctrl Pts',(-23.4515531900704,94.4612492047027,5.10252187729233));
#20190=CARTESIAN_POINT('Ctrl Pts',(-24.2609923324847,94.6416187157001,5.15518293237521));
#20191=CARTESIAN_POINT('Ctrl Pts',(-25.1681073653747,94.3836509013857,5.20784398745809));
#20192=CARTESIAN_POINT('Ctrl Pts',(-25.7615061404264,93.8043385680607,5.26050504254096));
#20193=CARTESIAN_POINT('Ctrl Pts',(-26.2381975681409,93.3389631158763,5.30280892752999));
#20194=CARTESIAN_POINT('Ctrl Pts',(-26.5124386983965,92.6662146256838,5.345112812519));
#20195=CARTESIAN_POINT('Ctrl Pts',(-26.5184741887082,91.9978439082844,5.38741669750802));
#20196=CARTESIAN_POINT('Origin',(-24.,92.,5.));
#20197=CARTESIAN_POINT('',(-26.5199605075385,92.0017354236374,6.38741669750802));
#20198=CARTESIAN_POINT('',(-26.5147661754846,92.0016589575576,6.11258330249198));
#20199=CARTESIAN_POINT('',(-26.5175,92.,5.));
#20200=CARTESIAN_POINT('Ctrl Pts',(-26.5147661754846,92.0016589575576,6.11258330249198));
#20201=CARTESIAN_POINT('Ctrl Pts',(-26.5166141920308,92.3036180613248,6.09354263098009));
#20202=CARTESIAN_POINT('Ctrl Pts',(-26.4662618562805,92.604981570585,6.07450195946819));
#20203=CARTESIAN_POINT('Ctrl Pts',(-26.3609398422945,92.8857228268249,6.0554612879563));
#20204=CARTESIAN_POINT('Ctrl Pts',(-26.0696492553794,93.6621728984334,6.00280023287342));
#20205=CARTESIAN_POINT('Ctrl Pts',(-25.3578859858684,94.2808797500175,5.95013917779054));
#20206=CARTESIAN_POINT('Ctrl Pts',(-24.54844682347,94.4612492654679,5.89747812270766));
#20207=CARTESIAN_POINT('Ctrl Pts',(-23.7390076610717,94.6416187809184,5.84481706762479));
#20208=CARTESIAN_POINT('Ctrl Pts',(-22.831892605786,94.3836509602352,5.79215601254191));
#20209=CARTESIAN_POINT('Ctrl Pts',(-22.2384938160841,93.8043386126077,5.73949495745903));
#20210=CARTESIAN_POINT('Ctrl Pts',(-21.6450950263821,93.2250262649801,5.68683390237615));
#20211=CARTESIAN_POINT('Ctrl Pts',(-21.3654125022639,92.3243693904083,5.63417284729328));
#20212=CARTESIAN_POINT('Ctrl Pts',(-21.5262870414957,91.5108312521748,5.58151179221039));
#20213=CARTESIAN_POINT('Ctrl Pts',(-21.6871615807276,90.6972931139413,5.52885073712751));
#20214=CARTESIAN_POINT('Ctrl Pts',(-22.2885931833095,89.9708737120461,5.47618968204464));
#20215=CARTESIAN_POINT('Ctrl Pts',(-23.0578223533957,89.6610166423891,5.42352862696176));
#20216=CARTESIAN_POINT('Ctrl Pts',(-23.827051523482,89.3511595727321,5.37086757187888));
#20217=CARTESIAN_POINT('Ctrl Pts',(-24.7640782610726,89.4578648353135,5.318206516796));
#20218=CARTESIAN_POINT('Ctrl Pts',(-25.4439449493076,89.9327397724859,5.26554546171313));
#20219=CARTESIAN_POINT('Ctrl Pts',(-26.102204178709,90.392522279284,5.21455807530608));
#20220=CARTESIAN_POINT('Ctrl Pts',(-26.5193896768554,91.1974440773951,5.16357068889903));
#20221=CARTESIAN_POINT('Ctrl Pts',(-26.5215002261917,92.0004777596725,5.11258330249198));
#20222=CARTESIAN_POINT('Ctrl Pts',(-26.5184741887082,91.9978439082844,5.38741669750802));
#20223=CARTESIAN_POINT('Ctrl Pts',(-26.5199518449512,91.8342081285527,5.39777386760188));
#20224=CARTESIAN_POINT('Ctrl Pts',(-26.5053530710441,91.670834755527,5.40813103769574));
#20225=CARTESIAN_POINT('Ctrl Pts',(-26.4737128974313,91.5108312642518,5.4184882077896));
#20226=CARTESIAN_POINT('Ctrl Pts',(-26.3128383621713,90.6972931461036,5.47114926287248));
#20227=CARTESIAN_POINT('Ctrl Pts',(-25.711406774438,89.9708737621428,5.52381031795536));
#20228=CARTESIAN_POINT('Ctrl Pts',(-24.9421776233431,89.6610167001358,5.57647137303823));
#20229=CARTESIAN_POINT('Ctrl Pts',(-24.1729484722482,89.3511596381288,5.62913242812111));
#20230=CARTESIAN_POINT('Ctrl Pts',(-23.2359217577917,89.4578648980757,5.68179348320399));
#20231=CARTESIAN_POINT('Ctrl Pts',(-22.5560550863417,89.9327398235241,5.73445453828687));
#20232=CARTESIAN_POINT('Ctrl Pts',(-21.8761884148918,90.4076147489724,5.78711559336975));
#20233=CARTESIAN_POINT('Ctrl Pts',(-21.4534817864484,91.2506593399223,5.83977664845262));
#20234=CARTESIAN_POINT('Ctrl Pts',(-21.4796398709601,92.0795384869714,5.8924377035355));
#20235=CARTESIAN_POINT('Ctrl Pts',(-21.5057979554718,92.9084176340206,5.94509875861838));
#20236=CARTESIAN_POINT('Ctrl Pts',(-21.9808207529386,93.723131337169,5.99775981370126));
#20237=CARTESIAN_POINT('Ctrl Pts',(-22.6892773179196,94.1541930279687,6.05042086878414));
#20238=CARTESIAN_POINT('Ctrl Pts',(-23.3977338829005,94.5852547187683,6.10308192386702));
#20239=CARTESIAN_POINT('Ctrl Pts',(-24.3396242153956,94.6326643972192,6.15574297894989));
#20240=CARTESIAN_POINT('Ctrl Pts',(-25.0877849752844,94.2749209652664,6.20840403403277));
#20241=CARTESIAN_POINT('Ctrl Pts',(-25.8359457351732,93.9171775333136,6.26106508911565));
#20242=CARTESIAN_POINT('Ctrl Pts',(-26.3903769224557,93.154280990957,6.31372614419853));
#20243=CARTESIAN_POINT('Ctrl Pts',(-26.499634531667,92.3322179393546,6.36638719928141));
#20244=CARTESIAN_POINT('Ctrl Pts',(-26.5141780603748,92.2227912579824,6.37339703202361));
#20245=CARTESIAN_POINT('Ctrl Pts',(-26.5208336131063,92.1123162124966,6.38040686476582));
#20246=CARTESIAN_POINT('Ctrl Pts',(-26.5199605075385,92.0017354236374,6.38741669750802));
#20247=CARTESIAN_POINT('Origin',(-24.,92.,5.));
#20248=CARTESIAN_POINT('',(-26.5136288801011,92.0004946012931,7.38741669750802));
#20249=CARTESIAN_POINT('',(-26.5157924718976,91.9979483278017,7.11258330249198));
#20250=CARTESIAN_POINT('',(-26.5175,92.,5.));
#20251=CARTESIAN_POINT('Ctrl Pts',(-26.5157924718976,91.9979483278017,7.11258330249198));
#20252=CARTESIAN_POINT('Ctrl Pts',(-26.511298709256,92.5747303258767,7.07617562814402));
#20253=CARTESIAN_POINT('Ctrl Pts',(-26.3140597937548,93.1542901069194,7.03976795379606));
#20254=CARTESIAN_POINT('Ctrl Pts',(-25.9507613607754,93.5978335256406,7.0033602794481));
#20255=CARTESIAN_POINT('Ctrl Pts',(-25.4252765795229,94.2393868471104,6.95069922436522));
#20256=CARTESIAN_POINT('Ctrl Pts',(-24.552370044704,94.5963732625152,6.89803816928235));
#20257=CARTESIAN_POINT('Ctrl Pts',(-23.7279197656472,94.5068933387405,6.84537711419947));
#20258=CARTESIAN_POINT('Ctrl Pts',(-22.9034694865904,94.4174134149657,6.79271605911659));
#20259=CARTESIAN_POINT('Ctrl Pts',(-22.1274754632958,93.8814671520113,6.74005500403371));
#20260=CARTESIAN_POINT('Ctrl Pts',(-21.7518642291324,93.1421153272968,6.68739394895083));
#20261=CARTESIAN_POINT('Ctrl Pts',(-21.3762529949691,92.4027635025822,6.63473289386796));
#20262=CARTESIAN_POINT('Ctrl Pts',(-21.4010245499371,91.4600061161074,6.58207183878508));
#20263=CARTESIAN_POINT('Ctrl Pts',(-21.8149445707942,90.7413997314748,6.5294107837022));
#20264=CARTESIAN_POINT('Ctrl Pts',(-22.2288645916513,90.0227933468422,6.47674972861932));
#20265=CARTESIAN_POINT('Ctrl Pts',(-23.0319330783976,89.5283379640518,6.42408867353645));
#20266=CARTESIAN_POINT('Ctrl Pts',(-23.8599447672214,89.4822775377715,6.37142761845357));
#20267=CARTESIAN_POINT('Ctrl Pts',(-24.6879564560451,89.4362171114911,6.31876656337069));
#20268=CARTESIAN_POINT('Ctrl Pts',(-25.5409113469464,89.8385516417208,6.26610550828781));
#20269=CARTESIAN_POINT('Ctrl Pts',(-26.0319798402375,90.5068155526521,6.21344445320493));
#20270=CARTESIAN_POINT('Ctrl Pts',(-26.3454925694847,90.9334551058627,6.17982406963395));
#20271=CARTESIAN_POINT('Ctrl Pts',(-26.5115031064752,91.4684854880682,6.14620368606297));
#20272=CARTESIAN_POINT('Ctrl Pts',(-26.5147661754846,92.0016589575576,6.11258330249198));
#20273=CARTESIAN_POINT('Ctrl Pts',(-26.5199605075385,92.0017354236374,6.38741669750802));
#20274=CARTESIAN_POINT('Ctrl Pts',(-26.5142744465628,91.2815829799959,6.43306791984869));
#20275=CARTESIAN_POINT('Ctrl Pts',(-26.1892823731636,90.556945740582,6.47871914218937));
#20276=CARTESIAN_POINT('Ctrl Pts',(-25.6442302498738,90.0881819026962,6.52437036453004));
#20277=CARTESIAN_POINT('Ctrl Pts',(-25.0154843277294,89.5474384784885,6.57703141961292));
#20278=CARTESIAN_POINT('Ctrl Pts',(-24.0939084523006,89.3471811909213,6.6296924746958));
#20279=CARTESIAN_POINT('Ctrl Pts',(-23.2974530104828,89.5782301356438,6.68235352977867));
#20280=CARTESIAN_POINT('Ctrl Pts',(-22.5009975686649,89.8092790803663,6.73501458486155));
#20281=CARTESIAN_POINT('Ctrl Pts',(-21.829662560458,90.4716342573785,6.78767563994443));
#20282=CARTESIAN_POINT('Ctrl Pts',(-21.5879098697311,91.2649062939185,6.84033669502731));
#20283=CARTESIAN_POINT('Ctrl Pts',(-21.3461571790042,92.0581783304585,6.89299775011019));
#20284=CARTESIAN_POINT('Ctrl Pts',(-21.5339868057573,92.9823672265264,6.94565880519306));
#20285=CARTESIAN_POINT('Ctrl Pts',(-22.0662148075274,93.6183375376923,6.99831986027594));
#20286=CARTESIAN_POINT('Ctrl Pts',(-22.5984428092974,94.2543078488581,7.05098091535882));
#20287=CARTESIAN_POINT('Ctrl Pts',(-23.4750691860844,94.602059575122,7.1036419704417));
#20288=CARTESIAN_POINT('Ctrl Pts',(-24.2985289179312,94.5038813897733,7.15630302552458));
#20289=CARTESIAN_POINT('Ctrl Pts',(-25.121988649778,94.4057032044246,7.20896408060746));
#20290=CARTESIAN_POINT('Ctrl Pts',(-25.8922817366847,93.8615951074632,7.26162513569033));
#20291=CARTESIAN_POINT('Ctrl Pts',(-26.2600671127882,93.1183193741671,7.31428619077321));
#20292=CARTESIAN_POINT('Ctrl Pts',(-26.4303151951188,92.7742565689049,7.33866302635148));
#20293=CARTESIAN_POINT('Ctrl Pts',(-26.5143151353889,92.3875167213616,7.36303986192975));
#20294=CARTESIAN_POINT('Ctrl Pts',(-26.5136288801011,92.0004946012931,7.38741669750802));
#20295=CARTESIAN_POINT('Origin',(-24.,92.,5.));
#20296=CARTESIAN_POINT('',(-26.5182105203766,91.9978055611691,8.38741669750802));
#20297=CARTESIAN_POINT('',(-26.5215632327497,92.0003195913041,8.11258330249199));
#20298=CARTESIAN_POINT('',(-26.5175,92.,5.));
#20299=CARTESIAN_POINT('Ctrl Pts',(-26.5215632327497,92.0003195913041,8.11258330249199));
#20300=CARTESIAN_POINT('Ctrl Pts',(-26.5215948568411,92.0178575782261,8.11146968039084));
#20301=CARTESIAN_POINT('Ctrl Pts',(-26.521427546271,92.0353949460436,8.1103560582897));
#20302=CARTESIAN_POINT('Ctrl Pts',(-26.5210594500516,92.052928098419,8.10924243618855));
#20303=CARTESIAN_POINT('Ctrl Pts',(-26.5036528852352,92.8820372747418,8.05658138110567));
#20304=CARTESIAN_POINT('Ctrl Pts',(-26.0372569095473,93.7017200358608,8.00392032602279));
#20305=CARTESIAN_POINT('Ctrl Pts',(-25.3333902497356,94.1402364642016,7.95125927093991));
#20306=CARTESIAN_POINT('Ctrl Pts',(-24.6295235899239,94.5787528925424,7.89859821585703));
#20307=CARTESIAN_POINT('Ctrl Pts',(-23.6881862459885,94.636102988105,7.84593716077416));
#20308=CARTESIAN_POINT('Ctrl Pts',(-22.9362906742079,94.2862774042331,7.79327610569128));
#20309=CARTESIAN_POINT('Ctrl Pts',(-22.1843951024273,93.9364518203612,7.7406150506084));
#20310=CARTESIAN_POINT('Ctrl Pts',(-21.6219413028015,93.1794505570548,7.68795399552552));
#20311=CARTESIAN_POINT('Ctrl Pts',(-21.5040117184286,92.3585866550213,7.63529294044264));
#20312=CARTESIAN_POINT('Ctrl Pts',(-21.3860821340558,91.5377227529878,7.58263188535977));
#20313=CARTESIAN_POINT('Ctrl Pts',(-21.7126767649359,90.6529962122272,7.52997083027689));
#20314=CARTESIAN_POINT('Ctrl Pts',(-22.3356793497081,90.105645593905,7.47730977519401));
#20315=CARTESIAN_POINT('Ctrl Pts',(-22.9586819344804,89.5582949755827,7.42464872011113));
#20316=CARTESIAN_POINT('Ctrl Pts',(-23.8780924731448,89.3483202796988,7.37198766502825));
#20317=CARTESIAN_POINT('Ctrl Pts',(-24.6769426067422,89.5709486259712,7.31932660994537));
#20318=CARTESIAN_POINT('Ctrl Pts',(-25.4757927403397,89.7935769722436,7.2666655548625));
#20319=CARTESIAN_POINT('Ctrl Pts',(-26.1540824688701,90.4488083606723,7.21400449977962));
#20320=CARTESIAN_POINT('Ctrl Pts',(-26.4041958192921,91.2394841686541,7.16134344469674));
#20321=CARTESIAN_POINT('Ctrl Pts',(-26.4813911490268,91.4835194414908,7.14509006396182));
#20322=CARTESIAN_POINT('Ctrl Pts',(-26.517798610341,91.7404570822428,7.1288366832269));
#20323=CARTESIAN_POINT('Ctrl Pts',(-26.5157924718976,91.9979483278017,7.11258330249198));
#20324=CARTESIAN_POINT('Ctrl Pts',(-26.5136288801011,92.0004946012931,7.38741669750802));
#20325=CARTESIAN_POINT('Ctrl Pts',(-26.5128326243634,91.5514363729595,7.41570091701263));
#20326=CARTESIAN_POINT('Ctrl Pts',(-26.3980254709817,91.1019981282164,7.44398513651724));
#20327=CARTESIAN_POINT('Ctrl Pts',(-26.1716472904104,90.7184034835404,7.47226935602185));
#20328=CARTESIAN_POINT('Ctrl Pts',(-25.7501644266289,90.0042066958411,7.52493041110473));
#20329=CARTESIAN_POINT('Ctrl Pts',(-24.9419210337657,89.5182564900734,7.5775914661876));
#20330=CARTESIAN_POINT('Ctrl Pts',(-24.1134692628649,89.4809394423544,7.63025252127048));
#20331=CARTESIAN_POINT('Ctrl Pts',(-23.285017491964,89.4436223946354,7.68291357635336));
#20332=CARTESIAN_POINT('Ctrl Pts',(-22.4363573430257,89.8549385049651,7.73557463143624));
#20333=CARTESIAN_POINT('Ctrl Pts',(-21.9523707200979,90.5283491743849,7.78823568651912));
#20334=CARTESIAN_POINT('Ctrl Pts',(-21.4683840971702,91.2017598438046,7.840896741602));
#20335=CARTESIAN_POINT('Ctrl Pts',(-21.3490710002532,92.1372650723145,7.89355779668487));
#20336=CARTESIAN_POINT('Ctrl Pts',(-21.648541866765,92.9105967084797,7.94621885176775));
#20337=CARTESIAN_POINT('Ctrl Pts',(-21.9480127332768,93.6839283446448,7.99887990685063));
#20338=CARTESIAN_POINT('Ctrl Pts',(-22.6662675632174,94.2950863884653,8.05154096193351));
#20339=CARTESIAN_POINT('Ctrl Pts',(-23.4775657136168,94.4669013906121,8.10420201701639));
#20340=CARTESIAN_POINT('Ctrl Pts',(-24.2888638640162,94.6387163927589,8.15686307209926));
#20341=CARTESIAN_POINT('Ctrl Pts',(-25.1932053348746,94.3711883532321,8.20952412718214));
#20342=CARTESIAN_POINT('Ctrl Pts',(-25.7804554676164,93.785643447789,8.26218518226502));
#20343=CARTESIAN_POINT('Ctrl Pts',(-26.2459621805258,93.3214884497798,8.30392902067936));
#20344=CARTESIAN_POINT('Ctrl Pts',(-26.5122227023915,92.6575056999379,8.34567285909369));
#20345=CARTESIAN_POINT('Ctrl Pts',(-26.5182105203766,91.9978055611691,8.38741669750802));
#20346=CARTESIAN_POINT('Origin',(-24.,92.,5.));
#20347=CARTESIAN_POINT('',(-26.5201758362126,92.0015868137837,9.38741669750802));
#20348=CARTESIAN_POINT('',(-26.5149491154365,92.0017493991467,9.11258330249198));
#20349=CARTESIAN_POINT('',(-26.5175,92.,5.));
#20350=CARTESIAN_POINT('',(-22.0865340033349,93.6359872033749,10.));
#20351=CARTESIAN_POINT('Ctrl Pts',(-26.5201758362126,92.0015868137837,9.38741669750802));
#20352=CARTESIAN_POINT('Ctrl Pts',(-26.5146934294681,91.2729074143925,9.43362796642338));
#20353=CARTESIAN_POINT('Ctrl Pts',(-26.1807323142246,90.5399684977903,9.47983923533873));
#20354=CARTESIAN_POINT('Ctrl Pts',(-25.6239878020485,90.0711234457756,9.52605050425409));
#20355=CARTESIAN_POINT('Ctrl Pts',(-24.9895375021336,89.5368408846388,9.57871155933697));
#20356=CARTESIAN_POINT('Ctrl Pts',(-24.0657754031769,89.3455168748646,9.63137261441985));
#20357=CARTESIAN_POINT('Ctrl Pts',(-23.2718707713924,89.5853895680493,9.68403366950273));
#20358=CARTESIAN_POINT('Ctrl Pts',(-22.4779661396078,89.825262261234,9.73669472458561));
#20359=CARTESIAN_POINT('Ctrl Pts',(-21.8139189749953,90.4963316573775,9.78935577966849));
#20360=CARTESIAN_POINT('Ctrl Pts',(-21.5807324199303,91.2907313838813,9.84201683475137));
#20361=CARTESIAN_POINT('Ctrl Pts',(-21.3475458648653,92.0851311103851,9.89467788983424));
#20362=CARTESIAN_POINT('Ctrl Pts',(-21.5452199193478,93.0028611672492,9.94733894491712));
#20363=CARTESIAN_POINT('Ctrl Pts',(-22.0865340033349,93.6359872033749,10.));
#20364=CARTESIAN_POINT('',(-25.9171032040961,93.6385343199285,10.));
#20365=CARTESIAN_POINT('Origin',(-24.,92.,10.));
#20366=CARTESIAN_POINT('Ctrl Pts',(-25.9171116625783,93.6385402433575,10.));
#20367=CARTESIAN_POINT('Ctrl Pts',(-25.393956920721,94.2476959894344,9.94901908464118));
#20368=CARTESIAN_POINT('Ctrl Pts',(-24.5534186715195,94.5878275437024,9.89803816928236));
#20369=CARTESIAN_POINT('Ctrl Pts',(-23.7542642292644,94.5094851289583,9.84705725392353));
#20370=CARTESIAN_POINT('Ctrl Pts',(-22.9287726544835,94.4285608421125,9.79439619884065));
#20371=CARTESIAN_POINT('Ctrl Pts',(-22.1474375442602,93.9011254113112,9.74173514375777));
#20372=CARTESIAN_POINT('Ctrl Pts',(-21.7641120845165,93.1658537236911,9.68907408867489));
#20373=CARTESIAN_POINT('Ctrl Pts',(-21.3807866247728,92.4305820360709,9.63641303359201));
#20374=CARTESIAN_POINT('Ctrl Pts',(-21.3954708155088,91.487474091632,9.58375197850913));
#20375=CARTESIAN_POINT('Ctrl Pts',(-21.8017477031856,90.764502097224,9.53109092342626));
#20376=CARTESIAN_POINT('Ctrl Pts',(-22.2080245908624,90.041530102816,9.47842986834338));
#20377=CARTESIAN_POINT('Ctrl Pts',(-23.0058941754799,89.5386940584389,9.4257688132605));
#20378=CARTESIAN_POINT('Ctrl Pts',(-23.8333902143466,89.4839130383455,9.37310775817762));
#20379=CARTESIAN_POINT('Ctrl Pts',(-24.6608862532133,89.4291320182521,9.32044670309475));
#20380=CARTESIAN_POINT('Ctrl Pts',(-25.518008746329,89.8224060224424,9.26778564801186));
#20381=CARTESIAN_POINT('Ctrl Pts',(-26.016096172441,90.4854401035392,9.21512459292899));
#20382=CARTESIAN_POINT('Ctrl Pts',(-26.3393871214709,90.9157920981482,9.18094416278332));
#20383=CARTESIAN_POINT('Ctrl Pts',(-26.5114220034557,91.4597899508601,9.14676373263765));
#20384=CARTESIAN_POINT('Ctrl Pts',(-26.5149491154365,92.0017493991467,9.11258330249198));
#20385=CARTESIAN_POINT('Origin',(-24.,92.,12.2084234471775));
#20386=CARTESIAN_POINT('',(-27.078276640009,92.0007881209763,1.79157655282254));
#20387=CARTESIAN_POINT('',(-27.0686108047355,92.0003349297086,1.70842344717745));
#20388=CARTESIAN_POINT('',(-27.0735,92.0000000000001,12.2084234471775));
#20389=CARTESIAN_POINT('',(-23.2062007174672,89.0307770462543,0.999999999999999));
#20390=CARTESIAN_POINT('Ctrl Pts',(-27.0686108047355,92.0003349297086,1.70842344717745));
#20391=CARTESIAN_POINT('Ctrl Pts',(-27.0689532420951,92.4946153833655,1.68292651844981));
#20392=CARTESIAN_POINT('Ctrl Pts',(-26.723556593627,94.0092287415617,1.6047685346393));
#20393=CARTESIAN_POINT('Ctrl Pts',(-24.3539160917338,95.6088396578189,1.4739494957459));
#20394=CARTESIAN_POINT('Ctrl Pts',(-21.1687762982368,94.2698556568795,1.31596633049727));
#20395=CARTESIAN_POINT('Ctrl Pts',(-20.5566852567634,90.8667001441213,1.15798316524863));
#20396=CARTESIAN_POINT('Ctrl Pts',(-22.2237466982397,89.2934286920664,1.05266105508288));
#20397=CARTESIAN_POINT('Ctrl Pts',(-23.2062007174672,89.0307770462543,0.999999999999999));
#20398=CARTESIAN_POINT('',(-24.7937992825329,89.0307770462543,0.999999999999999));
#20399=CARTESIAN_POINT('Origin',(-24.,92.,0.999999999999999));
#20400=CARTESIAN_POINT('Ctrl Pts',(-27.078276640009,92.0007881209763,1.79157655282254));
#20401=CARTESIAN_POINT('Ctrl Pts',(-27.0784227334426,92.0437415110921,1.78934283757203));
#20402=CARTESIAN_POINT('Ctrl Pts',(-27.0582221315001,93.0992023691253,1.73444806723864));
#20403=CARTESIAN_POINT('Ctrl Pts',(-25.8523949517842,95.1179531681003,1.62689224182237));
#20404=CARTESIAN_POINT('Ctrl Pts',(-22.40096829048,95.2555127221397,1.46890907657374));
#20405=CARTESIAN_POINT('Ctrl Pts',(-20.4000492676845,92.4393710995324,1.3109259113251));
#20406=CARTESIAN_POINT('Ctrl Pts',(-21.6506968017521,89.2605902470592,1.15462288580052));
#20407=CARTESIAN_POINT('Ctrl Pts',(-23.8480943965222,88.774594383454,1.05098091535882));
#20408=CARTESIAN_POINT('Ctrl Pts',(-24.7957016814436,89.0256872793281,1.));
#20409=CARTESIAN_POINT('Origin',(-24.,92.,12.2084234471775));
#20410=CARTESIAN_POINT('',(-27.069948942502,92.0019027882837,2.79157655282254));
#20411=CARTESIAN_POINT('',(-27.0750082483734,91.9974244677008,2.70842344717745));
#20412=CARTESIAN_POINT('',(-27.0735,92.0000000000001,12.2084234471775));
#20413=CARTESIAN_POINT('Ctrl Pts',(-27.0750082483734,91.9974244677008,2.70842344717745));
#20414=CARTESIAN_POINT('Ctrl Pts',(-27.0676141928259,92.8239896640293,2.66555951561375));
#20415=CARTESIAN_POINT('Ctrl Pts',(-26.2993639886887,94.678166986954,2.57003452896717));
#20416=CARTESIAN_POINT('Ctrl Pts',(-23.1738622446318,95.5314376817822,2.42184848723771));
#20417=CARTESIAN_POINT('Ctrl Pts',(-20.5910236590807,93.2380222607045,2.26386532198907));
#20418=CARTESIAN_POINT('Ctrl Pts',(-21.1003115510402,89.8216058212251,2.10588215674044));
#20419=CARTESIAN_POINT('Ctrl Pts',(-24.2395757883417,88.3812154557912,1.94789899149181));
#20420=CARTESIAN_POINT('Ctrl Pts',(-26.6902007202702,89.9256564305863,1.81541275497081));
#20421=CARTESIAN_POINT('Ctrl Pts',(-27.0682459760221,91.4737343794429,1.73558757353269));
#20422=CARTESIAN_POINT('Ctrl Pts',(-27.0686108047355,92.0003349297086,1.70842344717745));
#20423=CARTESIAN_POINT('Ctrl Pts',(-27.069948942502,92.0019027882837,2.79157655282254));
#20424=CARTESIAN_POINT('Ctrl Pts',(-27.072121005747,92.3814602607307,2.77197583473597));
#20425=CARTESIAN_POINT('Ctrl Pts',(-26.8315578651691,93.7781155062161,2.69971406156651));
#20426=CARTESIAN_POINT('Ctrl Pts',(-24.7514083303165,95.5481002919865,2.57479123331418));
#20427=CARTESIAN_POINT('Ctrl Pts',(-21.4392014827728,94.5682622165549,2.41680806806554));
#20428=CARTESIAN_POINT('Ctrl Pts',(-20.4497281061605,91.2589110713399,2.25882490281691));
#20429=CARTESIAN_POINT('Ctrl Pts',(-22.6804688187274,88.6217765261786,2.10084173756827));
#20430=CARTESIAN_POINT('Ctrl Pts',(-26.0596141395782,89.0427206231847,1.94509228757015));
#20431=CARTESIAN_POINT('Ctrl Pts',(-27.0749785010789,91.0310919164918,1.84200389265491));
#20432=CARTESIAN_POINT('Ctrl Pts',(-27.078276640009,92.0007881209763,1.79157655282254));
#20433=CARTESIAN_POINT('Origin',(-24.,92.,12.2084234471775));
#20434=CARTESIAN_POINT('',(-27.0716996757212,91.9974284306968,3.79157655282255));
#20435=CARTESIAN_POINT('',(-27.0762204956331,92.0022328813937,3.70842344717745));
#20436=CARTESIAN_POINT('',(-27.0735,92.0000000000001,12.2084234471775));
#20437=CARTESIAN_POINT('Ctrl Pts',(-27.0762204956331,92.0022328813937,3.70842344717745));
#20438=CARTESIAN_POINT('Ctrl Pts',(-27.0774152743552,92.1480569517705,3.70085356786056));
#20439=CARTESIAN_POINT('Ctrl Pts',(-27.0019699142738,93.3070874795555,3.6406226334608));
#20440=CARTESIAN_POINT('Ctrl Pts',(-25.5299145201095,95.2883129487163,3.52773064397815));
#20441=CARTESIAN_POINT('Ctrl Pts',(-22.0822081585386,95.0782646692958,3.36974747872952));
#20442=CARTESIAN_POINT('Ctrl Pts',(-20.3740039924776,92.0761257570406,3.21176431348088));
#20443=CARTESIAN_POINT('Ctrl Pts',(-21.9547029138477,89.0049371841951,3.05378114823225));
#20444=CARTESIAN_POINT('Ctrl Pts',(-25.3905541717125,88.6503748565914,2.89579798298361));
#20445=CARTESIAN_POINT('Ctrl Pts',(-26.9751243964845,90.605903680769,2.78067874929868));
#20446=CARTESIAN_POINT('Ctrl Pts',(-27.0766982584323,91.8085019627027,2.71822057069663));
#20447=CARTESIAN_POINT('Ctrl Pts',(-27.0750082483734,91.9974244677008,2.70842344717745));
#20448=CARTESIAN_POINT('Ctrl Pts',(-27.0716996757212,91.9974284306968,3.79157655282255));
#20449=CARTESIAN_POINT('Ctrl Pts',(-27.0659413561646,92.7122593975924,3.7546088318999));
#20450=CARTESIAN_POINT('Ctrl Pts',(-26.4623933413542,94.4541466296605,3.66498005589438));
#20451=CARTESIAN_POINT('Ctrl Pts',(-23.5706310470027,95.6012890799134,3.52269022480599));
#20452=CARTESIAN_POINT('Ctrl Pts',(-20.7493847378944,93.6084593551842,3.36470705955735));
#20453=CARTESIAN_POINT('Ctrl Pts',(-20.8765574469375,90.1567019355188,3.20672389430872));
#20454=CARTESIAN_POINT('Ctrl Pts',(-23.8367991104361,88.3768791020246,3.04874072906008));
#20455=CARTESIAN_POINT('Ctrl Pts',(-26.5594315108873,89.6964445021905,2.91035828189802));
#20456=CARTESIAN_POINT('Ctrl Pts',(-27.0662853449471,91.3617069600934,2.82463688981884));
#20457=CARTESIAN_POINT('Ctrl Pts',(-27.069948942502,92.0019027882837,2.79157655282254));
#20458=CARTESIAN_POINT('Origin',(-24.,92.,12.2084234471775));
#20459=CARTESIAN_POINT('',(-27.0783836922344,92.0005832748178,4.79157655282255));
#20460=CARTESIAN_POINT('',(-27.0687189181701,92.0004324466973,4.70842344717745));
#20461=CARTESIAN_POINT('',(-27.0735,92.0000000000001,12.2084234471775));
#20462=CARTESIAN_POINT('Ctrl Pts',(-27.0687189181701,92.0004324466973,4.70842344717746));
#20463=CARTESIAN_POINT('Ctrl Pts',(-27.0693320714153,92.4838070199057,4.6834865650245));
#20464=CARTESIAN_POINT('Ctrl Pts',(-26.734694995182,93.9871566204806,4.60588862778867));
#20465=CARTESIAN_POINT('Ctrl Pts',(-24.3913282534434,95.6056209517321,4.47562963546996));
#20466=CARTESIAN_POINT('Ctrl Pts',(-21.1942539711864,94.2981360810344,4.31764647022132));
#20467=CARTESIAN_POINT('Ctrl Pts',(-20.5420870968054,90.9061633512837,4.15966330497269));
#20468=CARTESIAN_POINT('Ctrl Pts',(-23.0263652646397,88.5063377831116,4.00168013972405));
#20469=CARTESIAN_POINT('Ctrl Pts',(-26.232411992584,89.2385337482431,3.85126685379231));
#20470=CARTESIAN_POINT('Ctrl Pts',(-27.0691036084141,91.1336088897795,3.75351462294344));
#20471=CARTESIAN_POINT('Ctrl Pts',(-27.0762204956331,92.0022328813937,3.70842344717745));
#20472=CARTESIAN_POINT('Ctrl Pts',(-27.0783836922344,92.0005832748178,4.79157655282255));
#20473=CARTESIAN_POINT('Ctrl Pts',(-27.078468271904,92.0327646232159,4.78990288414672));
#20474=CARTESIAN_POINT('Ctrl Pts',(-27.0634880644545,93.0774335875127,4.73556816038801));
#20475=CARTESIAN_POINT('Ctrl Pts',(-25.8851896583917,95.0983384007904,4.62857238154643));
#20476=CARTESIAN_POINT('Ctrl Pts',(-22.4354577715254,95.2719792949115,4.47058921629779));
#20477=CARTESIAN_POINT('Ctrl Pts',(-20.4048190868974,92.4778232899584,4.31260605104916));
#20478=CARTESIAN_POINT('Ctrl Pts',(-21.6351322020288,89.2502652496793,4.15462288580052));
#20479=CARTESIAN_POINT('Ctrl Pts',(-25.010461127225,88.5168104867762,3.99663972055189));
#20480=CARTESIAN_POINT('Ctrl Pts',(-26.893911960326,90.3750681296893,3.8756242762259));
#20481=CARTESIAN_POINT('Ctrl Pts',(-27.0741441659616,91.693972308664,3.80726988698278));
#20482=CARTESIAN_POINT('Ctrl Pts',(-27.0716996757212,91.9974284306968,3.79157655282255));
#20483=CARTESIAN_POINT('Origin',(-24.,92.,12.2084234471775));
#20484=CARTESIAN_POINT('',(-27.0701623993453,92.0020253450063,5.79157655282255));
#20485=CARTESIAN_POINT('',(-27.0746893422025,91.9973677267577,5.70842344717746));
#20486=CARTESIAN_POINT('',(-27.0735,92.0000000000001,12.2084234471775));
#20487=CARTESIAN_POINT('Ctrl Pts',(-27.0746893422025,91.9973677267577,5.70842344717746));
#20488=CARTESIAN_POINT('Ctrl Pts',(-27.0673208895816,92.8133508051795,5.66611956218844));
#20489=CARTESIAN_POINT('Ctrl Pts',(-26.3157336914085,94.657090117177,5.57115462211654));
#20490=CARTESIAN_POINT('Ctrl Pts',(-23.2111785026033,95.5399718768618,5.42352862696177));
#20491=CARTESIAN_POINT('Ctrl Pts',(-20.6043014164074,93.2739196885051,5.26554546171313));
#20492=CARTESIAN_POINT('Ctrl Pts',(-21.0774388479142,89.8523788611612,5.1075622964645));
#20493=CARTESIAN_POINT('Ctrl Pts',(-24.2014389978196,88.3788037094653,4.94957913121586));
#20494=CARTESIAN_POINT('Ctrl Pts',(-26.6784589321776,89.9039237459709,4.81653284812018));
#20495=CARTESIAN_POINT('Ctrl Pts',(-27.0680372304395,91.4630292470767,4.73614762010738));
#20496=CARTESIAN_POINT('Ctrl Pts',(-27.0687189181701,92.0004324466973,4.70842344717746));
#20497=CARTESIAN_POINT('Ctrl Pts',(-27.0701623993453,92.0020253450063,5.79157655282255));
#20498=CARTESIAN_POINT('Ctrl Pts',(-27.0724185577782,92.3706733312739,5.77253588131066));
#20499=CARTESIAN_POINT('Ctrl Pts',(-26.840929369154,93.7561580997579,5.70083415471589));
#20500=CARTESIAN_POINT('Ctrl Pts',(-24.7888215168716,95.5399719642594,5.57647137303822));
#20501=CARTESIAN_POINT('Ctrl Pts',(-21.4664563263011,94.5951488100945,5.41848820778961));
#20502=CARTESIAN_POINT('Ctrl Pts',(-20.4421017230708,91.2964371072188,5.26050504254096));
#20503=CARTESIAN_POINT('Ctrl Pts',(-22.6448822957049,88.6358809621643,5.10252187729233));
#20504=CARTESIAN_POINT('Ctrl Pts',(-26.0404432418415,89.0225553310303,4.94621238071952));
#20505=CARTESIAN_POINT('Ctrl Pts',(-27.075807019589,91.0201963741306,4.84256393922959));
#20506=CARTESIAN_POINT('Ctrl Pts',(-27.0783836922344,92.0005832748178,4.79157655282255));
#20507=CARTESIAN_POINT('Origin',(-24.,92.,12.2084234471775));
#20508=CARTESIAN_POINT('',(-27.0714153574487,91.9974952077453,6.79157655282255));
#20509=CARTESIAN_POINT('',(-27.0765039205242,92.0021186989274,6.70842344717745));
#20510=CARTESIAN_POINT('',(-27.0735,92.0000000000001,12.2084234471775));
#20511=CARTESIAN_POINT('Ctrl Pts',(-27.0765039205242,92.0021186989274,6.70842344717745));
#20512=CARTESIAN_POINT('Ctrl Pts',(-27.0775698549682,92.1371216997451,6.70141361443525));
#20513=CARTESIAN_POINT('Ctrl Pts',(-27.0084022542901,93.2852297742065,6.64174272661016));
#20514=CARTESIAN_POINT('Ctrl Pts',(-25.5645421898479,95.27197921413,6.5294107837022));
#20515=CARTESIAN_POINT('Ctrl Pts',(-22.1148103881513,95.0983383242963,6.37142761845358));
#20516=CARTESIAN_POINT('Ctrl Pts',(-20.3750099098822,92.114398820868,6.21344445320493));
#20517=CARTESIAN_POINT('Ctrl Pts',(-21.9231991720717,89.0266956824957,6.05546128795631));
#20518=CARTESIAN_POINT('Ctrl Pts',(-25.355117670839,88.6358810452203,5.89747812270766));
#20519=CARTESIAN_POINT('Ctrl Pts',(-26.9680494317645,90.584007681798,5.78179884244805));
#20520=CARTESIAN_POINT('Ctrl Pts',(-27.0764933447696,91.7975923269541,5.71878061727132));
#20521=CARTESIAN_POINT('Ctrl Pts',(-27.0746893422025,91.9973677267577,5.70842344717746));
#20522=CARTESIAN_POINT('Ctrl Pts',(-27.0714153574487,91.9974952077453,6.79157655282255));
#20523=CARTESIAN_POINT('Ctrl Pts',(-27.0659291292545,92.7016618298241,6.75516887847459));
#20524=CARTESIAN_POINT('Ctrl Pts',(-26.4768296167088,94.4326507862167,6.66610014904376));
#20525=CARTESIAN_POINT('Ctrl Pts',(-23.6086717368945,95.6056210407497,6.52437036453004));
#20526=CARTESIAN_POINT('Ctrl Pts',(-20.7665454640887,93.6426845888844,6.36638719928141));
#20527=CARTESIAN_POINT('Ctrl Pts',(-20.857272821619,90.1897771481731,6.20840403403277));
#20528=CARTESIAN_POINT('Ctrl Pts',(-23.7985609972073,88.3788036200625,6.05042086878414));
#20529=CARTESIAN_POINT('Ctrl Pts',(-26.5460460301536,89.6747784855977,5.91147837504739));
#20530=CARTESIAN_POINT('Ctrl Pts',(-27.0661786684217,91.351098370438,5.82519693639353));
#20531=CARTESIAN_POINT('Ctrl Pts',(-27.0701623993453,92.0020253450063,5.79157655282255));
#20532=CARTESIAN_POINT('Origin',(-24.,92.,12.2084234471775));
#20533=CARTESIAN_POINT('',(-27.0784606140442,92.000390174329,7.79157655282255));
#20534=CARTESIAN_POINT('',(-27.0687739277024,92.0006038359779,7.70842344717745));
#20535=CARTESIAN_POINT('',(-27.0735,92.0000000000001,12.2084234471775));
#20536=CARTESIAN_POINT('Ctrl Pts',(-27.0687739277024,92.0006038359779,7.70842344717745));
#20537=CARTESIAN_POINT('Ctrl Pts',(-27.0696117452305,92.4731013478073,7.68404661159918));
#20538=CARTESIAN_POINT('Ctrl Pts',(-26.745518655979,93.9652418365262,7.60700872093803));
#20539=CARTESIAN_POINT('Ctrl Pts',(-24.4293689423972,95.6012889909869,7.47730977519402));
#20540=CARTESIAN_POINT('Ctrl Pts',(-21.2186704291245,94.3276267101463,7.31932660994538));
#20541=CARTESIAN_POINT('Ctrl Pts',(-20.5307327633938,90.9427275180138,7.16134344469674));
#20542=CARTESIAN_POINT('Ctrl Pts',(-22.9895388977221,88.5168105727741,7.00336027944811));
#20543=CARTESIAN_POINT('Ctrl Pts',(-26.2151018414649,89.2177213748181,6.85238694694168));
#20544=CARTESIAN_POINT('Ctrl Pts',(-27.0695620701135,91.1229176917646,6.75407466951813));
#20545=CARTESIAN_POINT('Ctrl Pts',(-27.0765039205242,92.0021186989274,6.70842344717745));
#20546=CARTESIAN_POINT('Ctrl Pts',(-27.0784606140442,92.000390174329,7.79157655282255));
#20547=CARTESIAN_POINT('Ctrl Pts',(-27.0784992224434,92.0218014961978,7.79046293072141));
#20548=CARTESIAN_POINT('Ctrl Pts',(-27.0686358124042,93.0556766999574,7.73668825353738));
#20549=CARTESIAN_POINT('Ctrl Pts',(-25.9177918888646,95.0782647453892,7.63025252127048));
#20550=CARTESIAN_POINT('Ctrl Pts',(-22.4700854420894,95.288313029852,7.47226935602185));
#20551=CARTESIAN_POINT('Ctrl Pts',(-20.4100634919605,92.5157489192991,7.31428619077322));
#20552=CARTESIAN_POINT('Ctrl Pts',(-21.6062365978313,89.275383052732,7.15630302552458));
#20553=CARTESIAN_POINT('Ctrl Pts',(-24.9736347594025,88.5063376968639,6.99831986027595));
#20554=CARTESIAN_POINT('Ctrl Pts',(-26.8854039328385,90.3531166132715,6.87674436937527));
#20555=CARTESIAN_POINT('Ctrl Pts',(-27.0738645596358,91.6831359850143,6.80782993355747));
#20556=CARTESIAN_POINT('Ctrl Pts',(-27.0714153574487,91.9974952077453,6.79157655282255));
#20557=CARTESIAN_POINT('Origin',(-24.,92.,12.2084234471775));
#20558=CARTESIAN_POINT('',(-27.0703857423214,92.0021357609841,8.79157655282255));
#20559=CARTESIAN_POINT('',(-27.0743674416594,91.9973209105276,8.70842344717745));
#20560=CARTESIAN_POINT('',(-27.0735,92.0000000000001,12.2084234471775));
#20561=CARTESIAN_POINT('Ctrl Pts',(-27.0743674416594,91.9973209105276,8.70842344717745));
#20562=CARTESIAN_POINT('Ctrl Pts',(-27.0670571899902,92.8027184781566,8.66667960876312));
#20563=CARTESIAN_POINT('Ctrl Pts',(-26.3319128073199,94.6359725607219,8.57227471526591));
#20564=CARTESIAN_POINT('Ctrl Pts',(-23.24859168833,95.5481002036266,8.42520876668582));
#20565=CARTESIAN_POINT('Ctrl Pts',(-20.6179387947979,93.3096959362796,8.26722560143718));
#20566=CARTESIAN_POINT('Ctrl Pts',(-21.0549304174885,89.8833499742237,8.10924243618856));
#20567=CARTESIAN_POINT('Ctrl Pts',(-24.1632008855267,88.3768791915844,7.95125927093991));
#20568=CARTESIAN_POINT('Ctrl Pts',(-26.6666765768248,89.8820749507615,7.81765294126956));
#20569=CARTESIAN_POINT('Ctrl Pts',(-27.0678018156826,91.4523692918733,7.73670766668206));
#20570=CARTESIAN_POINT('Ctrl Pts',(-27.0687739277024,92.0006038359779,7.70842344717745));
#20571=CARTESIAN_POINT('Ctrl Pts',(-27.0703857423214,92.0021357609841,8.79157655282255));
#20572=CARTESIAN_POINT('Ctrl Pts',(-27.0727139521361,92.3598775376807,8.77309592788534));
#20573=CARTESIAN_POINT('Ctrl Pts',(-26.8501666541559,93.7342139358697,8.70195424786525));
#20574=CARTESIAN_POINT('Ctrl Pts',(-24.8261377777637,95.5314377737091,8.57815151276229));
#20575=CARTESIAN_POINT('Ctrl Pts',(-21.493997547754,94.6217541894132,8.42016834751366));
#20576=CARTESIAN_POINT('Ctrl Pts',(-20.4348706359933,91.3340326759415,8.26218518226502));
#20577=CARTESIAN_POINT('Ctrl Pts',(-22.6094457936036,88.6503747732116,8.10420201701639));
#20578=CARTESIAN_POINT('Ctrl Pts',(-26.0210778474872,89.0024378034505,7.94733247386889));
#20579=CARTESIAN_POINT('Ctrl Pts',(-27.0766735052339,91.0093011164261,7.84312398580429));
#20580=CARTESIAN_POINT('Ctrl Pts',(-27.0784606140442,92.000390174329,7.79157655282255));
#20581=CARTESIAN_POINT('Origin',(-24.,92.,12.2084234471775));
#20582=CARTESIAN_POINT('',(-27.0702888275776,91.9968971804147,9.79157655282255));
#20583=CARTESIAN_POINT('',(-27.076766805402,92.0019372679897,9.70842344717746));
#20584=CARTESIAN_POINT('',(-27.0735,92.0000000000001,12.2084234471775));
#20585=CARTESIAN_POINT('',(-24.7937992825329,89.0307770462543,10.));
#20586=CARTESIAN_POINT('Ctrl Pts',(-24.7937992825329,89.0307770462543,10.));
#20587=CARTESIAN_POINT('Ctrl Pts',(-25.7762533017603,89.2934286920664,9.94733894491712));
#20588=CARTESIAN_POINT('Ctrl Pts',(-26.8759105460538,90.3312191677288,9.87786446252464));
#20589=CARTESIAN_POINT('Ctrl Pts',(-27.0726356002046,91.6716361186704,9.80838998013215));
#20590=CARTESIAN_POINT('Ctrl Pts',(-27.0702888275776,91.9968971804148,9.79157655282255));
#20591=CARTESIAN_POINT('',(-23.2043027735401,89.0256991239338,10.));
#20592=CARTESIAN_POINT('Origin',(-24.,92.,10.));
#20593=CARTESIAN_POINT('Ctrl Pts',(-23.2042983602306,89.0256873161863,10.));
#20594=CARTESIAN_POINT('Ctrl Pts',(-24.1519057059922,88.7745943606123,9.94901908464117));
#20595=CARTESIAN_POINT('Ctrl Pts',(-26.2125558943074,89.2303462451956,9.851826900367));
#20596=CARTESIAN_POINT('Ctrl Pts',(-27.0700735870785,91.1123260926059,9.75463471609281));
#20597=CARTESIAN_POINT('Ctrl Pts',(-27.076766805402,92.0019372679896,9.70842344717745));
#20598=CARTESIAN_POINT('Origin',(-24.,-92.,5.));
#20599=CARTESIAN_POINT('',(-26.5134954281454,-91.9997257032743,1.38741669750802));
#20600=CARTESIAN_POINT('',(-26.5156258041287,-92.0035321038279,1.11258330249198));
#20601=CARTESIAN_POINT('',(-26.5175,-92.,5.));
#20602=CARTESIAN_POINT('',(-25.913465996665,-90.364012796625,0.999999999999999));
#20603=CARTESIAN_POINT('Ctrl Pts',(-26.5156258041287,-92.0035321038279,
1.11258330249198));
#20604=CARTESIAN_POINT('Ctrl Pts',(-26.5104632893492,-91.410913677985,1.07505553499465));
#20605=CARTESIAN_POINT('Ctrl Pts',(-26.299221828084,-90.8151964396956,1.03752776749732));
#20606=CARTESIAN_POINT('Ctrl Pts',(-25.913465996665,-90.364012796625,0.999999999999993));
#20607=CARTESIAN_POINT('',(-26.5175,-92.,1.));
#20608=CARTESIAN_POINT('Origin',(-24.,-92.,1.));
#20609=CARTESIAN_POINT('',(-26.5175,-92.,0.));
#20610=CARTESIAN_POINT('',(-26.5175,-92.,5.));
#20611=CARTESIAN_POINT('Origin',(-24.,-92.,0.));
#20612=CARTESIAN_POINT('',(-22.0828967253639,-90.3614656719992,1.));
#20613=CARTESIAN_POINT('Origin',(-24.,-92.,1.));
#20614=CARTESIAN_POINT('Ctrl Pts',(-22.0828882653787,-90.3614597476137,
1.));
#20615=CARTESIAN_POINT('Ctrl Pts',(-22.6060429859409,-89.7523041107177,
1.05098091535882));
#20616=CARTESIAN_POINT('Ctrl Pts',(-23.4465812877835,-89.4121723295192,
1.10196183071765));
#20617=CARTESIAN_POINT('Ctrl Pts',(-24.2457357736239,-89.4905147002801,
1.15294274607647));
#20618=CARTESIAN_POINT('Ctrl Pts',(-25.0712273934265,-89.5714389416932,
1.20560380115935));
#20619=CARTESIAN_POINT('Ctrl Pts',(-25.8525625390091,-90.0988745222663,
1.25826485624222));
#20620=CARTESIAN_POINT('Ctrl Pts',(-26.2358880111547,-90.8341462678707,
1.3109259113251));
#20621=CARTESIAN_POINT('Ctrl Pts',(-26.4214828919903,-91.1901431476069,
1.33642284005274));
#20622=CARTESIAN_POINT('Ctrl Pts',(-26.5137759227878,-91.5948612017176,
1.36191976878038));
#20623=CARTESIAN_POINT('Ctrl Pts',(-26.5134954281454,-91.9997257032743,
1.38741669750802));
#20624=CARTESIAN_POINT('Origin',(-24.,-92.,5.));
#20625=CARTESIAN_POINT('',(-26.5187355654992,-92.0021096152222,2.38741669750802));
#20626=CARTESIAN_POINT('',(-26.5214126870217,-91.999354461019,2.11258330249198));
#20627=CARTESIAN_POINT('',(-26.5175,-92.,5.));
#20628=CARTESIAN_POINT('Ctrl Pts',(-26.5214126870217,-91.999354461019,2.11258330249198));
#20629=CARTESIAN_POINT('Ctrl Pts',(-26.5215323520691,-91.9641713906796,
2.11034958724147));
#20630=CARTESIAN_POINT('Ctrl Pts',(-26.5208590695048,-91.928993057358,2.10811587199095));
#20631=CARTESIAN_POINT('Ctrl Pts',(-26.5193785186672,-91.8938487960073,
2.10588215674044));
#20632=CARTESIAN_POINT('Ctrl Pts',(-26.4844737253229,-91.0653036703885,
2.05322110165756));
#20633=CARTESIAN_POINT('Ctrl Pts',(-26.0008841105951,-90.25569596213,2.00056004657468));
#20634=CARTESIAN_POINT('Ctrl Pts',(-25.2879127216155,-89.8321129915859,
1.9478989914918));
#20635=CARTESIAN_POINT('Ctrl Pts',(-24.5749413326358,-89.4085300210418,
1.89523793640892));
#20636=CARTESIAN_POINT('Ctrl Pts',(-23.6325881694044,-89.370971788212,1.84257688132604));
#20637=CARTESIAN_POINT('Ctrl Pts',(-22.8882532181424,-89.7366423255222,
1.78991582624316));
#20638=CARTESIAN_POINT('Ctrl Pts',(-22.1439182668803,-90.1023128628323,
1.73725477116029));
#20639=CARTESIAN_POINT('Ctrl Pts',(-21.5976015275877,-90.8712121702823,
1.68459371607741));
#20640=CARTESIAN_POINT('Ctrl Pts',(-21.4970123488694,-91.6942825335227,
1.63193266099453));
#20641=CARTESIAN_POINT('Ctrl Pts',(-21.3964231701512,-92.5173528967631,
1.57927160591165));
#20642=CARTESIAN_POINT('Ctrl Pts',(-21.7415615520075,-93.3945943157939,
1.52661055082878));
#20643=CARTESIAN_POINT('Ctrl Pts',(-22.3760119861909,-93.9288768514158,
1.4739494957459));
#20644=CARTESIAN_POINT('Ctrl Pts',(-23.0104624203743,-94.4631593870375,
1.42128844066302));
#20645=CARTESIAN_POINT('Ctrl Pts',(-23.934224906885,-94.6544830392504,1.36862738558014));
#20646=CARTESIAN_POINT('Ctrl Pts',(-24.7281293260075,-94.4146105531457,
1.31596633049726));
#20647=CARTESIAN_POINT('Ctrl Pts',(-25.5220337451301,-94.1747380670411,
1.26330527541438));
#20648=CARTESIAN_POINT('Ctrl Pts',(-26.1860800968646,-93.503669442619,1.21064422033151));
#20649=CARTESIAN_POINT('Ctrl Pts',(-26.4192666807451,-92.7092696340464,
1.15798316524863));
#20650=CARTESIAN_POINT('Ctrl Pts',(-26.4862778644254,-92.4809817514334,
1.14284987766308));
#20651=CARTESIAN_POINT('Ctrl Pts',(-26.5177076178372,-92.2425088846187,
1.12771659007753));
#20652=CARTESIAN_POINT('Ctrl Pts',(-26.5156258041287,-92.0035321038279,
1.11258330249198));
#20653=CARTESIAN_POINT('Ctrl Pts',(-26.5134954281454,-91.9997257032743,
1.38741669750802));
#20654=CARTESIAN_POINT('Ctrl Pts',(-26.5131965924704,-92.4310635555512,
1.41458082386326));
#20655=CARTESIAN_POINT('Ctrl Pts',(-26.4078219950606,-92.8625676332891,
1.4417449502185));
#20656=CARTESIAN_POINT('Ctrl Pts',(-26.1982523776868,-93.2354979308673,
1.46890907657374));
#20657=CARTESIAN_POINT('Ctrl Pts',(-25.7919754733646,-93.9584699376238,
1.52157013165662));
#20658=CARTESIAN_POINT('Ctrl Pts',(-24.9941058660117,-94.4613060405015,
1.57423118673949));
#20659=CARTESIAN_POINT('Ctrl Pts',(-24.1666097958723,-94.5160870716528,
1.62689224182237));
#20660=CARTESIAN_POINT('Ctrl Pts',(-23.3391137257328,-94.5708681028041,
1.67955329690525));
#20661=CARTESIAN_POINT('Ctrl Pts',(-22.4819911928069,-94.1775940622292,
1.73221435198813));
#20662=CARTESIAN_POINT('Ctrl Pts',(-21.9839037459974,-93.5145599501885,
1.78487540707101));
#20663=CARTESIAN_POINT('Ctrl Pts',(-21.4858162991878,-92.8515258381478,
1.83753646215388));
#20664=CARTESIAN_POINT('Ctrl Pts',(-21.3467639384947,-91.9187316546413,
1.89019751723676));
#20665=CARTESIAN_POINT('Ctrl Pts',(-21.6298377538243,-91.1392455882325,
1.94285857231964));
#20666=CARTESIAN_POINT('Ctrl Pts',(-21.912911569154,-90.3597595218238,1.99551962740252));
#20667=CARTESIAN_POINT('Ctrl Pts',(-22.6181115605066,-89.7335815725127,
2.0481806824854));
#20668=CARTESIAN_POINT('Ctrl Pts',(-23.425603556166,-89.5446793850464,2.10084173756827));
#20669=CARTESIAN_POINT('Ctrl Pts',(-24.2330955518254,-89.35577719758,2.15350279265115));
#20670=CARTESIAN_POINT('Ctrl Pts',(-25.1428795517915,-89.6041507719583,
2.20616384773403));
#20671=CARTESIAN_POINT('Ctrl Pts',(-25.7423598115282,-90.1771656715372,
2.25882490281691));
#20672=CARTESIAN_POINT('Ctrl Pts',(-26.2303120712523,-90.6435762172788,
2.30168883438061));
#20673=CARTESIAN_POINT('Ctrl Pts',(-26.512679103923,-91.325071055923,2.34455276594432));
#20674=CARTESIAN_POINT('Ctrl Pts',(-26.5187355654992,-92.0021096152222,
2.38741669750802));
#20675=CARTESIAN_POINT('Origin',(-24.,-92.,5.));
#20676=CARTESIAN_POINT('',(-26.5197285159005,-91.9981710495135,3.38741669750802));
#20677=CARTESIAN_POINT('',(-26.5145914825342,-91.9984414286209,3.11258330249198));
#20678=CARTESIAN_POINT('',(-26.5175,-92.,5.));
#20679=CARTESIAN_POINT('Ctrl Pts',(-26.5145914825342,-91.9984414286209,
3.11258330249198));
#20680=CARTESIAN_POINT('Ctrl Pts',(-26.5163706169191,-91.687546359978,3.0929825844054));
#20681=CARTESIAN_POINT('Ctrl Pts',(-26.4629229514308,-91.3772412892129,
3.07338186631882));
#20682=CARTESIAN_POINT('Ctrl Pts',(-26.3514583308843,-91.0894032152641,
3.05378114823224));
#20683=CARTESIAN_POINT('Ctrl Pts',(-26.0519874392331,-90.3160715138328,
3.00112009314936));
#20684=CARTESIAN_POINT('Ctrl Pts',(-25.3337325490401,-89.7049134175565,
2.94845903806649));
#20685=CARTESIAN_POINT('Ctrl Pts',(-24.52243433036,-89.5330984014484,2.89579798298361));
#20686=CARTESIAN_POINT('Ctrl Pts',(-23.7111361116798,-89.3612833853403,
2.84313692790073));
#20687=CARTESIAN_POINT('Ctrl Pts',(-22.8067945645126,-89.6288114494004,
2.79047587281785));
#20688=CARTESIAN_POINT('Ctrl Pts',(-22.219544382578,-90.2143564031656,2.73781481773497));
#20689=CARTESIAN_POINT('Ctrl Pts',(-21.6322942006435,-90.7999013569307,
2.68515376265209));
#20690=CARTESIAN_POINT('Ctrl Pts',(-21.3621353839418,-91.703463200401,2.63249270756922));
#20691=CARTESIAN_POINT('Ctrl Pts',(-21.5315888137355,-92.515256413142,2.57983165248634));
#20692=CARTESIAN_POINT('Ctrl Pts',(-21.7010422435292,-93.327049625883,2.52717059740346));
#20693=CARTESIAN_POINT('Ctrl Pts',(-22.3101079198185,-94.0470742078948,
2.47450954232058));
#20694=CARTESIAN_POINT('Ctrl Pts',(-23.0825657012675,-94.3487965351803,
2.4218484872377));
#20695=CARTESIAN_POINT('Ctrl Pts',(-23.8550234827164,-94.6505188624658,
2.36918743215482));
#20696=CARTESIAN_POINT('Ctrl Pts',(-24.7908733693249,-94.5339389350251,
2.31652637707195));
#20697=CARTESIAN_POINT('Ctrl Pts',(-25.4656883266487,-94.0519076998152,
2.26386532198907));
#20698=CARTESIAN_POINT('Ctrl Pts',(-26.1118797697061,-93.5903227036641,
2.21343798215671));
#20699=CARTESIAN_POINT('Ctrl Pts',(-26.5187111833227,-92.7936314593702,
2.16301064232434));
#20700=CARTESIAN_POINT('Ctrl Pts',(-26.5214126870217,-91.999354461019,2.11258330249198));
#20701=CARTESIAN_POINT('Ctrl Pts',(-26.5187355654992,-92.0021096152222,
2.38741669750802));
#20702=CARTESIAN_POINT('Ctrl Pts',(-26.5201198506077,-92.1568558120996,
2.39721382102719));
#20703=CARTESIAN_POINT('Ctrl Pts',(-26.5070693393431,-92.3113692075874,
2.40701094454637));
#20704=CARTESIAN_POINT('Ctrl Pts',(-26.4787395411232,-92.4630283942082,
2.41680806806554));
#20705=CARTESIAN_POINT('Ctrl Pts',(-26.3264624914741,-93.2782199925207,
2.46946912314842));
#20706=CARTESIAN_POINT('Ctrl Pts',(-25.7327318726689,-94.0109469643662,
2.5221301782313));
#20707=CARTESIAN_POINT('Ctrl Pts',(-24.9668162894688,-94.3289068537565,
2.57479123331418));
#20708=CARTESIAN_POINT('Ctrl Pts',(-24.2009007062687,-94.6468667431468,
2.62745228839706));
#20709=CARTESIAN_POINT('Ctrl Pts',(-23.2628001586737,-94.5500595500819,
2.68011334347993));
#20710=CARTESIAN_POINT('Ctrl Pts',(-22.5779584534227,-94.0823881414071,
2.73277439856281));
#20711=CARTESIAN_POINT('Ctrl Pts',(-21.8931167481717,-93.6147167327323,
2.78543545364569));
#20712=CARTESIAN_POINT('Ctrl Pts',(-21.4615338852647,-92.7761811084476,
2.83809650872857));
#20713=CARTESIAN_POINT('Ctrl Pts',(-21.4789404507956,-91.9470718995605,
2.89075756381145));
#20714=CARTESIAN_POINT('Ctrl Pts',(-21.4963470163266,-91.1179626906734,
2.94341861889432));
#20715=CARTESIAN_POINT('Ctrl Pts',(-21.9627430102955,-90.2982798971839,
2.9960796739772));
#20716=CARTESIAN_POINT('Ctrl Pts',(-22.6666096977841,-89.8597634515608,
3.04874072906008));
#20717=CARTESIAN_POINT('Ctrl Pts',(-23.3704763852727,-89.4212470059377,
3.10140178414296));
#20718=CARTESIAN_POINT('Ctrl Pts',(-24.311813766281,-89.363896908181,3.15406283922584));
#20719=CARTESIAN_POINT('Ctrl Pts',(-25.063709367653,-89.7137225058316,3.20672389430872));
#20720=CARTESIAN_POINT('Ctrl Pts',(-25.8156049690249,-90.0635481034822,
3.25938494939159));
#20721=CARTESIAN_POINT('Ctrl Pts',(-26.3780587907605,-90.8205493965401,
3.31204600447447));
#20722=CARTESIAN_POINT('Ctrl Pts',(-26.4959883797686,-91.641413330862,3.36470705955735));
#20723=CARTESIAN_POINT('Ctrl Pts',(-26.5129404282089,-91.7594102245555,
3.37227693887424));
#20724=CARTESIAN_POINT('Ctrl Pts',(-26.520707157718,-91.8787267284854,3.37984681819113));
#20725=CARTESIAN_POINT('Ctrl Pts',(-26.5197285159005,-91.9981710495135,
3.38741669750802));
#20726=CARTESIAN_POINT('Origin',(-24.,-92.,5.));
#20727=CARTESIAN_POINT('',(-26.5135839828142,-91.9996457834291,4.38741669750802));
#20728=CARTESIAN_POINT('',(-26.5160255060301,-92.0021063693209,4.11258330249198));
#20729=CARTESIAN_POINT('',(-26.5175,-92.,5.));
#20730=CARTESIAN_POINT('Ctrl Pts',(-26.5160255060301,-92.0021063693209,
4.11258330249198));
#20731=CARTESIAN_POINT('Ctrl Pts',(-26.5113088734142,-91.4165891850021,
4.07561558156934));
#20732=CARTESIAN_POINT('Ctrl Pts',(-26.30740600999,-90.828109419245,4.03864786064669));
#20733=CARTESIAN_POINT('Ctrl Pts',(-25.9337853550359,-90.381662326268,4.00168013972405));
#20734=CARTESIAN_POINT('Ctrl Pts',(-25.4015573085244,-89.7456919616342,
3.94901908464117));
#20735=CARTESIAN_POINT('Ctrl Pts',(-24.5249308580447,-89.3979402061153,
3.89635802955829));
#20736=CARTESIAN_POINT('Ctrl Pts',(-23.7014710569733,-89.4961183997274,
3.84369697447542));
#20737=CARTESIAN_POINT('Ctrl Pts',(-22.8780112559018,-89.5942965933394,
3.79103591939254));
#20738=CARTESIAN_POINT('Ctrl Pts',(-22.1077181042387,-90.1384047360825,
3.73837486430966));
#20739=CARTESIAN_POINT('Ctrl Pts',(-21.7399326972187,-90.8816805318427,
3.68571380922678));
#20740=CARTESIAN_POINT('Ctrl Pts',(-21.3721472901988,-91.624956327603,3.6330527541439));
#20741=CARTESIAN_POINT('Ctrl Pts',(-21.406869627822,-92.5673997763804,3.58039169906102));
#20742=CARTESIAN_POINT('Ctrl Pts',(-21.8283525270324,-93.2815966241557,
3.52773064397815));
#20743=CARTESIAN_POINT('Ctrl Pts',(-22.2498354262427,-93.9957934719311,
3.47506958889527));
#20744=CARTESIAN_POINT('Ctrl Pts',(-23.0580788870402,-94.4817437187044,
3.42240853381239));
#20745=CARTESIAN_POINT('Ctrl Pts',(-23.8865307275917,-94.5190607694894,
3.36974747872951));
#20746=CARTESIAN_POINT('Ctrl Pts',(-24.7149825681432,-94.5563778202745,
3.31708642364663));
#20747=CARTESIAN_POINT('Ctrl Pts',(-25.5636427884488,-94.1450616750713,
3.26442536856375));
#20748=CARTESIAN_POINT('Ctrl Pts',(-26.0476294520469,-93.4716509491765,
3.21176431348088));
#20749=CARTESIAN_POINT('Ctrl Pts',(-26.3514737668842,-93.0488871914059,
3.17870397648458));
#20750=CARTESIAN_POINT('Ctrl Pts',(-26.5115906341944,-92.5228250606093,
3.14564363948828));
#20751=CARTESIAN_POINT('Ctrl Pts',(-26.5145914825342,-91.9984414286209,
3.11258330249198));
#20752=CARTESIAN_POINT('Ctrl Pts',(-26.5197285159005,-91.9981710495135,
3.38741669750802));
#20753=CARTESIAN_POINT('Ctrl Pts',(-26.5138990821199,-92.7096599185249,
3.43250787327401));
#20754=CARTESIAN_POINT('Ctrl Pts',(-26.1977684432012,-93.4256839637041,
3.47759904904));
#20755=CARTESIAN_POINT('Ctrl Pts',(-25.664320715776,-93.8943544806311,3.52269022480598));
#20756=CARTESIAN_POINT('Ctrl Pts',(-25.0413181064947,-94.4417051204924,
3.57535127988886));
#20757=CARTESIAN_POINT('Ctrl Pts',(-24.1219075316514,-94.6516798246292,
3.62801233497174));
#20758=CARTESIAN_POINT('Ctrl Pts',(-23.3230573666226,-94.4290514695956,
3.68067339005462));
#20759=CARTESIAN_POINT('Ctrl Pts',(-22.5242072015938,-94.206423114562,3.7333344451375));
#20760=CARTESIAN_POINT('Ctrl Pts',(-21.8459174463795,-93.5511917003581,
3.78599550022038));
#20761=CARTESIAN_POINT('Ctrl Pts',(-21.5958040861176,-92.7605158612689,
3.83865655530325));
#20762=CARTESIAN_POINT('Ctrl Pts',(-21.3456907258557,-91.9698400221797,
3.89131761038613));
#20763=CARTESIAN_POINT('Ctrl Pts',(-21.5237537605461,-91.0437197582053,
3.94397866546901));
#20764=CARTESIAN_POINT('Ctrl Pts',(-22.0492385624731,-90.4021664114935,
3.99663972055189));
#20765=CARTESIAN_POINT('Ctrl Pts',(-22.5747233644,-89.7606130647817,4.04930077563477));
#20766=CARTESIAN_POINT('Ctrl Pts',(-23.4476299335634,-89.4036266353326,
4.10196183071764));
#20767=CARTESIAN_POINT('Ctrl Pts',(-24.2720802450577,-89.4931065626282,
4.15462288580052));
#20768=CARTESIAN_POINT('Ctrl Pts',(-25.096530556552,-89.5825864899237,4.2072839408834));
#20769=CARTESIAN_POINT('Ctrl Pts',(-25.8725246103771,-90.1185327739639,
4.25994499596628));
#20770=CARTESIAN_POINT('Ctrl Pts',(-26.2481358593184,-90.8578846277675,
4.31260605104916));
#20771=CARTESIAN_POINT('Ctrl Pts',(-26.4260011420294,-91.2079940211105,
4.33754293320211));
#20772=CARTESIAN_POINT('Ctrl Pts',(-26.5140862159014,-91.6037142506574,
4.36247981535507));
#20773=CARTESIAN_POINT('Ctrl Pts',(-26.5135839828142,-91.9996457834291,
4.38741669750802));
#20774=CARTESIAN_POINT('Origin',(-24.,-92.,5.));
#20775=CARTESIAN_POINT('',(-26.5184743499735,-92.0021560918536,5.38741669750802));
#20776=CARTESIAN_POINT('',(-26.5215003759084,-91.9995222402991,5.11258330249198));
#20777=CARTESIAN_POINT('',(-26.5175,-92.,5.));
#20778=CARTESIAN_POINT('Ctrl Pts',(-26.5215003759084,-91.9995222402991,
5.11258330249198));
#20779=CARTESIAN_POINT('Ctrl Pts',(-26.521569655014,-91.9731625365728,5.11090963381615));
#20780=CARTESIAN_POINT('Ctrl Pts',(-26.5211916947534,-91.9468048672737,
5.10923596514032));
#20781=CARTESIAN_POINT('Ctrl Pts',(-26.5203603409136,-91.9204615063421,
5.10756229646449));
#20782=CARTESIAN_POINT('Ctrl Pts',(-26.4942022542029,-91.0915822896134,
5.05490124138162));
#20783=CARTESIAN_POINT('Ctrl Pts',(-26.0191794168034,-90.2768685179763,
5.00224018629873));
#20784=CARTESIAN_POINT('Ctrl Pts',(-25.3107227922661,-89.8458067909394,
4.94957913121586));
#20785=CARTESIAN_POINT('Ctrl Pts',(-24.6022661677289,-89.4147450639025,
4.89691807613298));
#20786=CARTESIAN_POINT('Ctrl Pts',(-23.6603757560539,-89.3673353814657,
4.8442570210501));
#20787=CARTESIAN_POINT('Ctrl Pts',(-22.9122149332711,-89.7250788434924,
4.79159596596722));
#20788=CARTESIAN_POINT('Ctrl Pts',(-22.1640541104882,-90.0828223055191,
4.73893491088435));
#20789=CARTESIAN_POINT('Ctrl Pts',(-21.6096228765975,-90.8457189120093,
4.68627385580147));
#20790=CARTESIAN_POINT('Ctrl Pts',(-21.5003652582016,-91.667782032718,4.63361280071859));
#20791=CARTESIAN_POINT('Ctrl Pts',(-21.3911076398056,-92.4898451534267,
4.58095174563571));
#20792=CARTESIAN_POINT('Ctrl Pts',(-21.7270236369044,-93.3710747883539,
4.52829069055283));
#20793=CARTESIAN_POINT('Ctrl Pts',(-22.3557696119043,-93.9118182580198,
4.47562963546995));
#20794=CARTESIAN_POINT('Ctrl Pts',(-22.9845155869041,-94.4525617276857,
4.42296858038707));
#20795=CARTESIAN_POINT('Ctrl Pts',(-23.906091539805,-94.6528190320904,4.3703075253042));
#20796=CARTESIAN_POINT('Ctrl Pts',(-24.7025470485768,-94.4217700679434,
4.31764647022132));
#20797=CARTESIAN_POINT('Ctrl Pts',(-25.4990025573486,-94.1907211037964,
4.26498541513844));
#20798=CARTESIAN_POINT('Ctrl Pts',(-26.1703376219913,-93.5283658710978,
4.21232436005556));
#20799=CARTESIAN_POINT('Ctrl Pts',(-26.412090333041,-92.7350937678741,4.15966330497269));
#20800=CARTESIAN_POINT('Ctrl Pts',(-26.484134200614,-92.4986935632772,4.14396997081245));
#20801=CARTESIAN_POINT('Ctrl Pts',(-26.5180277850428,-92.250666913513,4.12827663665222));
#20802=CARTESIAN_POINT('Ctrl Pts',(-26.5160255060301,-92.0021063693209,
4.11258330249198));
#20803=CARTESIAN_POINT('Ctrl Pts',(-26.5135839828142,-91.9996457834291,
4.38741669750802));
#20804=CARTESIAN_POINT('Ctrl Pts',(-26.5130256132123,-92.4398320992502,
4.41514087043794));
#20805=CARTESIAN_POINT('Ctrl Pts',(-26.4029696961734,-92.8802795945302,
4.44286504336787));
#20806=CARTESIAN_POINT('Ctrl Pts',(-26.185055515175,-93.2586003180438,4.47058921629779));
#20807=CARTESIAN_POINT('Ctrl Pts',(-25.7711354780326,-93.9772067309494,
4.52325027138067));
#20808=CARTESIAN_POINT('Ctrl Pts',(-24.9680669596902,-94.4716621331935,
4.57591132646355));
#20809=CARTESIAN_POINT('Ctrl Pts',(-24.140055238289,-94.5177225612861,4.62857238154642));
#20810=CARTESIAN_POINT('Ctrl Pts',(-23.3120435168878,-94.5637829893786,
4.6812334366293));
#20811=CARTESIAN_POINT('Ctrl Pts',(-22.4590885924278,-94.1614484433196,
4.73389449171218));
#20812=CARTESIAN_POINT('Ctrl Pts',(-21.968020079816,-93.493184506096,4.78655554679506));
#20813=CARTESIAN_POINT('Ctrl Pts',(-21.4769515672042,-92.8249205688725,
4.83921660187794));
#20814=CARTESIAN_POINT('Ctrl Pts',(-21.3477694664407,-91.8907272404844,
4.89187765696082));
#20815=CARTESIAN_POINT('Ctrl Pts',(-21.6390600648163,-91.1142771383271,
4.94453871204369));
#20816=CARTESIAN_POINT('Ctrl Pts',(-21.9303506631919,-90.3378270361698,
4.99719976712657));
#20817=CARTESIAN_POINT('Ctrl Pts',(-22.6421139607067,-89.7191201602431,
5.04986082220945));
#20818=CARTESIAN_POINT('Ctrl Pts',(-23.4515531549517,-89.5387506376962,
5.10252187729233));
#20819=CARTESIAN_POINT('Ctrl Pts',(-24.2609923491968,-89.3583811151493,
5.15518293237521));
#20820=CARTESIAN_POINT('Ctrl Pts',(-25.1681074401721,-89.6163489459821,
5.20784398745809));
#20821=CARTESIAN_POINT('Ctrl Pts',(-25.7615062532208,-90.1956613164022,
5.26050504254096));
#20822=CARTESIAN_POINT('Ctrl Pts',(-26.2381977114593,-90.6610367983859,
5.30280892752998));
#20823=CARTESIAN_POINT('Ctrl Pts',(-26.5124388592754,-91.3337853316565,
5.345112812519));
#20824=CARTESIAN_POINT('Ctrl Pts',(-26.5184743499735,-92.0021560918536,
5.38741669750802));
#20825=CARTESIAN_POINT('Origin',(-24.,-92.,5.));
#20826=CARTESIAN_POINT('',(-26.5199606688991,-91.9982645762516,6.38741669750802));
#20827=CARTESIAN_POINT('',(-26.5147663248015,-91.9983410423439,6.11258330249198));
#20828=CARTESIAN_POINT('',(-26.5175,-92.,5.));
#20829=CARTESIAN_POINT('Ctrl Pts',(-26.5147663248015,-91.9983410423439,
6.11258330249198));
#20830=CARTESIAN_POINT('Ctrl Pts',(-26.5166143414574,-91.6963819206475,
6.09354263098009));
#20831=CARTESIAN_POINT('Ctrl Pts',(-26.4662620027174,-91.3950183934935,
6.07450195946819));
#20832=CARTESIAN_POINT('Ctrl Pts',(-26.3609399824778,-91.1142771205843,
6.0554612879563));
#20833=CARTESIAN_POINT('Ctrl Pts',(-26.0696493782671,-90.3378270028732,
6.00280023287342));
#20834=CARTESIAN_POINT('Ctrl Pts',(-25.3578860664943,-89.7191201145527,
5.95013917779054));
#20835=CARTESIAN_POINT('Ctrl Pts',(-24.5484468560347,-89.5387505883926,
5.89747812270766));
#20836=CARTESIAN_POINT('Ctrl Pts',(-23.739007645575,-89.3583810622326,5.84481706762479));
#20837=CARTESIAN_POINT('Ctrl Pts',(-22.8318925364284,-89.616348898233,5.79215601254191));
#20838=CARTESIAN_POINT('Ctrl Pts',(-22.2384937114928,-90.1956612802579,
5.73949495745903));
#20839=CARTESIAN_POINT('Ctrl Pts',(-21.6450948865572,-90.7749736622827,
5.68683390237615));
#20840=CARTESIAN_POINT('Ctrl Pts',(-21.3654123458325,-91.6756305903319,
5.63417284729328));
#20841=CARTESIAN_POINT('Ctrl Pts',(-21.5262868946164,-92.4891687768701,
5.5815117922104));
#20842=CARTESIAN_POINT('Ctrl Pts',(-21.6871614434003,-93.3027069634083,
5.52885073712752));
#20843=CARTESIAN_POINT('Ctrl Pts',(-22.2885930816928,-94.0291264084354,
5.47618968204464));
#20844=CARTESIAN_POINT('Ctrl Pts',(-23.0578222974529,-94.3389834964905,
5.42352862696176));
#20845=CARTESIAN_POINT('Ctrl Pts',(-23.8270515132129,-94.6488405845455,
5.37086757187888));
#20846=CARTESIAN_POINT('Ctrl Pts',(-24.7640783064405,-94.5421353156285,
5.318206516796));
#20847=CARTESIAN_POINT('Ctrl Pts',(-25.4439450350434,-94.0672603502598,
5.26554546171313));
#20848=CARTESIAN_POINT('Ctrl Pts',(-26.1022043035296,-93.6074778161617,
5.21455807530608));
#20849=CARTESIAN_POINT('Ctrl Pts',(-26.5193898264469,-92.8025559702575,
5.16357068889903));
#20850=CARTESIAN_POINT('Ctrl Pts',(-26.5215003759084,-91.9995222402991,
5.11258330249198));
#20851=CARTESIAN_POINT('Ctrl Pts',(-26.5184743499735,-92.0021560918536,
5.38741669750802));
#20852=CARTESIAN_POINT('Ctrl Pts',(-26.5199520063112,-92.1657918820634,
5.39777386760188));
#20853=CARTESIAN_POINT('Ctrl Pts',(-26.5053532314693,-92.3291652655503,
5.40813103769574));
#20854=CARTESIAN_POINT('Ctrl Pts',(-26.4737130558304,-92.4891687670711,
5.4184882077896));
#20855=CARTESIAN_POINT('Ctrl Pts',(-26.3128385102691,-93.3027069373125,
5.47114926287248));
#20856=CARTESIAN_POINT('Ctrl Pts',(-25.7114068840244,-94.0291263677881,
5.52381031795536));
#20857=CARTESIAN_POINT('Ctrl Pts',(-24.9421776836735,-94.3389834496361,
5.57647137303823));
#20858=CARTESIAN_POINT('Ctrl Pts',(-24.1729484833226,-94.6488405314842,
5.62913242812111));
#20859=CARTESIAN_POINT('Ctrl Pts',(-23.2359217088655,-94.5421352647047,
5.68179348320399));
#20860=CARTESIAN_POINT('Ctrl Pts',(-22.5560549938817,-94.0672603088487,
5.73445453828687));
#20861=CARTESIAN_POINT('Ctrl Pts',(-21.8761882788978,-93.5923853529927,
5.78711559336975));
#20862=CARTESIAN_POINT('Ctrl Pts',(-21.4534816233873,-92.7493407080601,
5.83977664845262));
#20863=CARTESIAN_POINT('Ctrl Pts',(-21.479639709574,-91.9204615079354,5.8924377035355));
#20864=CARTESIAN_POINT('Ctrl Pts',(-21.5057977957607,-91.0915823078107,
5.94509875861838));
#20865=CARTESIAN_POINT('Ctrl Pts',(-21.9808206236446,-90.276868552494,5.99775981370126));
#20866=CARTESIAN_POINT('Ctrl Pts',(-22.6892772339901,-89.8458068340921,
6.05042086878414));
#20867=CARTESIAN_POINT('Ctrl Pts',(-23.3977338443356,-89.4147451156901,
6.10308192386701));
#20868=CARTESIAN_POINT('Ctrl Pts',(-24.3396242371427,-89.3673354342031,
6.15574297894989));
#20869=CARTESIAN_POINT('Ctrl Pts',(-25.0877850449385,-89.7250788890635,
6.20840403403277));
#20870=CARTESIAN_POINT('Ctrl Pts',(-25.8359458527343,-90.0828223439238,
6.26106508911565));
#20871=CARTESIAN_POINT('Ctrl Pts',(-26.3903770755186,-90.8457189351315,
6.31372614419853));
#20872=CARTESIAN_POINT('Ctrl Pts',(-26.499634691726,-91.6677820393728,6.36638719928141));
#20873=CARTESIAN_POINT('Ctrl Pts',(-26.5141782213651,-91.7772087277519,
6.37339703202361));
#20874=CARTESIAN_POINT('Ctrl Pts',(-26.5208337745228,-91.8876837803117,
6.38040686476582));
#20875=CARTESIAN_POINT('Ctrl Pts',(-26.5199606688991,-91.9982645762516,
6.38741669750802));
#20876=CARTESIAN_POINT('Origin',(-24.,-92.,5.));
#20877=CARTESIAN_POINT('',(-26.5136290410546,-91.9995053986546,7.38741669750802));
#20878=CARTESIAN_POINT('',(-26.5157926212741,-92.0020516723221,7.11258330249198));
#20879=CARTESIAN_POINT('',(-26.5175,-92.,5.));
#20880=CARTESIAN_POINT('Ctrl Pts',(-26.5157926212741,-92.0020516723221,
7.11258330249198));
#20881=CARTESIAN_POINT('Ctrl Pts',(-26.5112988583661,-91.4252696399995,
7.07617562814402));
#20882=CARTESIAN_POINT('Ctrl Pts',(-26.3140599311548,-90.8457098245431,
7.03976795379607));
#20883=CARTESIAN_POINT('Ctrl Pts',(-25.9507614766046,-90.4021663794855,
7.00336027944811));
#20884=CARTESIAN_POINT('Ctrl Pts',(-25.4252766641513,-89.760613019922,6.95069922436523));
#20885=CARTESIAN_POINT('Ctrl Pts',(-24.5523700775015,-89.4036265833224,
6.89803816928235));
#20886=CARTESIAN_POINT('Ctrl Pts',(-23.7279197494918,-89.4931065124105,
6.84537711419947));
#20887=CARTESIAN_POINT('Ctrl Pts',(-22.9034694214822,-89.5825864414987,
6.79271605911659));
#20888=CARTESIAN_POINT('Ctrl Pts',(-22.1274753521126,-90.1185327362745,
6.74005500403372));
#20889=CARTESIAN_POINT('Ctrl Pts',(-21.7518640956471,-90.8578846048887,
6.68739394895084));
#20890=CARTESIAN_POINT('Ctrl Pts',(-21.3762528391816,-91.5972364735028,
6.63473289386796));
#20891=CARTESIAN_POINT('Ctrl Pts',(-21.4010243956202,-92.5399939159553,
6.58207183878508));
#20892=CARTESIAN_POINT('Ctrl Pts',(-21.8149444410541,-93.258600343256,6.5294107837022));
#20893=CARTESIAN_POINT('Ctrl Pts',(-22.2288644864881,-93.9772067705567,
6.47674972861932));
#20894=CARTESIAN_POINT('Ctrl Pts',(-23.0319330209176,-94.4716621827056,
6.42408867353644));
#20895=CARTESIAN_POINT('Ctrl Pts',(-23.8599447589054,-94.5177226117208,
6.37142761845357));
#20896=CARTESIAN_POINT('Ctrl Pts',(-24.6879564968933,-94.563783040736,6.31876656337069));
#20897=CARTESIAN_POINT('Ctrl Pts',(-25.5409114384397,-94.1614484866175,
6.26610550828781));
#20898=CARTESIAN_POINT('Ctrl Pts',(-26.0319799608885,-93.4931845360073,
6.21344445320493));
#20899=CARTESIAN_POINT('Ctrl Pts',(-26.3454927087509,-93.0665449574646,
6.17982406963395));
#20900=CARTESIAN_POINT('Ctrl Pts',(-26.5115032555984,-92.531514543491,6.14620368606296));
#20901=CARTESIAN_POINT('Ctrl Pts',(-26.5147663248015,-91.9983410423439,
6.11258330249198));
#20902=CARTESIAN_POINT('Ctrl Pts',(-26.5199606688991,-91.9982645762516,
6.38741669750802));
#20903=CARTESIAN_POINT('Ctrl Pts',(-26.5142746075592,-92.7184170660063,
6.43306791984869));
#20904=CARTESIAN_POINT('Ctrl Pts',(-26.1892825133498,-93.4430543518201,
6.47871914218937));
#20905=CARTESIAN_POINT('Ctrl Pts',(-25.6442303551587,-93.9118182197226,
6.52437036453004));
#20906=CARTESIAN_POINT('Ctrl Pts',(-25.0154843927538,-94.4525616785562,
6.57703141961292));
#20907=CARTESIAN_POINT('Ctrl Pts',(-24.0939084583138,-94.6528189789487,
6.6296924746958));
#20908=CARTESIAN_POINT('Ctrl Pts',(-23.2974529654966,-94.4217700194304,
6.68235352977868));
#20909=CARTESIAN_POINT('Ctrl Pts',(-22.5009974726793,-94.1907210599122,
6.73501458486155));
#20910=CARTESIAN_POINT('Ctrl Pts',(-21.8296624214848,-93.5283658404832,
6.78767563994443));
#20911=CARTESIAN_POINT('Ctrl Pts',(-21.5879097152778,-92.7350937531496,
6.84033669502731));
#20912=CARTESIAN_POINT('Ctrl Pts',(-21.3461570090709,-91.941821665816,6.89299775011018));
#20913=CARTESIAN_POINT('Ctrl Pts',(-21.5339866478515,-91.0176327105778,
6.94565880519306));
#20914=CARTESIAN_POINT('Ctrl Pts',(-22.0662146837015,-90.381662358685,6.99831986027594));
#20915=CARTESIAN_POINT('Ctrl Pts',(-22.5984427195515,-89.7456920067921,
7.05098091535882));
#20916=CARTESIAN_POINT('Ctrl Pts',(-23.4750691524708,-89.3979402582445,
7.1036419704417));
#20917=CARTESIAN_POINT('Ctrl Pts',(-24.2985289370467,-89.4961184498875,
7.15630302552458));
#20918=CARTESIAN_POINT('Ctrl Pts',(-25.1219887216225,-89.5942966415305,
7.20896408060745));
#20919=CARTESIAN_POINT('Ctrl Pts',(-25.8922818578547,-90.1384047733641,
7.26162513569033));
#20920=CARTESIAN_POINT('Ctrl Pts',(-26.2600672575076,-90.8816805542397,
7.31428619077321));
#20921=CARTESIAN_POINT('Ctrl Pts',(-26.4303153507392,-91.2257433815264,
7.33866302635148));
#20922=CARTESIAN_POINT('Ctrl Pts',(-26.5143152963871,-91.6124832538171,
7.36303986192975));
#20923=CARTESIAN_POINT('Ctrl Pts',(-26.5136290410546,-91.9995053986546,
7.38741669750802));
#20924=CARTESIAN_POINT('Origin',(-24.,-92.,5.));
#20925=CARTESIAN_POINT('',(-26.5182106813093,-92.0021944371302,8.38741669750803));
#20926=CARTESIAN_POINT('',(-26.5215633824187,-91.9996804087644,8.11258330249198));
#20927=CARTESIAN_POINT('',(-26.5175,-92.,5.));
#20928=CARTESIAN_POINT('Ctrl Pts',(-26.5215633824187,-91.9996804087644,
8.11258330249198));
#20929=CARTESIAN_POINT('Ctrl Pts',(-26.5215950065109,-91.9821424208031,
8.11146968039083));
#20930=CARTESIAN_POINT('Ctrl Pts',(-26.5214276959298,-91.9646050519462,
8.11035605828969));
#20931=CARTESIAN_POINT('Ctrl Pts',(-26.5210595996876,-91.9470718985316,
8.10924243618854));
#20932=CARTESIAN_POINT('Ctrl Pts',(-26.5036530337928,-91.1179626730645,
8.05658138110567));
#20933=CARTESIAN_POINT('Ctrl Pts',(-26.0372570305162,-90.2982798630938,
8.00392032602279));
#20934=CARTESIAN_POINT('Ctrl Pts',(-25.333390328936,-89.8597634086715,7.95125927093992));
#20935=CARTESIAN_POINT('Ctrl Pts',(-24.6295236273558,-89.4212469542493,
7.89859821585704));
#20936=CARTESIAN_POINT('Ctrl Pts',(-23.688186227472,-89.3638968553754,7.84593716077416));
#20937=CARTESIAN_POINT('Ctrl Pts',(-22.9362906110337,-89.7137224600414,
7.79327610569128));
#20938=CARTESIAN_POINT('Ctrl Pts',(-22.1843949945955,-90.0635480647073,
7.7406150506084));
#20939=CARTESIAN_POINT('Ctrl Pts',(-21.6219411616028,-90.8205493729132,
7.68795399552552));
#20940=CARTESIAN_POINT('Ctrl Pts',(-21.5040115702347,-91.6414133236746,
7.63529294044264));
#20941=CARTESIAN_POINT('Ctrl Pts',(-21.3860819788666,-92.462277274436,7.58263188535977));
#20942=CARTESIAN_POINT('Ctrl Pts',(-21.7126766291231,-93.347003867753,7.52997083027689));
#20943=CARTESIAN_POINT('Ctrl Pts',(-22.3356792508831,-93.8943545185808,
7.47730977519401));
#20944=CARTESIAN_POINT('Ctrl Pts',(-22.9586818726432,-94.4417051694086,
7.42464872011113));
#20945=CARTESIAN_POINT('Ctrl Pts',(-23.8780924659067,-94.6516798777473,
7.37198766502825));
#20946=CARTESIAN_POINT('Ctrl Pts',(-24.6769426469386,-94.429051518253,7.31932660994537));
#20947=CARTESIAN_POINT('Ctrl Pts',(-25.4757928279705,-94.2064231587587,
7.2666655548625));
#20948=CARTESIAN_POINT('Ctrl Pts',(-26.1540825967709,-93.5511917314314,
7.21400449977962));
#20949=CARTESIAN_POINT('Ctrl Pts',(-26.4041959620427,-92.760515876504,7.16134344469674));
#20950=CARTESIAN_POINT('Ctrl Pts',(-26.4813912963606,-92.516480589178,7.14509006396182));
#20951=CARTESIAN_POINT('Ctrl Pts',(-26.5177987598365,-92.25954293317,7.1288366832269));
#20952=CARTESIAN_POINT('Ctrl Pts',(-26.5157926212741,-92.0020516723221,
7.11258330249198));
#20953=CARTESIAN_POINT('Ctrl Pts',(-26.5136290410546,-91.9995053986546,
7.38741669750802));
#20954=CARTESIAN_POINT('Ctrl Pts',(-26.5128327852651,-92.4485636557274,
7.41570091701263));
#20955=CARTESIAN_POINT('Ctrl Pts',(-26.3980256245316,-92.8980019292389,
7.44398513651724));
#20956=CARTESIAN_POINT('Ctrl Pts',(-26.1716474294659,-93.2815965984927,
7.47226935602185));
#20957=CARTESIAN_POINT('Ctrl Pts',(-25.7501645386979,-93.9957934319524,
7.52493041110472));
#20958=CARTESIAN_POINT('Ctrl Pts',(-24.9419210940886,-94.4817436689544,
7.5775914661876));
#20959=CARTESIAN_POINT('Ctrl Pts',(-24.1134692701342,-94.5190607190089,
7.63025252127048));
#20960=CARTESIAN_POINT('Ctrl Pts',(-23.2850174461799,-94.5563777690633,
7.68291357635336));
#20961=CARTESIAN_POINT('Ctrl Pts',(-22.4363572428804,-94.1450616321701,
7.73557463143624));
#20962=CARTESIAN_POINT('Ctrl Pts',(-21.9523705889737,-93.4716509197329,
7.78823568651911));
#20963=CARTESIAN_POINT('Ctrl Pts',(-21.468383935067,-92.7982402072957,7.840896741602));
#20964=CARTESIAN_POINT('Ctrl Pts',(-21.3490708305531,-91.8627349193144,
7.89355779668488));
#20965=CARTESIAN_POINT('Ctrl Pts',(-21.6485417162138,-91.0894032334354,
7.94621885176776));
#20966=CARTESIAN_POINT('Ctrl Pts',(-21.9480126018744,-90.3160715475563,
7.99887990685063));
#20967=CARTESIAN_POINT('Ctrl Pts',(-22.6662674777097,-89.7049134637794,
8.05154096193351));
#20968=CARTESIAN_POINT('Ctrl Pts',(-23.4775656801192,-89.5330984509984,
8.10420201701639));
#20969=CARTESIAN_POINT('Ctrl Pts',(-24.2888638825287,-89.3612834382173,
8.15686307209926));
#20970=CARTESIAN_POINT('Ctrl Pts',(-25.1932054115124,-89.628811496432,8.20952412718214));
#20971=CARTESIAN_POINT('Ctrl Pts',(-25.7804555817247,-90.2143564386821,
8.26218518226502));
#20972=CARTESIAN_POINT('Ctrl Pts',(-26.2459623243365,-90.6785114658679,
8.30392902067935));
#20973=CARTESIAN_POINT('Ctrl Pts',(-26.5122228629259,-91.3424942562717,
8.34567285909369));
#20974=CARTESIAN_POINT('Ctrl Pts',(-26.5182106813093,-92.0021944371302,
8.38741669750803));
#20975=CARTESIAN_POINT('Origin',(-24.,-92.,5.));
#20976=CARTESIAN_POINT('',(-26.5201759878003,-91.9984131478585,9.38741669750802));
#20977=CARTESIAN_POINT('',(-26.5149492652116,-91.9982505980886,9.11258330249198));
#20978=CARTESIAN_POINT('',(-26.5175,-92.,5.));
#20979=CARTESIAN_POINT('',(-22.0865340033349,-90.364012796625,10.));
#20980=CARTESIAN_POINT('Ctrl Pts',(-26.5201759878003,-91.9984131478585,
9.38741669750802));
#20981=CARTESIAN_POINT('Ctrl Pts',(-26.5146936217042,-92.7270926513296,
9.43362796642338));
#20982=CARTESIAN_POINT('Ctrl Pts',(-26.180732565303,-93.4600317456745,9.47983923533874));
#20983=CARTESIAN_POINT('Ctrl Pts',(-25.6239879633605,-93.9288767806186,
9.5260505042541));
#20984=CARTESIAN_POINT('Ctrl Pts',(-24.9895375611504,-94.4631593223022,
9.57871155933697));
#20985=CARTESIAN_POINT('Ctrl Pts',(-24.0657751669118,-94.6544830596338,
9.63137261441985));
#20986=CARTESIAN_POINT('Ctrl Pts',(-23.2718706971314,-94.4146105241972,
9.68403366950273));
#20987=CARTESIAN_POINT('Ctrl Pts',(-22.4779662273509,-94.1747379887606,
9.73669472458561));
#20988=CARTESIAN_POINT('Ctrl Pts',(-21.8139196820286,-93.5036691805557,
9.78935577966849));
#20989=CARTESIAN_POINT('Ctrl Pts',(-21.5807331050278,-92.7092693915533,
9.84201683475137));
#20990=CARTESIAN_POINT('Ctrl Pts',(-21.347546528027,-91.9148696025508,9.89467788983425));
#20991=CARTESIAN_POINT('Ctrl Pts',(-21.5452199193478,-90.9971388327508,
9.94733894491712));
#20992=CARTESIAN_POINT('Ctrl Pts',(-22.0865340033349,-90.364012796625,10.));
#20993=CARTESIAN_POINT('',(-25.9171033105362,-90.3614656677959,10.));
#20994=CARTESIAN_POINT('Origin',(-24.,-92.,10.));
#20995=CARTESIAN_POINT('Ctrl Pts',(-25.9171117712833,-90.3614597429255,
10.));
#20996=CARTESIAN_POINT('Ctrl Pts',(-25.3939570615584,-89.7523041616072,
9.94901908464118));
#20997=CARTESIAN_POINT('Ctrl Pts',(-24.5534187329285,-89.4121722649682,
9.89803816928235));
#20998=CARTESIAN_POINT('Ctrl Pts',(-23.7542642249036,-89.4905146133597,
9.84705725392353));
#20999=CARTESIAN_POINT('Ctrl Pts',(-22.9287725821855,-89.5714388316664,
9.79439619884065));
#21000=CARTESIAN_POINT('Ctrl Pts',(-22.1474374185984,-90.0988744884397,
9.74173514375777));
#21001=CARTESIAN_POINT('Ctrl Pts',(-21.7641119401365,-90.8341462635555,
9.68907408867489));
#21002=CARTESIAN_POINT('Ctrl Pts',(-21.3807864616747,-91.5694180386713,
9.63641303359202));
#21003=CARTESIAN_POINT('Ctrl Pts',(-21.3954706683382,-92.5125259321295,
9.58375197850914));
#21004=CARTESIAN_POINT('Ctrl Pts',(-21.8017475811356,-93.2354979451803,
9.53109092342626));
#21005=CARTESIAN_POINT('Ctrl Pts',(-22.2080244939329,-93.9584699582311,
9.47842986834338));
#21006=CARTESIAN_POINT('Ctrl Pts',(-23.0058941128643,-94.4613060908746,
9.4257688132605));
#21007=CARTESIAN_POINT('Ctrl Pts',(-23.8333901989263,-94.5160871276519,
9.37310775817762));
#21008=CARTESIAN_POINT('Ctrl Pts',(-24.6608862849884,-94.5708681644292,
9.32044670309475));
#21009=CARTESIAN_POINT('Ctrl Pts',(-25.5180088381812,-94.1775941053403,
9.26778564801187));
#21010=CARTESIAN_POINT('Ctrl Pts',(-26.0160962955285,-93.5145599775471,
9.21512459292899));
#21011=CARTESIAN_POINT('Ctrl Pts',(-26.339387264832,-93.0842079526292,9.18094416278332));
#21012=CARTESIAN_POINT('Ctrl Pts',(-26.5114221549398,-92.5402100730638,
9.14676373263765));
#21013=CARTESIAN_POINT('Ctrl Pts',(-26.5149492652116,-91.9982505980886,
9.11258330249198));
#21014=CARTESIAN_POINT('Origin',(-24.,-92.,12.2084234471775));
#21015=CARTESIAN_POINT('',(-27.0782768196867,-91.9992118911386,1.79157655282254));
#21016=CARTESIAN_POINT('',(-27.0686110023456,-91.9996651237392,1.70842344717745));
#21017=CARTESIAN_POINT('',(-27.0735,-91.9999999999999,12.2084234471775));
#21018=CARTESIAN_POINT('',(-23.2062007174672,-94.9692229537457,0.999999999999999));
#21019=CARTESIAN_POINT('Ctrl Pts',(-27.0686110023456,-91.9996651237392,
1.70842344717745));
#21020=CARTESIAN_POINT('Ctrl Pts',(-27.0689534453578,-91.5053846687106,
1.68292651844981));
#21021=CARTESIAN_POINT('Ctrl Pts',(-26.7235567931003,-89.9907712706007,
1.6047685346393));
#21022=CARTESIAN_POINT('Ctrl Pts',(-24.3539161166825,-88.3911596148569,
1.4739494957459));
#21023=CARTESIAN_POINT('Ctrl Pts',(-21.1687759971456,-89.7301450507159,
1.31596633049727));
#21024=CARTESIAN_POINT('Ctrl Pts',(-20.5566856051374,-93.1332975040884,
1.15798316524863));
#21025=CARTESIAN_POINT('Ctrl Pts',(-22.2237466982397,-94.7065713079336,
1.05266105508288));
#21026=CARTESIAN_POINT('Ctrl Pts',(-23.2062007174672,-94.9692229537457,
0.999999999999999));
#21027=CARTESIAN_POINT('',(-24.7937992825329,-94.9692229537457,0.999999999999999));
#21028=CARTESIAN_POINT('Origin',(-24.,-92.,0.999999999999999));
#21029=CARTESIAN_POINT('Ctrl Pts',(-27.0782768196867,-91.9992118911386,
1.79157655282254));
#21030=CARTESIAN_POINT('Ctrl Pts',(-27.0784229132411,-91.9562584982139,
1.78934283757203));
#21031=CARTESIAN_POINT('Ctrl Pts',(-27.058222313234,-90.9007975699364,1.73444806723864));
#21032=CARTESIAN_POINT('Ctrl Pts',(-25.852395087606,-88.8820465732967,1.62689224182237));
#21033=CARTESIAN_POINT('Ctrl Pts',(-22.4009681396119,-88.7444872144855,
1.46890907657374));
#21034=CARTESIAN_POINT('Ctrl Pts',(-20.4000491745082,-91.5606286501729,
1.3109259113251));
#21035=CARTESIAN_POINT('Ctrl Pts',(-21.6506964041098,-94.7394102869818,
1.15462288580052));
#21036=CARTESIAN_POINT('Ctrl Pts',(-23.8480946426715,-95.2254055619768,
1.05098091535882));
#21037=CARTESIAN_POINT('Ctrl Pts',(-24.7957017813267,-94.9743128096467,
1.));
#21038=CARTESIAN_POINT('Origin',(-24.,-92.,12.2084234471775));
#21039=CARTESIAN_POINT('',(-27.0699491247542,-91.9980972118633,2.79157655282254));
#21040=CARTESIAN_POINT('',(-27.075008445109,-92.0025755322285,2.70842344717745));
#21041=CARTESIAN_POINT('',(-27.0735,-91.9999999999999,12.2084234471775));
#21042=CARTESIAN_POINT('Ctrl Pts',(-27.075008445109,-92.0025755322285,2.70842344717745));
#21043=CARTESIAN_POINT('Ctrl Pts',(-27.0676143896354,-91.1760102841626,
2.66555951561375));
#21044=CARTESIAN_POINT('Ctrl Pts',(-26.2993641383815,-89.3218328468575,
2.57003452896717));
#21045=CARTESIAN_POINT('Ctrl Pts',(-23.1738621865499,-88.4685620798055,
2.42184848723771));
#21046=CARTESIAN_POINT('Ctrl Pts',(-20.5910234496019,-90.7619776832305,
2.26386532198907));
#21047=CARTESIAN_POINT('Ctrl Pts',(-21.1003113510007,-94.1783942746989,
2.10588215674044));
#21048=CARTESIAN_POINT('Ctrl Pts',(-24.2395758256157,-95.6187848570707,
1.94789899149181));
#21049=CARTESIAN_POINT('Ctrl Pts',(-26.690200871183,-94.074343589762,1.81541275497081));
#21050=CARTESIAN_POINT('Ctrl Pts',(-27.0682461676098,-92.5262656754663,
1.73558757353269));
#21051=CARTESIAN_POINT('Ctrl Pts',(-27.0686110023456,-91.9996651237392,
1.70842344717745));
#21052=CARTESIAN_POINT('Ctrl Pts',(-27.0699491247542,-91.9980972118633,
2.79157655282254));
#21053=CARTESIAN_POINT('Ctrl Pts',(-27.0721211881235,-91.6185397169383,
2.77197583473597));
#21054=CARTESIAN_POINT('Ctrl Pts',(-26.8315580332634,-90.2218843885842,
2.69971406156651));
#21055=CARTESIAN_POINT('Ctrl Pts',(-24.7514083751606,-88.4518994955133,
2.57479123331418));
#21056=CARTESIAN_POINT('Ctrl Pts',(-21.4392013302128,-89.4317376344075,
2.41680806806554));
#21057=CARTESIAN_POINT('Ctrl Pts',(-20.4497278964894,-92.7410889661721,
2.25882490281691));
#21058=CARTESIAN_POINT('Ctrl Pts',(-22.6804687378898,-95.3782236865055,
2.10084173756827));
#21059=CARTESIAN_POINT('Ctrl Pts',(-26.0596142672113,-94.9572795305498,
1.94509228757015));
#21060=CARTESIAN_POINT('Ctrl Pts',(-27.0749786780307,-92.9689081590363,
1.84200389265491));
#21061=CARTESIAN_POINT('Ctrl Pts',(-27.0782768196867,-91.9992118911386,
1.79157655282254));
#21062=CARTESIAN_POINT('Origin',(-24.,-92.,12.2084234471775));
#21063=CARTESIAN_POINT('',(-27.0716998581066,-92.0025715694568,3.79157655282255));
#21064=CARTESIAN_POINT('',(-27.0762206925998,-91.9977671184427,3.70842344717745));
#21065=CARTESIAN_POINT('',(-27.0735,-91.9999999999999,12.2084234471775));
#21066=CARTESIAN_POINT('Ctrl Pts',(-27.0762206925998,-91.9977671184427,
3.70842344717745));
#21067=CARTESIAN_POINT('Ctrl Pts',(-27.0774154713987,-91.8519430387287,
3.70085356786056));
#21068=CARTESIAN_POINT('Ctrl Pts',(-27.0019701064919,-90.6929124367373,
3.6406226334608));
#21069=CARTESIAN_POINT('Ctrl Pts',(-25.5299146181504,-88.7116868408497,
3.52773064397815));
#21070=CARTESIAN_POINT('Ctrl Pts',(-22.0822080355935,-88.9217351333484,
3.36974747872952));
#21071=CARTESIAN_POINT('Ctrl Pts',(-20.3740037605626,-91.92387423856,3.21176431348088));
#21072=CARTESIAN_POINT('Ctrl Pts',(-21.9547027823836,-94.99506300667,3.05378114823225));
#21073=CARTESIAN_POINT('Ctrl Pts',(-25.3905542616683,-95.349625359661,2.89579798298362));
#21074=CARTESIAN_POINT('Ctrl Pts',(-26.9751245860296,-93.3940964065108,
2.78067874929868));
#21075=CARTESIAN_POINT('Ctrl Pts',(-27.076698455151,-92.1914980490519,2.71822057069663));
#21076=CARTESIAN_POINT('Ctrl Pts',(-27.075008445109,-92.0025755322285,2.70842344717745));
#21077=CARTESIAN_POINT('Ctrl Pts',(-27.0716998581066,-92.0025715694568,
3.79157655282254));
#21078=CARTESIAN_POINT('Ctrl Pts',(-27.0659415382079,-91.2877405601207,
3.7546088318999));
#21079=CARTESIAN_POINT('Ctrl Pts',(-26.4623934875611,-89.5458532246352,
3.66498005589438));
#21080=CARTESIAN_POINT('Ctrl Pts',(-23.5706310215098,-88.3987107062197,
3.52269022480598));
#21081=CARTESIAN_POINT('Ctrl Pts',(-20.7493845448822,-90.3915405493825,
3.36470705955735));
#21082=CARTESIAN_POINT('Ctrl Pts',(-20.876557261488,-93.8432981737925,3.20672389430871));
#21083=CARTESIAN_POINT('Ctrl Pts',(-23.8367991007265,-95.6231211133646,
3.04874072906008));
#21084=CARTESIAN_POINT('Ctrl Pts',(-26.5594316628929,-94.3035556341771,
2.91035828189802));
#21085=CARTESIAN_POINT('Ctrl Pts',(-27.0662855269897,-92.6382930779672,
2.82463688981884));
#21086=CARTESIAN_POINT('Ctrl Pts',(-27.0699491247542,-91.9980972118633,
2.79157655282254));
#21087=CARTESIAN_POINT('Origin',(-24.,-92.,12.2084234471775));
#21088=CARTESIAN_POINT('',(-27.0783838750167,-91.9994167251476,4.79157655282255));
#21089=CARTESIAN_POINT('',(-27.0687191146691,-91.9995675532748,4.70842344717746));
#21090=CARTESIAN_POINT('',(-27.0735,-91.9999999999999,12.2084234471775));
#21091=CARTESIAN_POINT('Ctrl Pts',(-27.0687191146691,-91.9995675532748,
4.70842344717746));
#21092=CARTESIAN_POINT('Ctrl Pts',(-27.0693322679535,-91.5161929491144,
4.6834865650245));
#21093=CARTESIAN_POINT('Ctrl Pts',(-26.7346951702922,-90.0128432522753,
4.60588862778867));
#21094=CARTESIAN_POINT('Ctrl Pts',(-24.3913282785028,-88.3943788173915,
4.47562963546995));
#21095=CARTESIAN_POINT('Ctrl Pts',(-21.1942537915233,-89.7018637718047,
4.31764647022133));
#21096=CARTESIAN_POINT('Ctrl Pts',(-20.5420868753907,-93.0938367187666,
4.15966330497269));
#21097=CARTESIAN_POINT('Ctrl Pts',(-23.026365202284,-95.4936624405808,4.00168013972406));
#21098=CARTESIAN_POINT('Ctrl Pts',(-26.2324121355514,-94.7614664286128,
3.85126685379231));
#21099=CARTESIAN_POINT('Ctrl Pts',(-27.0691038049237,-92.8663911656747,
3.75351462294344));
#21100=CARTESIAN_POINT('Ctrl Pts',(-27.0762206925998,-91.9977671184427,
3.70842344717745));
#21101=CARTESIAN_POINT('Ctrl Pts',(-27.0783838750167,-91.9994167251476,
4.79157655282255));
#21102=CARTESIAN_POINT('Ctrl Pts',(-27.0784684546913,-91.9672353748387,
4.78990288414672));
#21103=CARTESIAN_POINT('Ctrl Pts',(-27.0634882463523,-90.9225663485135,
4.73556816038801));
#21104=CARTESIAN_POINT('Ctrl Pts',(-25.8851897703268,-88.9016614152428,
4.62857238154642));
#21105=CARTESIAN_POINT('Ctrl Pts',(-22.435457678629,-88.7280205108105,4.4705892162978));
#21106=CARTESIAN_POINT('Ctrl Pts',(-20.4048188734298,-91.5221766816716,
4.31260605104916));
#21107=CARTESIAN_POINT('Ctrl Pts',(-21.6351320616123,-94.7497349135865,
4.15462288580052));
#21108=CARTESIAN_POINT('Ctrl Pts',(-25.0104611872221,-95.4831897200468,
3.99663972055189));
#21109=CARTESIAN_POINT('Ctrl Pts',(-26.8939121321552,-93.6249319667866,
3.8756242762259));
#21110=CARTESIAN_POINT('Ctrl Pts',(-27.0741443484921,-92.3060277095063,
3.80726988698278));
#21111=CARTESIAN_POINT('Ctrl Pts',(-27.0716998581066,-92.0025715694568,
3.79157655282254));
#21112=CARTESIAN_POINT('Origin',(-24.,-92.,12.2084234471775));
#21113=CARTESIAN_POINT('',(-27.0701625816395,-91.9979746548734,5.79157655282255));
#21114=CARTESIAN_POINT('',(-27.0746895390839,-92.0026322734109,5.70842344717746));
#21115=CARTESIAN_POINT('',(-27.0735,-91.9999999999999,12.2084234471775));
#21116=CARTESIAN_POINT('Ctrl Pts',(-27.0746895390839,-92.0026322734109,
5.70842344717746));
#21117=CARTESIAN_POINT('Ctrl Pts',(-27.0673210859912,-91.1866491427393,
5.66611956218844));
#21118=CARTESIAN_POINT('Ctrl Pts',(-26.3157338396918,-89.3429097126816,
5.57115462211654));
#21119=CARTESIAN_POINT('Ctrl Pts',(-23.2111784520928,-88.4600278964635,
5.42352862696177));
#21120=CARTESIAN_POINT('Ctrl Pts',(-20.6043011989706,-90.7260802299217,
5.26554546171313));
#21121=CARTESIAN_POINT('Ctrl Pts',(-21.0774386607742,-94.1476212763577,
5.1075622964645));
#21122=CARTESIAN_POINT('Ctrl Pts',(-24.2014390107181,-95.6211965224102,
4.94957913121586));
#21123=CARTESIAN_POINT('Ctrl Pts',(-26.6784591036876,-94.0960763882476,
4.81653284812018));
#21124=CARTESIAN_POINT('Ctrl Pts',(-27.068037426895,-92.536970787307,4.73614762010738));
#21125=CARTESIAN_POINT('Ctrl Pts',(-27.0687191146691,-91.9995675532748,
4.70842344717746));
#21126=CARTESIAN_POINT('Ctrl Pts',(-27.0701625816395,-91.9979746548734,
5.79157655282255));
#21127=CARTESIAN_POINT('Ctrl Pts',(-27.0724187402063,-91.629326646717,5.77253588131066));
#21128=CARTESIAN_POINT('Ctrl Pts',(-26.8409295378372,-90.2438417959684,
5.70083415471588));
#21129=CARTESIAN_POINT('Ctrl Pts',(-24.7888215637087,-88.4600278255509,
5.57647137303823));
#21130=CARTESIAN_POINT('Ctrl Pts',(-21.4664561758692,-89.404851035816,5.41848820778961));
#21131=CARTESIAN_POINT('Ctrl Pts',(-20.4421015118168,-92.7035629345559,
5.26050504254096));
#21132=CARTESIAN_POINT('Ctrl Pts',(-22.6448822152433,-95.3641192375839,
5.10252187729233));
#21133=CARTESIAN_POINT('Ctrl Pts',(-26.040443362995,-94.9774448457586,4.94621238071952));
#21134=CARTESIAN_POINT('Ctrl Pts',(-27.0758072022183,-92.9798036840462,
4.8425639392296));
#21135=CARTESIAN_POINT('Ctrl Pts',(-27.0783838750167,-91.9994167251476,
4.79157655282255));
#21136=CARTESIAN_POINT('Origin',(-24.,-92.,12.2084234471775));
#21137=CARTESIAN_POINT('',(-27.0714155398157,-92.0025047924058,6.79157655282255));
#21138=CARTESIAN_POINT('',(-27.0765041175219,-91.9978813009372,6.70842344717745));
#21139=CARTESIAN_POINT('',(-27.0735,-91.9999999999999,12.2084234471775));
#21140=CARTESIAN_POINT('Ctrl Pts',(-27.0765041175218,-91.9978813009372,
6.70842344717745));
#21141=CARTESIAN_POINT('Ctrl Pts',(-27.077570052034,-91.8628782914749,6.70141361443525));
#21142=CARTESIAN_POINT('Ctrl Pts',(-27.0084024469269,-90.7147701434973,
6.64174272661016));
#21143=CARTESIAN_POINT('Ctrl Pts',(-25.5645422900302,-88.7280205763547,
6.52941078370221));
#21144=CARTESIAN_POINT('Ctrl Pts',(-22.114810267437,-88.9016614773084,6.37142761845357));
#21145=CARTESIAN_POINT('Ctrl Pts',(-20.3750096777634,-91.8856011718064,
6.21344445320494));
#21146=CARTESIAN_POINT('Ctrl Pts',(-21.923199039088,-94.9733045078939,6.0554612879563));
#21147=CARTESIAN_POINT('Ctrl Pts',(-25.3551177576112,-95.3641191701941,
5.89747812270767));
#21148=CARTESIAN_POINT('Ctrl Pts',(-26.9680496218174,-93.4159924088721,
5.78179884244805));
#21149=CARTESIAN_POINT('Ctrl Pts',(-27.0764935417666,-92.2024076860066,
5.71878061727132));
#21150=CARTESIAN_POINT('Ctrl Pts',(-27.0746895390839,-92.0026322734109,
5.70842344717746));
#21151=CARTESIAN_POINT('Ctrl Pts',(-27.0714155398157,-92.0025047924058,
6.79157655282255));
#21152=CARTESIAN_POINT('Ctrl Pts',(-27.0659293112961,-91.2983381285157,
6.75516887847459));
#21153=CARTESIAN_POINT('Ctrl Pts',(-26.4768297637755,-89.5673490693385,
6.66610014904375));
#21154=CARTESIAN_POINT('Ctrl Pts',(-23.6086717136575,-88.3943787451648,
6.52437036453005));
#21155=CARTESIAN_POINT('Ctrl Pts',(-20.7665452720997,-90.3573153135784,
6.36638719928141));
#21156=CARTESIAN_POINT('Ctrl Pts',(-20.8572726350159,-93.8102229593112,
6.20840403403277));
#21157=CARTESIAN_POINT('Ctrl Pts',(-23.7985609852469,-95.6211965949497,
6.05042086878414));
#21158=CARTESIAN_POINT('Ctrl Pts',(-26.5460461813277,-94.3252216524648,
5.9114783750474));
#21159=CARTESIAN_POINT('Ctrl Pts',(-27.0661788504793,-92.6489016680912,
5.82519693639353));
#21160=CARTESIAN_POINT('Ctrl Pts',(-27.0701625816395,-91.9979746548734,
5.79157655282255));
#21161=CARTESIAN_POINT('Origin',(-24.,-92.,12.2084234471775));
#21162=CARTESIAN_POINT('',(-27.0784607967681,-91.9996098257547,7.79157655282255));
#21163=CARTESIAN_POINT('',(-27.0687741242031,-91.9993961639582,7.70842344717745));
#21164=CARTESIAN_POINT('',(-27.0735,-91.9999999999999,12.2084234471775));
#21165=CARTESIAN_POINT('Ctrl Pts',(-27.0687741242031,-91.9993961639582,
7.70842344717745));
#21166=CARTESIAN_POINT('Ctrl Pts',(-27.0696119417858,-91.5268986218895,
7.68404661159918));
#21167=CARTESIAN_POINT('Ctrl Pts',(-26.7455188317855,-90.0347580376889,
7.60700872093803));
#21168=CARTESIAN_POINT('Ctrl Pts',(-24.4293689698895,-88.3987107783728,
7.47730977519402));
#21169=CARTESIAN_POINT('Ctrl Pts',(-21.2186702510283,-89.672373140829,7.31932660994537));
#21170=CARTESIAN_POINT('Ctrl Pts',(-20.5307325412461,-93.057272549676,7.16134344469675));
#21171=CARTESIAN_POINT('Ctrl Pts',(-22.9895388330194,-95.4831896502703,
7.0033602794481));
#21172=CARTESIAN_POINT('Ctrl Pts',(-26.2151019833044,-94.7822788033369,
6.85238694694168));
#21173=CARTESIAN_POINT('Ctrl Pts',(-27.0695622666666,-92.8770823643973,
6.75407466951813));
#21174=CARTESIAN_POINT('Ctrl Pts',(-27.0765041175218,-91.9978813009372,
6.70842344717745));
#21175=CARTESIAN_POINT('Ctrl Pts',(-27.0784607967681,-91.9996098257547,
7.79157655282255));
#21176=CARTESIAN_POINT('Ctrl Pts',(-27.0784994051683,-91.9781985026171,
7.7904629307214));
#21177=CARTESIAN_POINT('Ctrl Pts',(-27.0686359944836,-90.944323237583,7.73668825353738));
#21178=CARTESIAN_POINT('Ctrl Pts',(-25.9177920028682,-88.9217350716083,
7.63025252127049));
#21179=CARTESIAN_POINT('Ctrl Pts',(-22.4700853511787,-88.7116867750179,
7.47226935602185));
#21180=CARTESIAN_POINT('Ctrl Pts',(-20.4100632788413,-91.4842510500175,
7.31428619077321));
#21181=CARTESIAN_POINT('Ctrl Pts',(-21.6062364556795,-94.7246171090759,
7.15630302552459));
#21182=CARTESIAN_POINT('Ctrl Pts',(-24.9736348172233,-95.4936625105602,
6.99831986027594));
#21183=CARTESIAN_POINT('Ctrl Pts',(-26.8854041041607,-93.6468834845165,
6.87674436937527));
#21184=CARTESIAN_POINT('Ctrl Pts',(-27.073864742148,-92.3168640338026,6.80782993355747));
#21185=CARTESIAN_POINT('Ctrl Pts',(-27.0714155398157,-92.0025047924058,
6.79157655282255));
#21186=CARTESIAN_POINT('Origin',(-24.,-92.,12.2084234471775));
#21187=CARTESIAN_POINT('',(-27.0703859251749,-91.9978642356407,8.79157655282255));
#21188=CARTESIAN_POINT('',(-27.0743676381347,-92.0026790873961,8.70842344717746));
#21189=CARTESIAN_POINT('',(-27.0735,-91.9999999999999,12.2084234471775));
#21190=CARTESIAN_POINT('Ctrl Pts',(-27.0743676381347,-92.0026790873961,
8.70842344717746));
#21191=CARTESIAN_POINT('Ctrl Pts',(-27.0670573859793,-91.1972814683818,
8.66667960876313));
#21192=CARTESIAN_POINT('Ctrl Pts',(-26.3319129571347,-89.3640272738251,
8.57227471526591));
#21193=CARTESIAN_POINT('Ctrl Pts',(-23.2485916399684,-88.4518995672047,
8.42520876668582));
#21194=CARTESIAN_POINT('Ctrl Pts',(-20.6179385783441,-90.6903039808948,
8.26722560143718));
#21195=CARTESIAN_POINT('Ctrl Pts',(-21.0549302288588,-94.116650160768,8.10924243618856));
#21196=CARTESIAN_POINT('Ctrl Pts',(-24.1632008959979,-95.6231210406981,
7.95125927093991));
#21197=CARTESIAN_POINT('Ctrl Pts',(-26.6666767475757,-94.1179251847747,
7.81765294126956));
#21198=CARTESIAN_POINT('Ctrl Pts',(-27.0678020121201,-92.5476307431492,
7.73670766668206));
#21199=CARTESIAN_POINT('Ctrl Pts',(-27.0687741242031,-91.9993961639582,
7.70842344717745));
#21200=CARTESIAN_POINT('Ctrl Pts',(-27.0703859251749,-91.9978642356407,
8.79157655282255));
#21201=CARTESIAN_POINT('Ctrl Pts',(-27.0727141338614,-91.6401224413272,
8.77309592788534));
#21202=CARTESIAN_POINT('Ctrl Pts',(-26.8501668180301,-90.265785975548,8.70195424786525));
#21203=CARTESIAN_POINT('Ctrl Pts',(-24.8261378316183,-88.4685620052275,
8.57815151276229));
#21204=CARTESIAN_POINT('Ctrl Pts',(-21.493997396212,-89.3782456609066,8.42016834751366));
#21205=CARTESIAN_POINT('Ctrl Pts',(-20.4348704258473,-92.6659673604641,
8.26218518226503));
#21206=CARTESIAN_POINT('Ctrl Pts',(-22.6094457101907,-95.3496254273119,
8.10420201701638));
#21207=CARTESIAN_POINT('Ctrl Pts',(-26.0210779679428,-94.9975623737004,
7.94733247386889));
#21208=CARTESIAN_POINT('Ctrl Pts',(-27.0766736879126,-92.9906989423899,
7.84312398580428));
#21209=CARTESIAN_POINT('Ctrl Pts',(-27.0784607967681,-91.9996098257547,
7.79157655282255));
#21210=CARTESIAN_POINT('Origin',(-24.,-92.,12.2084234471775));
#21211=CARTESIAN_POINT('',(-27.0702887490762,-92.0031018432153,9.79157655282255));
#21212=CARTESIAN_POINT('',(-27.0767669904684,-91.998062685181,9.70842344717746));
#21213=CARTESIAN_POINT('',(-27.0735,-91.9999999999999,12.2084234471775));
#21214=CARTESIAN_POINT('',(-24.7937992825329,-94.9692229537457,10.));
#21215=CARTESIAN_POINT('Ctrl Pts',(-24.7937992825329,-94.9692229537457,
10.));
#21216=CARTESIAN_POINT('Ctrl Pts',(-25.7762533017603,-94.7065713079336,
9.94733894491712));
#21217=CARTESIAN_POINT('Ctrl Pts',(-26.875910333047,-93.6687793941585,9.87786446252463));
#21218=CARTESIAN_POINT('Ctrl Pts',(-27.0726354893275,-92.3283627763233,
9.80838998013215));
#21219=CARTESIAN_POINT('Ctrl Pts',(-27.0702887490762,-92.0031018432153,
9.79157655282255));
#21220=CARTESIAN_POINT('',(-23.2043026670138,-94.9743009685655,10.));
#21221=CARTESIAN_POINT('Origin',(-24.,-92.,10.));
#21222=CARTESIAN_POINT('Ctrl Pts',(-23.2042982523172,-94.9743127795766,
10.));
#21223=CARTESIAN_POINT('Ctrl Pts',(-24.1519054403103,-95.2254055803294,
9.94901908464118));
#21224=CARTESIAN_POINT('Ctrl Pts',(-26.2125562800898,-94.7696542914347,
9.851826900367));
#21225=CARTESIAN_POINT('Ctrl Pts',(-27.0700738217707,-92.8876739876312,
9.75463471609282));
#21226=CARTESIAN_POINT('Ctrl Pts',(-27.0767669904684,-91.998062685181,9.70842344717746));
#21227=CARTESIAN_POINT('Origin',(92.,-24.,5.));
#21228=CARTESIAN_POINT('',(89.486504426694,-23.9997257424662,1.38741669750802));
#21229=CARTESIAN_POINT('',(89.4843725317804,-24.0035302714347,1.11258330249198));
#21230=CARTESIAN_POINT('',(89.4825,-24.,5.));
#21231=CARTESIAN_POINT('',(90.086534003335,-22.364012796625,0.999999999999999));
#21232=CARTESIAN_POINT('Ctrl Pts',(89.4843725317804,-24.0035302714347,1.11258330249198));
#21233=CARTESIAN_POINT('Ctrl Pts',(89.4895356694446,-23.4109125587034,1.07505553499465));
#21234=CARTESIAN_POINT('Ctrl Pts',(89.7007781719159,-22.8151964396956,1.03752776749733));
#21235=CARTESIAN_POINT('Ctrl Pts',(90.0865340033349,-22.364012796625,0.999999999999998));
#21236=CARTESIAN_POINT('',(89.4825,-24.,1.));
#21237=CARTESIAN_POINT('Origin',(92.,-24.,1.));
#21238=CARTESIAN_POINT('',(89.4825,-24.,0.));
#21239=CARTESIAN_POINT('',(89.4825,-24.,5.));
#21240=CARTESIAN_POINT('Origin',(92.,-24.,0.));
#21241=CARTESIAN_POINT('',(93.9171033775211,-22.3614656597818,0.999999999999999));
#21242=CARTESIAN_POINT('Origin',(92.,-24.,1.));
#21243=CARTESIAN_POINT('Ctrl Pts',(93.9171118396844,-22.3614597340103,0.999999999999999));
#21244=CARTESIAN_POINT('Ctrl Pts',(93.39395715018,-21.7523042564146,1.05098091535882));
#21245=CARTESIAN_POINT('Ctrl Pts',(92.5534187715749,-21.4121721444715,1.10196183071765));
#21246=CARTESIAN_POINT('Ctrl Pts',(91.7542642221519,-21.4905144511518,1.15294274607647));
#21247=CARTESIAN_POINT('Ctrl Pts',(90.9287725366714,-21.5714386263726,1.20560380115935));
#21248=CARTESIAN_POINT('Ctrl Pts',(90.147437339474,-22.0988744252836,1.25826485624223));
#21249=CARTESIAN_POINT('Ctrl Pts',(89.7641118492187,-22.8341462554664,1.31092591132511));
#21250=CARTESIAN_POINT('Ctrl Pts',(89.578516959615,-23.190143176153,1.33642284005274));
#21251=CARTESIAN_POINT('Ctrl Pts',(89.4862239279038,-23.5948612398581,1.36191976878038));
#21252=CARTESIAN_POINT('Ctrl Pts',(89.486504426694,-23.9997257424662,1.38741669750802));
#21253=CARTESIAN_POINT('Origin',(92.,-24.,5.));
#21254=CARTESIAN_POINT('',(89.4812642899865,-24.0021096151709,2.38741669750802));
#21255=CARTESIAN_POINT('',(89.478587803344,-23.999354427872,2.11258330249198));
#21256=CARTESIAN_POINT('',(89.4825,-24.,5.));
#21257=CARTESIAN_POINT('Ctrl Pts',(89.478587803344,-23.999354427872,2.11258330249198));
#21258=CARTESIAN_POINT('Ctrl Pts',(89.478468138627,-23.9641713652006,2.11034958724147));
#21259=CARTESIAN_POINT('Ctrl Pts',(89.4791414214072,-23.928993039682,2.10811587199095));
#21260=CARTESIAN_POINT('Ctrl Pts',(89.4806219723461,-23.8938487862731,2.10588215674044));
#21261=CARTESIAN_POINT('Ctrl Pts',(89.5155267680806,-23.0653038478858,2.05322110165756));
#21262=CARTESIAN_POINT('Ctrl Pts',(89.9991163215577,-22.2556964040098,2.00056004657469));
#21263=CARTESIAN_POINT('Ctrl Pts',(90.7120875494009,-21.8321134766477,1.94789899149181));
#21264=CARTESIAN_POINT('Ctrl Pts',(91.4250587772441,-21.4085305492857,1.89523793640893));
#21265=CARTESIAN_POINT('Ctrl Pts',(92.3674116794532,-21.3709721384377,1.84257688132605));
#21266=CARTESIAN_POINT('Ctrl Pts',(93.1117465266451,-21.7366426720986,1.78991582624317));
#21267=CARTESIAN_POINT('Ctrl Pts',(93.8560813738369,-22.1023132057595,1.7372547711603));
#21268=CARTESIAN_POINT('Ctrl Pts',(94.4023981660114,-22.8712126839293,1.68459371607742));
#21269=CARTESIAN_POINT('Ctrl Pts',(94.502987230808,-23.6942827713943,1.63193266099454));
#21270=CARTESIAN_POINT('Ctrl Pts',(94.6035762956047,-24.5173528588592,1.57927160591166));
#21271=CARTESIAN_POINT('Ctrl Pts',(94.2584376330234,-25.3945935556193,1.52661055082878));
#21272=CARTESIAN_POINT('Ctrl Pts',(93.6239875152206,-25.9288761516102,1.4739494957459));
#21273=CARTESIAN_POINT('Ctrl Pts',(92.9895373974178,-26.4631587476011,1.42128844066303));
#21274=CARTESIAN_POINT('Ctrl Pts',(92.0657758243935,-26.6544832428228,1.36862738558015));
#21275=CARTESIAN_POINT('Ctrl Pts',(91.2718709044644,-26.4146102691233,1.31596633049727));
#21276=CARTESIAN_POINT('Ctrl Pts',(90.4779659845352,-26.1747372954238,1.26330527541439));
#21277=CARTESIAN_POINT('Ctrl Pts',(89.8139177177011,-25.503666852803,1.21064422033151));
#21278=CARTESIAN_POINT('Ctrl Pts',(89.5807312014043,-24.7092672371348,1.15798316524864));
#21279=CARTESIAN_POINT('Ctrl Pts',(89.5137200371456,-24.480979409957,1.14284987766308));
#21280=CARTESIAN_POINT('Ctrl Pts',(89.4822904668902,-24.2425067646591,1.12771659007753));
#21281=CARTESIAN_POINT('Ctrl Pts',(89.4843725317804,-24.0035302714347,1.11258330249198));
#21282=CARTESIAN_POINT('Ctrl Pts',(89.486504426694,-23.9997257424662,1.38741669750802));
#21283=CARTESIAN_POINT('Ctrl Pts',(89.4868032667881,-24.4310635958632,1.41458082386326));
#21284=CARTESIAN_POINT('Ctrl Pts',(89.5921778743622,-24.8625676650245,1.4417449502185));
#21285=CARTESIAN_POINT('Ctrl Pts',(89.8017475042685,-25.2354979719165,1.46890907657374));
#21286=CARTESIAN_POINT('Ctrl Pts',(90.2080244328865,-25.958469996729,1.52157013165662));
#21287=CARTESIAN_POINT('Ctrl Pts',(91.0058940734353,-26.4613061848995,1.57423118673949));
#21288=CARTESIAN_POINT('Ctrl Pts',(91.8333901892196,-26.5160872321709,1.62689224182237));
#21289=CARTESIAN_POINT('Ctrl Pts',(92.6608863050038,-26.5708682794422,1.67955329690525));
#21290=CARTESIAN_POINT('Ctrl Pts',(93.5180088960235,-26.1775941858145,1.73221435198813));
#21291=CARTESIAN_POINT('Ctrl Pts',(94.0160963730402,-25.5145600286215,1.78487540707101));
#21292=CARTESIAN_POINT('Ctrl Pts',(94.5141838500569,-24.8515258714286,1.83753646215389));
#21293=CARTESIAN_POINT('Ctrl Pts',(94.6532362130706,-23.9187316506705,1.89019751723677));
#21294=CARTESIAN_POINT('Ctrl Pts',(94.3701623803631,-23.1392455433219,1.94285857231964));
#21295=CARTESIAN_POINT('Ctrl Pts',(94.0870885476557,-22.3597594359734,1.99551962740252));
#21296=CARTESIAN_POINT('Ctrl Pts',(93.3818885192271,-21.7335814420345,2.0481806824854));
#21297=CARTESIAN_POINT('Ctrl Pts',(92.5743964779127,-21.5446792416752,2.10084173756828));
#21298=CARTESIAN_POINT('Ctrl Pts',(91.7669044365982,-21.3557770413159,2.15350279265115));
#21299=CARTESIAN_POINT('Ctrl Pts',(90.8571203823979,-21.6041506345363,2.20616384773403));
#21300=CARTESIAN_POINT('Ctrl Pts',(90.2576400878061,-22.1771655681069,2.25882490281691));
#21301=CARTESIAN_POINT('Ctrl Pts',(89.7696877997114,-22.6435761415163,2.30168883438061));
#21302=CARTESIAN_POINT('Ctrl Pts',(89.4873207515092,-23.3250710178654,2.34455276594432));
#21303=CARTESIAN_POINT('Ctrl Pts',(89.4812642899865,-24.0021096151709,2.38741669750802));
#21304=CARTESIAN_POINT('Origin',(92.,-24.,5.));
#21305=CARTESIAN_POINT('',(89.4802713394158,-23.9981710493934,3.38741669750802));
#21306=CARTESIAN_POINT('',(89.4854090148867,-23.9984414282173,3.11258330249198));
#21307=CARTESIAN_POINT('',(89.4825,-24.,5.));
#21308=CARTESIAN_POINT('Ctrl Pts',(89.4854090148867,-23.9984414282173,3.11258330249198));
#21309=CARTESIAN_POINT('Ctrl Pts',(89.4836298808409,-23.6875464209234,3.0929825844054));
#21310=CARTESIAN_POINT('Ctrl Pts',(89.5370775357559,-23.3772414115068,3.07338186631883));
#21311=CARTESIAN_POINT('Ctrl Pts',(89.6485421342809,-23.0894033947305,3.05378114823225));
#21312=CARTESIAN_POINT('Ctrl Pts',(89.9480129667671,-22.3160718469038,3.00112009314937));
#21313=CARTESIAN_POINT('Ctrl Pts',(90.6662677151581,-21.704913874088,2.94845903806649));
#21314=CARTESIAN_POINT('Ctrl Pts',(91.4775657731397,-21.5330988908351,2.89579798298361));
#21315=CARTESIAN_POINT('Ctrl Pts',(92.2888638311213,-21.3612839075822,2.84313692790074));
#21316=CARTESIAN_POINT('Ctrl Pts',(93.1932051986935,-21.628811913892,2.79047587281786));
#21317=CARTESIAN_POINT('Ctrl Pts',(93.7804552648549,-22.2143567539363,2.73781481773498));
#21318=CARTESIAN_POINT('Ctrl Pts',(94.3677053310163,-22.7999015939806,2.6851537626521));
#21319=CARTESIAN_POINT('Ctrl Pts',(94.6378640957668,-23.7034632677594,2.63249270756922));
#21320=CARTESIAN_POINT('Ctrl Pts',(94.4684106985952,-24.5152563159491,2.57983165248635));
#21321=CARTESIAN_POINT('Ctrl Pts',(94.2989573014235,-25.3270493641389,2.52717059740347));
#21322=CARTESIAN_POINT('Ctrl Pts',(93.6898917423296,-26.0470737867397,2.47450954232059));
#21323=CARTESIAN_POINT('Ctrl Pts',(92.9174341156813,-26.3487960615596,2.42184848723771));
#21324=CARTESIAN_POINT('Ctrl Pts',(92.1449764890331,-26.6505183363795,2.36918743215483));
#21325=CARTESIAN_POINT('Ctrl Pts',(91.2091267948306,-26.5339384634185,2.31652637707196));
#21326=CARTESIAN_POINT('Ctrl Pts',(90.5343119667252,-26.0519073104888,2.26386532198908));
#21327=CARTESIAN_POINT('Ctrl Pts',(89.8881206474051,-25.5903223931277,2.21343798215671));
#21328=CARTESIAN_POINT('Ctrl Pts',(89.4812892995851,-24.7936312531159,2.16301064232435));
#21329=CARTESIAN_POINT('Ctrl Pts',(89.478587803344,-23.999354427872,2.11258330249198));
#21330=CARTESIAN_POINT('Ctrl Pts',(89.4812642899865,-24.0021096151709,2.38741669750802));
#21331=CARTESIAN_POINT('Ctrl Pts',(89.4798800048903,-24.1568558207352,2.3972138210272));
#21332=CARTESIAN_POINT('Ctrl Pts',(89.4929305169813,-24.3113692249256,2.40701094454637));
#21333=CARTESIAN_POINT('Ctrl Pts',(89.5212603168746,-24.4630284201485,2.41680806806555));
#21334=CARTESIAN_POINT('Ctrl Pts',(89.6735373755183,-25.2782200646988,2.46946912314842));
#21335=CARTESIAN_POINT('Ctrl Pts',(90.2672680277891,-26.0109470798785,2.5221301782313));
#21336=CARTESIAN_POINT('Ctrl Pts',(91.0331836548293,-26.3289069878288,2.57479123331418));
#21337=CARTESIAN_POINT('Ctrl Pts',(91.7990992818695,-26.6468668957791,2.62745228839706));
#21338=CARTESIAN_POINT('Ctrl Pts',(92.7371998836791,-26.5500596964999,2.68011334347994));
#21339=CARTESIAN_POINT('Ctrl Pts',(93.4220416283355,-26.0823882608119,2.73277439856281));
#21340=CARTESIAN_POINT('Ctrl Pts',(94.1068833729918,-25.6147168251239,2.78543545364569));
#21341=CARTESIAN_POINT('Ctrl Pts',(94.538466260495,-24.7761811530271,2.83809650872857));
#21342=CARTESIAN_POINT('Ctrl Pts',(94.5210596939212,-23.9470718966112,2.89075756381145));
#21343=CARTESIAN_POINT('Ctrl Pts',(94.5036531273474,-23.1179626401953,2.94341861889433));
#21344=CARTESIAN_POINT('Ctrl Pts',(94.0372571066967,-22.2982797994604,2.9960796739772));
#21345=CARTESIAN_POINT('Ctrl Pts',(93.3333903788127,-21.8597633286133,3.04874072906008));
#21346=CARTESIAN_POINT('Ctrl Pts',(92.6295236509286,-21.4212468577662,3.10140178414296));
#21347=CARTESIAN_POINT('Ctrl Pts',(91.6881862158112,-21.3638967568069,3.15406283922584));
#21348=CARTESIAN_POINT('Ctrl Pts',(90.9362905712497,-21.713722374568,3.20672389430872));
#21349=CARTESIAN_POINT('Ctrl Pts',(90.1843949266882,-22.063547992329,3.2593849493916));
#21350=CARTESIAN_POINT('Ctrl Pts',(89.6219410726826,-22.8205493288104,3.31204600447448));
#21351=CARTESIAN_POINT('Ctrl Pts',(89.5040114769093,-23.6414133102582,3.36470705955735));
#21352=CARTESIAN_POINT('Ctrl Pts',(89.4870594274965,-23.759410210726,3.37227693887424));
#21353=CARTESIAN_POINT('Ctrl Pts',(89.4792926975419,-23.8787267215066,3.37984681819113));
#21354=CARTESIAN_POINT('Ctrl Pts',(89.4802713394158,-23.9981710493934,3.38741669750802));
#21355=CARTESIAN_POINT('Origin',(92.,-24.,5.));
#21356=CARTESIAN_POINT('',(89.4864158728457,-23.9996457834086,4.38741669750802));
#21357=CARTESIAN_POINT('',(89.4839749917547,-24.0021063689016,4.11258330249198));
#21358=CARTESIAN_POINT('',(89.4825,-24.,5.));
#21359=CARTESIAN_POINT('Ctrl Pts',(89.4839749917547,-24.0021063689016,4.11258330249198));
#21360=CARTESIAN_POINT('Ctrl Pts',(89.4886916234371,-23.4165893004159,4.07561558156934));
#21361=CARTESIAN_POINT('Ctrl Pts',(89.6925944465198,-22.8281096510768,4.0386478606467));
#21362=CARTESIAN_POINT('Ctrl Pts',(90.066215027555,-22.381662646436,4.00168013972406));
#21363=CARTESIAN_POINT('Ctrl Pts',(90.598442968768,-21.7456924076384,3.94901908464118));
#21364=CARTESIAN_POINT('Ctrl Pts',(91.4750692458126,-21.3979407209711,3.8963580295583));
#21365=CARTESIAN_POINT('Ctrl Pts',(92.2985288839647,-21.4961188951354,3.84369697447542));
#21366=CARTESIAN_POINT('Ctrl Pts',(93.1219885221168,-21.5942970692997,3.79103591939254));
#21367=CARTESIAN_POINT('Ctrl Pts',(93.8922815213763,-22.1384051042956,3.73837486430966));
#21368=CARTESIAN_POINT('Ctrl Pts',(94.2600668556347,-22.8816807530475,3.68571380922679));
#21369=CARTESIAN_POINT('Ctrl Pts',(94.627852189893,-23.6249564017993,3.63305275414391));
#21370=CARTESIAN_POINT('Ctrl Pts',(94.5931298591502,-24.5673996643072,3.58039169906103));
#21371=CARTESIAN_POINT('Ctrl Pts',(94.1716470433212,-25.2815963706942,3.52773064397815));
#21372=CARTESIAN_POINT('Ctrl Pts',(93.7501642274922,-25.9957930770812,3.47506958889527));
#21373=CARTESIAN_POINT('Ctrl Pts',(92.941920926577,-26.4817432273472,3.4224085338124));
#21374=CARTESIAN_POINT('Ctrl Pts',(92.1134692499477,-26.5190602709168,3.36974747872952));
#21375=CARTESIAN_POINT('Ctrl Pts',(91.2850175733184,-26.5563773144864,3.31708642364664));
#21376=CARTESIAN_POINT('Ctrl Pts',(90.4363575209752,-26.1450612513594,3.26442536856376));
#21377=CARTESIAN_POINT('Ctrl Pts',(89.9523709530942,-25.4716506583771,3.21176431348088));
#21378=CARTESIAN_POINT('Ctrl Pts',(89.6485266983476,-25.0488869840482,3.17870397648458));
#21379=CARTESIAN_POINT('Ctrl Pts',(89.4884098626544,-24.5228249567292,3.14564363948828));
#21380=CARTESIAN_POINT('Ctrl Pts',(89.4854090148867,-23.9984414282173,3.11258330249198));
#21381=CARTESIAN_POINT('Ctrl Pts',(89.4802713394158,-23.9981710493934,3.38741669750802));
#21382=CARTESIAN_POINT('Ctrl Pts',(89.4861007735321,-24.7096599592594,3.43250787327401));
#21383=CARTESIAN_POINT('Ctrl Pts',(89.8022314305929,-25.4256840455739,3.47759904904));
#21384=CARTESIAN_POINT('Ctrl Pts',(90.3356791886478,-25.8943545894189,3.52269022480599));
#21385=CARTESIAN_POINT('Ctrl Pts',(90.958681833701,-26.4417052607172,3.57535127988886));
#21386=CARTESIAN_POINT('Ctrl Pts',(91.8780924613484,-26.6516799768993,3.62801233497174));
#21387=CARTESIAN_POINT('Ctrl Pts',(92.6769426722523,-26.4290516090785,3.68067339005462));
#21388=CARTESIAN_POINT('Ctrl Pts',(93.4757928831562,-26.2064232412577,3.7333344451375));
#21389=CARTESIAN_POINT('Ctrl Pts',(94.1540826773166,-25.551191789434,3.78599550022038));
#21390=CARTESIAN_POINT('Ctrl Pts',(94.4041960519401,-24.7605159049425,3.83865655530326));
#21391=CARTESIAN_POINT('Ctrl Pts',(94.6543094265635,-23.969840020451,3.89131761038614));
#21392=CARTESIAN_POINT('Ctrl Pts',(94.4762463816501,-23.0437197032917,3.94397866546901));
#21393=CARTESIAN_POINT('Ctrl Pts',(93.9507615495482,-22.4021663197385,3.99663972055189));
#21394=CARTESIAN_POINT('Ctrl Pts',(93.4252767174463,-21.7606129361853,4.04930077563477));
#21395=CARTESIAN_POINT('Ctrl Pts',(92.5523700981559,-21.4036264862383,4.10196183071765));
#21396=CARTESIAN_POINT('Ctrl Pts',(91.727919739318,-21.4931064186725,4.15462288580053));
#21397=CARTESIAN_POINT('Ctrl Pts',(90.9034693804802,-21.5825863511068,4.2072839408834));
#21398=CARTESIAN_POINT('Ctrl Pts',(90.1274752820949,-22.1185326659223,4.25994499596628));
#21399=CARTESIAN_POINT('Ctrl Pts',(89.7518640115846,-22.8578845621823,4.31260605104916));
#21400=CARTESIAN_POINT('Ctrl Pts',(89.5739987186599,-23.20799397563,4.33754293320212));
#21401=CARTESIAN_POINT('Ctrl Pts',(89.4859136397297,-23.6037142279007,4.36247981535507));
#21402=CARTESIAN_POINT('Ctrl Pts',(89.4864158728457,-23.9996457834086,4.38741669750802));
#21403=CARTESIAN_POINT('Origin',(92.,-24.,5.));
#21404=CARTESIAN_POINT('',(89.4815255054053,-24.0021560919774,5.38741669750802));
#21405=CARTESIAN_POINT('',(89.4785001229596,-23.9995222403937,5.11258330249198));
#21406=CARTESIAN_POINT('',(89.4825,-24.,5.));
#21407=CARTESIAN_POINT('Ctrl Pts',(89.4785001229596,-23.9995222403937,5.11258330249198));
#21408=CARTESIAN_POINT('Ctrl Pts',(89.4784308438678,-23.9731625418826,5.11090963381615));
#21409=CARTESIAN_POINT('Ctrl Pts',(89.4788088040536,-23.9468048777982,5.10923596514032));
#21410=CARTESIAN_POINT('Ctrl Pts',(89.4796401577289,-23.9204615220786,5.1075622964645));
#21411=CARTESIAN_POINT('Ctrl Pts',(89.5057982392643,-23.09158246934,5.05490124138162));
#21412=CARTESIAN_POINT('Ctrl Pts',(89.9808209826826,-22.2768688588901,5.00224018629874));
#21413=CARTESIAN_POINT('Ctrl Pts',(90.6892774670547,-21.8458072171371,4.94957913121586));
#21414=CARTESIAN_POINT('Ctrl Pts',(91.3977339514269,-21.4147455753842,4.89691807613299));
#21415=CARTESIAN_POINT('Ctrl Pts',(92.3396241767529,-21.3673359023281,4.84425702105011));
#21416=CARTESIAN_POINT('Ctrl Pts',(93.0877848515153,-21.7250792935763,4.79159596596723));
#21417=CARTESIAN_POINT('Ctrl Pts',(93.8359455262777,-22.0828226848245,4.73893491088435));
#21418=CARTESIAN_POINT('Ctrl Pts',(94.3903766504766,-22.8457191403771,4.68627385580147));
#21419=CARTESIAN_POINT('Ctrl Pts',(94.4996342472564,-23.667782098445,4.63361280071859));
#21420=CARTESIAN_POINT('Ctrl Pts',(94.6088918440362,-24.4898450565128,4.58095174563572));
#21421=CARTESIAN_POINT('Ctrl Pts',(94.272975913397,-25.371074517096,4.52829069055284));
#21422=CARTESIAN_POINT('Ctrl Pts',(93.6442300627918,-25.9118178797765,4.47562963546996));
#21423=CARTESIAN_POINT('Ctrl Pts',(93.0154842121866,-26.452561242457,4.42296858038708));
#21424=CARTESIAN_POINT('Ctrl Pts',(92.0939084416155,-26.6528185072348,4.3703075253042));
#21425=CARTESIAN_POINT('Ctrl Pts',(91.2974530904191,-26.4217695888032,4.31764647022132));
#21426=CARTESIAN_POINT('Ctrl Pts',(90.5009977392227,-26.1907206703715,4.26498541513845));
#21427=CARTESIAN_POINT('Ctrl Pts',(89.8296628074011,-25.5283655687303,4.21232436005557));
#21428=CARTESIAN_POINT('Ctrl Pts',(89.5879101441809,-24.7350936224458,4.15966330497269));
#21429=CARTESIAN_POINT('Ctrl Pts',(89.5158662908614,-24.4986934646177,4.14396997081245));
#21430=CARTESIAN_POINT('Ctrl Pts',(89.4819727131382,-24.2506668639209,4.12827663665222));
#21431=CARTESIAN_POINT('Ctrl Pts',(89.4839749917547,-24.0021063689016,4.11258330249198));
#21432=CARTESIAN_POINT('Ctrl Pts',(89.4864158728457,-23.9996457834086,4.38741669750802));
#21433=CARTESIAN_POINT('Ctrl Pts',(89.4869742424795,-24.439832124507,4.41514087043795));
#21434=CARTESIAN_POINT('Ctrl Pts',(89.5970301658382,-24.8802796450794,4.44286504336787));
#21435=CARTESIAN_POINT('Ctrl Pts',(89.8149443593501,-25.2586003903178,4.47058921629779));
#21436=CARTESIAN_POINT('Ctrl Pts',(90.2288644202614,-25.9772068444889,4.52325027138067));
#21437=CARTESIAN_POINT('Ctrl Pts',(91.0319329847194,-26.4716622751265,4.57591132646355));
#21438=CARTESIAN_POINT('Ctrl Pts',(91.8599447536684,-26.517722705864,4.62857238154643));
#21439=CARTESIAN_POINT('Ctrl Pts',(92.6879565226175,-26.5637831366015,4.68123343662931));
#21440=CARTESIAN_POINT('Ctrl Pts',(93.5409114960576,-26.1614485674388,4.73389449171218));
#21441=CARTESIAN_POINT('Ctrl Pts',(94.0319800368686,-25.4931845918408,4.78655554679506));
#21442=CARTESIAN_POINT('Ctrl Pts',(94.5230485776795,-24.8249206162428,4.83921660187794));
#21443=CARTESIAN_POINT('Ctrl Pts',(94.6522306858613,-23.8907272342096,4.89187765696082));
#21444=CARTESIAN_POINT('Ctrl Pts',(94.3609400707585,-23.1142770874653,4.9445387120437));
#21445=CARTESIAN_POINT('Ctrl Pts',(94.0696494556558,-22.337826940721,4.99719976712657));
#21446=CARTESIAN_POINT('Ctrl Pts',(93.3578861172687,-21.7191200292656,5.04986082220945));
#21447=CARTESIAN_POINT('Ctrl Pts',(92.5484468765423,-21.5387504963612,5.10252187729233));
#21448=CARTESIAN_POINT('Ctrl Pts',(91.739007635816,-21.3583809634567,5.15518293237521));
#21449=CARTESIAN_POINT('Ctrl Pts',(90.8318924927504,-21.6163488091031,5.20784398745809));
#21450=CARTESIAN_POINT('Ctrl Pts',(90.2384936456262,-22.1956612127896,5.26050504254097));
#21451=CARTESIAN_POINT('Ctrl Pts',(89.7618021600142,-22.6610367214972,5.30280892752999));
#21452=CARTESIAN_POINT('Ctrl Pts',(89.48756099645,-23.3337852933997,5.345112812519));
#21453=CARTESIAN_POINT('Ctrl Pts',(89.4815255054053,-24.0021560919774,5.38741669750802));
#21454=CARTESIAN_POINT('Origin',(92.,-24.,5.));
#21455=CARTESIAN_POINT('',(89.4800391863944,-23.9982645761521,6.38741669750803));
#21456=CARTESIAN_POINT('',(89.4852341727342,-23.9983410426721,6.11258330249198));
#21457=CARTESIAN_POINT('',(89.4825,-24.,5.));
#21458=CARTESIAN_POINT('Ctrl Pts',(89.4852341727342,-23.9983410426721,6.11258330249198));
#21459=CARTESIAN_POINT('Ctrl Pts',(89.483386156444,-23.6963819807171,6.09354263098009));
#21460=CARTESIAN_POINT('Ctrl Pts',(89.533738485222,-23.3950185131867,6.07450195946819));
#21461=CARTESIAN_POINT('Ctrl Pts',(89.6390604846241,-23.114277295821,6.0554612879563));
#21462=CARTESIAN_POINT('Ctrl Pts',(89.9303510312042,-22.3378273317272,6.00280023287342));
#21463=CARTESIAN_POINT('Ctrl Pts',(90.6421142021576,-21.719120565815,5.95013917779055));
#21464=CARTESIAN_POINT('Ctrl Pts',(91.4515532524732,-21.5387510753403,5.89747812270767));
#21465=CARTESIAN_POINT('Ctrl Pts',(92.2609923027888,-21.3583815848656,5.84481706762479));
#21466=CARTESIAN_POINT('Ctrl Pts',(93.1681072324665,-21.6163493698282,5.79215601254191));
#21467=CARTESIAN_POINT('Ctrl Pts',(93.7615059400007,-22.1956616372385,5.73949495745904));
#21468=CARTESIAN_POINT('Ctrl Pts',(94.354904647535,-22.7749739046489,5.68683390237616));
#21469=CARTESIAN_POINT('Ctrl Pts',(94.6345871329257,-23.675630654507,5.63417284729328));
#21470=CARTESIAN_POINT('Ctrl Pts',(94.4737126159701,-24.4891686800901,5.5815117922104));
#21471=CARTESIAN_POINT('Ctrl Pts',(94.3128380990145,-25.3027067056733,5.52885073712752));
#21472=CARTESIAN_POINT('Ctrl Pts',(93.7114065797127,-26.0291260069815,5.47618968204464));
#21473=CARTESIAN_POINT('Ctrl Pts',(92.9421775161413,-26.3389830337326,5.42352862696177));
#21474=CARTESIAN_POINT('Ctrl Pts',(92.17294845257,-26.6488400604838,5.37086757187889));
#21475=CARTESIAN_POINT('Ctrl Pts',(91.2359218447291,-26.5421348126778,5.31820651679601));
#21476=CARTESIAN_POINT('Ctrl Pts',(90.556055250635,-26.0672599412612,5.26554546171313));
#21477=CARTESIAN_POINT('Ctrl Pts',(89.8977961123825,-25.6074774981291,5.21455807530608));
#21478=CARTESIAN_POINT('Ctrl Pts',(89.4806106720036,-24.8025558114754,5.16357068889903));
#21479=CARTESIAN_POINT('Ctrl Pts',(89.4785001229596,-23.9995222403937,5.11258330249198));
#21480=CARTESIAN_POINT('Ctrl Pts',(89.4815255054053,-24.0021560919774,5.38741669750802));
#21481=CARTESIAN_POINT('Ctrl Pts',(89.4800478489828,-24.1657918915839,5.39777386760188));
#21482=CARTESIAN_POINT('Ctrl Pts',(89.494646624663,-24.3291652844524,5.40813103769574));
#21483=CARTESIAN_POINT('Ctrl Pts',(89.5262868021188,-24.4891687951612,5.4184882077896));
#21484=CARTESIAN_POINT('Ctrl Pts',(89.6871613569182,-25.3027070121193,5.47114926287248));
#21485=CARTESIAN_POINT('Ctrl Pts',(90.2885930176996,-26.0291264843089,5.52381031795536));
#21486=CARTESIAN_POINT('Ctrl Pts',(91.0578222622228,-26.3389835839502,5.57647137303824));
#21487=CARTESIAN_POINT('Ctrl Pts',(91.827051506746,-26.6488406835915,5.62913242812111));
#21488=CARTESIAN_POINT('Ctrl Pts',(92.764078335011,-26.5421354106845,5.68179348320399));
#21489=CARTESIAN_POINT('Ctrl Pts',(93.4439450890356,-26.0672604275592,5.73445453828687));
#21490=CARTESIAN_POINT('Ctrl Pts',(94.1238118430601,-25.5923854444339,5.78711559336975));
#21491=CARTESIAN_POINT('Ctrl Pts',(94.5465185228442,-24.7493407510902,5.83977664845263));
#21492=CARTESIAN_POINT('Ctrl Pts',(94.5203604351554,-23.920461503368,5.89243770353551));
#21493=CARTESIAN_POINT('Ctrl Pts',(94.4942023474666,-23.0915822556457,5.94509875861838));
#21494=CARTESIAN_POINT('Ctrl Pts',(94.019179492305,-22.2768684535448,5.99775981370126));
#21495=CARTESIAN_POINT('Ctrl Pts',(93.310722841277,-21.8458067103895,6.05042086878414));
#21496=CARTESIAN_POINT('Ctrl Pts',(92.602266190249,-21.4147449672342,6.10308192386702));
#21497=CARTESIAN_POINT('Ctrl Pts',(91.6603757433546,-21.3673352830245,6.15574297894989));
#21498=CARTESIAN_POINT('Ctrl Pts',(90.9122148925964,-21.725078758428,6.20840403403277));
#21499=CARTESIAN_POINT('Ctrl Pts',(90.1640540418382,-22.0828222338316,6.26106508911565));
#21500=CARTESIAN_POINT('Ctrl Pts',(89.6096227872161,-22.8457188688485,6.31372614419853));
#21501=CARTESIAN_POINT('Ctrl Pts',(89.5003651647348,-23.6677820202958,6.36638719928141));
#21502=CARTESIAN_POINT('Ctrl Pts',(89.4858216342605,-23.7772087149586,6.37339703202361));
#21503=CARTESIAN_POINT('Ctrl Pts',(89.4791660807206,-23.8876837738622,6.38040686476582));
#21504=CARTESIAN_POINT('Ctrl Pts',(89.4800391863944,-23.9982645761521,6.38741669750803));
#21505=CARTESIAN_POINT('Origin',(92.,-24.,5.));
#21506=CARTESIAN_POINT('',(89.4863708146039,-23.9995053986078,7.38741669750802));
#21507=CARTESIAN_POINT('',(89.4842078764603,-24.0020516719095,7.11258330249199));
#21508=CARTESIAN_POINT('',(89.4825,-24.,5.));
#21509=CARTESIAN_POINT('Ctrl Pts',(89.4842078764603,-24.0020516719095,7.11258330249199));
#21510=CARTESIAN_POINT('Ctrl Pts',(89.4887016384805,-23.4252697537026,7.07617562814403));
#21511=CARTESIAN_POINT('Ctrl Pts',(89.6859405266727,-22.8457100529155,7.03976795379607));
#21512=CARTESIAN_POINT('Ctrl Pts',(90.0492389093472,-22.4021666956129,7.00336027944811));
#21513=CARTESIAN_POINT('Ctrl Pts',(90.5747236178373,-21.7606134629807,6.95069922436523));
#21514=CARTESIAN_POINT('Ctrl Pts',(91.4476300317824,-21.4036270970037,6.89803816928236));
#21515=CARTESIAN_POINT('Ctrl Pts',(92.2720801966773,-21.4931070083872,6.84537711419948));
#21516=CARTESIAN_POINT('Ctrl Pts',(93.096530361572,-21.5825869197707,6.7927160591166));
#21517=CARTESIAN_POINT('Ctrl Pts',(93.8725242774164,-22.1185331085148,6.74005500403372));
#21518=CARTESIAN_POINT('Ctrl Pts',(94.2481354595693,-22.8578848308521,6.68739394895084));
#21519=CARTESIAN_POINT('Ctrl Pts',(94.6237466417222,-23.5972365531893,6.63473289386796));
#21520=CARTESIAN_POINT('Ctrl Pts',(94.5989750901836,-24.5399938091198,6.58207183878509));
#21521=CARTESIAN_POINT('Ctrl Pts',(94.1850551266417,-25.2586000942469,6.52941078370221));
#21522=CARTESIAN_POINT('Ctrl Pts',(93.7711351630998,-25.977206379374,6.47674972861933));
#21523=CARTESIAN_POINT('Ctrl Pts',(92.9680667875545,-26.4716616936979,6.42408867353645));
#21524=CARTESIAN_POINT('Ctrl Pts',(92.1400552133854,-26.5177221136004,6.37142761845357));
#21525=CARTESIAN_POINT('Ctrl Pts',(91.3120436392162,-26.5637825335029,6.31876656337069));
#21526=CARTESIAN_POINT('Ctrl Pts',(90.4590888664232,-26.1614480589841,6.26610550828782));
#21527=CARTESIAN_POINT('Ctrl Pts',(89.9680204411301,-25.4931842405871,6.21344445320494));
#21528=CARTESIAN_POINT('Ctrl Pts',(89.6545077552948,-25.0665447464531,6.17982406963395));
#21529=CARTESIAN_POINT('Ctrl Pts',(89.4884972412917,-24.5315144383331,6.14620368606297));
#21530=CARTESIAN_POINT('Ctrl Pts',(89.4852341727342,-23.9983410426721,6.11258330249198));
#21531=CARTESIAN_POINT('Ctrl Pts',(89.4800391863944,-23.9982645761521,6.38741669750803));
#21532=CARTESIAN_POINT('Ctrl Pts',(89.4857252480609,-24.7184171072605,6.4330679198487));
#21533=CARTESIAN_POINT('Ctrl Pts',(89.8107173609326,-25.4430544346852,6.47871914218937));
#21534=CARTESIAN_POINT('Ctrl Pts',(90.3557695504229,-25.9118183295065,6.52437036453004));
#21535=CARTESIAN_POINT('Ctrl Pts',(90.9845155489329,-26.4525618193923,6.57703141961292));
#21536=CARTESIAN_POINT('Ctrl Pts',(91.9060915362935,-26.6528191312864,6.6296924746958));
#21537=CARTESIAN_POINT('Ctrl Pts',(92.7025470748465,-26.4217701584994,6.68235352977868));
#21538=CARTESIAN_POINT('Ctrl Pts',(93.4990026133995,-26.1907211857124,6.73501458486155));
#21539=CARTESIAN_POINT('Ctrl Pts',(94.170337703145,-25.5283659282443,6.78767563994443));
#21540=CARTESIAN_POINT('Ctrl Pts',(94.4120904232343,-24.7350937953597,6.84033669502731));
#21541=CARTESIAN_POINT('Ctrl Pts',(94.6538431433237,-23.941821662475,6.89299775011019));
#21542=CARTESIAN_POINT('Ctrl Pts',(94.4660134937569,-23.0176326541737,6.94565880519307));
#21543=CARTESIAN_POINT('Ctrl Pts',(93.9337854273444,-22.3816622657573,6.99831986027595));
#21544=CARTESIAN_POINT('Ctrl Pts',(93.4015573609318,-21.7456918773409,7.05098091535883));
#21545=CARTESIAN_POINT('Ctrl Pts',(92.5249308776734,-21.3979401088093,7.1036419704417));
#21546=CARTESIAN_POINT('Ctrl Pts',(91.7014710458108,-21.4961183060969,7.15630302552458));
#21547=CARTESIAN_POINT('Ctrl Pts',(90.8780112139482,-21.5942965033845,7.20896408060746));
#21548=CARTESIAN_POINT('Ctrl Pts',(90.1077180334812,-22.1384046664913,7.26162513569034));
#21549=CARTESIAN_POINT('Ctrl Pts',(89.7399326127096,-22.8816804900357,7.31428619077321));
#21550=CARTESIAN_POINT('Ctrl Pts',(89.569684509702,-23.2257433370738,7.33866302635148));
#21551=CARTESIAN_POINT('Ctrl Pts',(89.4856845592314,-23.6124832315577,7.36303986192975));
#21552=CARTESIAN_POINT('Ctrl Pts',(89.4863708146039,-23.9995053986078,7.38741669750802));
#21553=CARTESIAN_POINT('Origin',(92.,-24.,5.));
#21554=CARTESIAN_POINT('',(89.4817891743669,-24.002194435609,8.38741669750802));
#21555=CARTESIAN_POINT('',(89.4784371162896,-23.999680408535,8.11258330249198));
#21556=CARTESIAN_POINT('',(89.4825,-24.,5.));
#21557=CARTESIAN_POINT('Ctrl Pts',(89.4784371162896,-23.999680408535,8.11258330249198));
#21558=CARTESIAN_POINT('Ctrl Pts',(89.4784054922001,-23.9821424240367,8.11146968039084));
#21559=CARTESIAN_POINT('Ctrl Pts',(89.4785728027447,-23.9646050586431,8.11035605828969));
#21560=CARTESIAN_POINT('Ctrl Pts',(89.4789408989109,-23.9470719086913,8.10924243618855));
#21561=CARTESIAN_POINT('Ctrl Pts',(89.4963474612121,-23.1179628469758,8.05658138110567));
#21562=CARTESIAN_POINT('Ctrl Pts',(89.9627433725619,-22.298280199785,8.0039203260228));
#21563=CARTESIAN_POINT('Ctrl Pts',(90.6666099349663,-21.8597638322688,7.95125927093992));
#21564=CARTESIAN_POINT('Ctrl Pts',(91.3704764973707,-21.4212474647526,7.89859821585704));
#21565=CARTESIAN_POINT('Ctrl Pts',(92.3118137108296,-21.3638973769109,7.84593716077416));
#21566=CARTESIAN_POINT('Ctrl Pts',(93.0637091784649,-21.7137229122891,7.79327610569128));
#21567=CARTESIAN_POINT('Ctrl Pts',(93.8156046461002,-22.0635484476673,7.7406150506084));
#21568=CARTESIAN_POINT('Ctrl Pts',(94.378058367912,-22.8205496062654,7.68795399552553));
#21569=CARTESIAN_POINT('Ctrl Pts',(94.4959879359714,-23.6414133946617,7.63529294044265));
#21570=CARTESIAN_POINT('Ctrl Pts',(94.6139175040309,-24.462277183058,7.58263188535977));
#21571=CARTESIAN_POINT('Ctrl Pts',(94.287322918338,-25.3470036012526,7.52997083027689));
#21572=CARTESIAN_POINT('Ctrl Pts',(93.6643204198241,-25.8943541437692,7.47730977519401));
#21573=CARTESIAN_POINT('Ctrl Pts',(93.0413179213102,-26.4417046862858,7.42464872011113));
#21574=CARTESIAN_POINT('Ctrl Pts',(92.1219075099752,-26.6516793531245,7.37198766502826));
#21575=CARTESIAN_POINT('Ctrl Pts',(91.3230574869989,-26.4290510376866,7.31932660994538));
#21576=CARTESIAN_POINT('Ctrl Pts',(90.5242074640225,-26.2064227222488,7.2666655548625));
#21577=CARTESIAN_POINT('Ctrl Pts',(89.8459178294048,-25.5511914245345,7.21400449977963));
#21578=CARTESIAN_POINT('Ctrl Pts',(89.5958045136134,-24.7605157260336,7.16134344469675));
#21579=CARTESIAN_POINT('Ctrl Pts',(89.5186091945673,-24.5164804869872,7.14509006396183));
#21580=CARTESIAN_POINT('Ctrl Pts',(89.4822017382943,-24.2595428818132,7.12883668322691));
#21581=CARTESIAN_POINT('Ctrl Pts',(89.4842078764603,-24.0020516719095,7.11258330249199));
#21582=CARTESIAN_POINT('Ctrl Pts',(89.4863708146039,-23.9995053986078,7.38741669750802));
#21583=CARTESIAN_POINT('Ctrl Pts',(89.4871670704398,-24.4485636814537,7.41570091701263));
#21584=CARTESIAN_POINT('Ctrl Pts',(89.6019742377664,-24.8980019807642,7.44398513651724));
#21585=CARTESIAN_POINT('Ctrl Pts',(89.8283524458306,-25.2815966720592,7.47226935602185));
#21586=CARTESIAN_POINT('Ctrl Pts',(90.2498353607997,-25.9957935465564,7.52493041110473));
#21587=CARTESIAN_POINT('Ctrl Pts',(91.0580788518144,-26.4817438115688,7.57759146618761));
#21588=CARTESIAN_POINT('Ctrl Pts',(91.8865307233466,-26.5190608637177,7.63025252127048));
#21589=CARTESIAN_POINT('Ctrl Pts',(92.7149825948789,-26.5563779158667,7.68291357635336));
#21590=CARTESIAN_POINT('Ctrl Pts',(93.5636428469287,-26.1450617551521,7.73557463143624));
#21591=CARTESIAN_POINT('Ctrl Pts',(94.0476295286171,-25.4716510041371,7.78823568651912));
#21592=CARTESIAN_POINT('Ctrl Pts',(94.5316162103055,-24.798240253122,7.84089674160199));
#21593=CARTESIAN_POINT('Ctrl Pts',(94.6509293216325,-23.8627349118064,7.89355779668488));
#21594=CARTESIAN_POINT('Ctrl Pts',(94.3514584187992,-23.0894031813449,7.94621885176775));
#21595=CARTESIAN_POINT('Ctrl Pts',(94.0519875159659,-22.3160714508834,7.99887990685063));
#21596=CARTESIAN_POINT('Ctrl Pts',(93.3337325989723,-21.7049133312758,8.0515409619335));
#21597=CARTESIAN_POINT('Ctrl Pts',(92.5224343499209,-21.5330983089572,8.10420201701638));
#21598=CARTESIAN_POINT('Ctrl Pts',(91.7111361008695,-21.3612832866386,8.15686307209926));
#21599=CARTESIAN_POINT('Ctrl Pts',(90.8067945197604,-21.6288113616088,8.20952412718214));
#21600=CARTESIAN_POINT('Ctrl Pts',(90.2195443159446,-22.2143563368687,8.26218518226502));
#21601=CARTESIAN_POINT('Ctrl Pts',(89.7540375466956,-22.6785113902208,8.30392902067936));
#21602=CARTESIAN_POINT('Ctrl Pts',(89.4877769931074,-23.3424942170044,8.34567285909369));
#21603=CARTESIAN_POINT('Ctrl Pts',(89.4817891743669,-24.002194435609,8.38741669750802));
#21604=CARTESIAN_POINT('Origin',(92.,-24.,5.));
#21605=CARTESIAN_POINT('',(89.4798238762261,-23.9984131135314,9.38741669750802));
#21606=CARTESIAN_POINT('',(89.4850512338518,-23.9982506073194,9.11258330249198));
#21607=CARTESIAN_POINT('',(89.4825,-24.,5.));
#21608=CARTESIAN_POINT('',(93.9134659966651,-22.3640127966251,10.));
#21609=CARTESIAN_POINT('Ctrl Pts',(89.4798238762261,-23.9984131135314,9.38741669750802));
#21610=CARTESIAN_POINT('Ctrl Pts',(89.4853062059344,-24.7270927102602,9.43362796642338));
#21611=CARTESIAN_POINT('Ctrl Pts',(89.8192672097013,-25.4600319638108,9.47983923533874));
#21612=CARTESIAN_POINT('Ctrl Pts',(90.3760118920419,-25.9288769835329,9.5260505042541));
#21613=CARTESIAN_POINT('Ctrl Pts',(91.0104623858714,-26.46315950787,9.57871155933697));
#21614=CARTESIAN_POINT('Ctrl Pts',(91.9342250444885,-26.6544830013391,9.63137261441985));
#21615=CARTESIAN_POINT('Ctrl Pts',(92.7281293690809,-26.4146106072968,9.68403366950273));
#21616=CARTESIAN_POINT('Ctrl Pts',(93.5220336936733,-26.1747382132545,9.73669472458561));
#21617=CARTESIAN_POINT('Ctrl Pts',(94.186079684241,-25.5036699317008,9.78935577966849));
#21618=CARTESIAN_POINT('Ctrl Pts',(94.4192662809857,-24.7092700865749,9.84201683475137));
#21619=CARTESIAN_POINT('Ctrl Pts',(94.6524528777304,-23.914870241449,9.89467788983425));
#21620=CARTESIAN_POINT('Ctrl Pts',(94.4547800806522,-22.9971388327508,9.94733894491712));
#21621=CARTESIAN_POINT('Ctrl Pts',(93.9134659966651,-22.3640127966251,10.));
#21622=CARTESIAN_POINT('',(90.0828970444786,-22.361465706548,10.));
#21623=CARTESIAN_POINT('Origin',(92.,-24.,10.));
#21624=CARTESIAN_POINT('Ctrl Pts',(90.0828885913555,-22.3614597865289,10.));
#21625=CARTESIAN_POINT('Ctrl Pts',(90.6060434082611,-21.752303655963,9.94901908464118));
#21626=CARTESIAN_POINT('Ctrl Pts',(91.4465814718894,-21.4121729024441,9.89803816928235));
#21627=CARTESIAN_POINT('Ctrl Pts',(92.2457357606075,-21.4905154724921,9.84705725392353));
#21628=CARTESIAN_POINT('Ctrl Pts',(93.0712271767912,-21.5714399197601,9.79439619884065));
#21629=CARTESIAN_POINT('Ctrl Pts',(93.8525621626002,-22.0988748222944,9.74173514375777));
#21630=CARTESIAN_POINT('Ctrl Pts',(94.2358875787344,-22.8341463056132,9.68907408867489));
#21631=CARTESIAN_POINT('Ctrl Pts',(94.6192129948686,-23.5694177889319,9.63641303359201));
#21632=CARTESIAN_POINT('Ctrl Pts',(94.6045288413281,-24.5125258530351,9.58375197850914));
#21633=CARTESIAN_POINT('Ctrl Pts',(94.1982520122281,-25.235497804129,9.53109092342626));
#21634=CARTESIAN_POINT('Ctrl Pts',(93.7919751831282,-25.9584697552228,9.47842986834338));
#21635=CARTESIAN_POINT('Ctrl Pts',(92.9941056784689,-26.4613055933073,9.42576881326051));
#21636=CARTESIAN_POINT('Ctrl Pts',(92.1666097496597,-26.5160865743966,9.37310775817763));
#21637=CARTESIAN_POINT('Ctrl Pts',(91.3391138208505,-26.570867555486,9.32044670309475));
#21638=CARTESIAN_POINT('Ctrl Pts',(90.4819914678916,-26.1775936795802,9.26778564801187));
#21639=CARTESIAN_POINT('Ctrl Pts',(89.9839041146304,-25.5145597074388,9.21512459292899));
#21640=CARTESIAN_POINT('Ctrl Pts',(89.6606132128854,-25.0842077835489,9.18094416278332));
#21641=CARTESIAN_POINT('Ctrl Pts',(89.4885783498304,-24.5402099934131,9.14676373263765));
#21642=CARTESIAN_POINT('Ctrl Pts',(89.4850512338518,-23.9982506073194,9.11258330249198));
#21643=CARTESIAN_POINT('Origin',(92.,-24.,12.2084234471775));
#21644=CARTESIAN_POINT('',(88.9217237789782,-23.9992118506711,1.79157655282254));
#21645=CARTESIAN_POINT('',(88.9313888204345,-23.9996651715868,1.70842344717745));
#21646=CARTESIAN_POINT('',(88.9265,-23.9999999999999,12.2084234471775));
#21647=CARTESIAN_POINT('',(92.7937992825328,-26.9692229537457,0.999999999999999));
#21648=CARTESIAN_POINT('Ctrl Pts',(88.9313888204345,-23.9996651715868,1.70842344717745));
#21649=CARTESIAN_POINT('Ctrl Pts',(88.9310463723584,-23.5053847152746,1.68292651844982));
#21650=CARTESIAN_POINT('Ctrl Pts',(89.2764430280357,-21.9907712812588,1.6047685346393));
#21651=CARTESIAN_POINT('Ctrl Pts',(91.6460838609914,-20.3911589633379,1.4739494957459));
#21652=CARTESIAN_POINT('Ctrl Pts',(94.8312242725849,-21.7301456837402,1.31596633049727));
#21653=CARTESIAN_POINT('Ctrl Pts',(95.4433140827682,-25.1332953965992,1.15798316524863));
#21654=CARTESIAN_POINT('Ctrl Pts',(93.7762533017603,-26.7065713079336,1.05266105508288));
#21655=CARTESIAN_POINT('Ctrl Pts',(92.7937992825328,-26.9692229537457,0.999999999999999));
#21656=CARTESIAN_POINT('',(91.2062007174671,-26.9692229537457,1.));
#21657=CARTESIAN_POINT('Origin',(92.,-24.,0.999999999999999));
#21658=CARTESIAN_POINT('Ctrl Pts',(88.9217237789782,-23.9992118506711,1.79157655282254));
#21659=CARTESIAN_POINT('Ctrl Pts',(88.9215776858271,-23.9562584671078,1.78934283757203));
#21660=CARTESIAN_POINT('Ctrl Pts',(88.9417782923113,-22.9007977729438,1.73444806723864));
#21661=CARTESIAN_POINT('Ctrl Pts',(90.1476053652115,-20.8820474355396,1.62689224182238));
#21662=CARTESIAN_POINT('Ctrl Pts',(93.5990313571954,-20.7444874247256,1.46890907657374));
#21663=CARTESIAN_POINT('Ctrl Pts',(95.5999505159819,-23.5606294856849,1.31092591132511));
#21664=CARTESIAN_POINT('Ctrl Pts',(94.349302269142,-26.7394085052657,1.15462288580053));
#21665=CARTESIAN_POINT('Ctrl Pts',(92.1519061796922,-27.2254057458095,1.05098091535883));
#21666=CARTESIAN_POINT('Ctrl Pts',(91.2042985533737,-26.9743125149969,1.));
#21667=CARTESIAN_POINT('Origin',(92.,-24.,12.2084234471775));
#21668=CARTESIAN_POINT('',(88.930051482524,-23.9980972113707,2.79157655282254));
#21669=CARTESIAN_POINT('',(88.9249913784601,-24.0025755321659,2.70842344717745));
#21670=CARTESIAN_POINT('',(88.9265,-23.9999999999999,12.2084234471775));
#21671=CARTESIAN_POINT('Ctrl Pts',(88.9249913784601,-24.0025755321659,2.70842344717745));
#21672=CARTESIAN_POINT('Ctrl Pts',(88.9323854338683,-23.1760102376997,2.66555951561375));
#21673=CARTESIAN_POINT('Ctrl Pts',(89.7006357273797,-21.3218326978092,2.57003452896717));
#21674=CARTESIAN_POINT('Ctrl Pts',(92.8261378655289,-20.4685618660265,2.42184848723771));
#21675=CARTESIAN_POINT('Ctrl Pts',(95.4089767382702,-22.7619776329039,2.26386532198907));
#21676=CARTESIAN_POINT('Ctrl Pts',(94.899688828372,-26.1783943608088,2.10588215674044));
#21677=CARTESIAN_POINT('Ctrl Pts',(91.7604241409854,-27.6187851374898,1.9478989914918));
#21678=CARTESIAN_POINT('Ctrl Pts',(89.3097989934579,-26.0743436082074,1.81541275497081));
#21679=CARTESIAN_POINT('Ctrl Pts',(88.9317536605653,-24.5262657246815,1.73558757353269));
#21680=CARTESIAN_POINT('Ctrl Pts',(88.9313888204345,-23.9996651715868,1.70842344717745));
#21681=CARTESIAN_POINT('Ctrl Pts',(88.930051482524,-23.9980972113707,2.79157655282254));
#21682=CARTESIAN_POINT('Ctrl Pts',(88.9278794195688,-23.6185397913437,2.77197583473597));
#21683=CARTESIAN_POINT('Ctrl Pts',(89.1684425268395,-22.2218847391138,2.69971406156651));
#21684=CARTESIAN_POINT('Ctrl Pts',(91.2485917742672,-20.451900203599,2.57479123331418));
#21685=CARTESIAN_POINT('Ctrl Pts',(94.5607981614372,-21.4317381309793,2.41680806806555));
#21686=CARTESIAN_POINT('Ctrl Pts',(95.5502714048858,-24.7410888412383,2.25882490281692));
#21687=CARTESIAN_POINT('Ctrl Pts',(93.3195309927209,-27.3782229777192,2.10084173756828));
#21688=CARTESIAN_POINT('Ctrl Pts',(89.9403861581344,-26.9572790184773,1.94509228757016));
#21689=CARTESIAN_POINT('Ctrl Pts',(88.9250219115292,-24.96890790723,1.84200389265491));
#21690=CARTESIAN_POINT('Ctrl Pts',(88.9217237789782,-23.9992118506711,1.79157655282254));
#21691=CARTESIAN_POINT('Origin',(92.,-24.,12.2084234471775));
#21692=CARTESIAN_POINT('',(88.9283007496159,-24.0025715689449,3.79157655282255));
#21693=CARTESIAN_POINT('',(88.9237791307625,-23.9977671182961,3.70842344717745));
#21694=CARTESIAN_POINT('',(88.9265,-23.9999999999999,12.2084234471775));
#21695=CARTESIAN_POINT('Ctrl Pts',(88.9237791307624,-23.9977671182961,3.70842344717745));
#21696=CARTESIAN_POINT('Ctrl Pts',(88.9225843518948,-23.8519430302087,3.70085356786056));
#21697=CARTESIAN_POINT('Ctrl Pts',(88.9980297211289,-22.6929123616698,3.6406226334608));
#21698=CARTESIAN_POINT('Ctrl Pts',(90.4700852939275,-20.7116866521342,3.52773064397815));
#21699=CARTESIAN_POINT('Ctrl Pts',(93.9177920746623,-20.9217349563625,3.36974747872952));
#21700=CARTESIAN_POINT('Ctrl Pts',(95.625996447417,-23.9238742346134,3.21176431348088));
#21701=CARTESIAN_POINT('Ctrl Pts',(94.0452973355112,-26.9950631778383,3.05378114823225));
#21702=CARTESIAN_POINT('Ctrl Pts',(90.6094456576621,-27.3496255535896,2.89579798298361));
#21703=CARTESIAN_POINT('Ctrl Pts',(89.0248752439865,-25.3940964847871,2.78067874929868));
#21704=CARTESIAN_POINT('Ctrl Pts',(88.923301368433,-24.1914980595946,2.71822057069663));
#21705=CARTESIAN_POINT('Ctrl Pts',(88.9249913784601,-24.0025755321659,2.70842344717745));
#21706=CARTESIAN_POINT('Ctrl Pts',(88.9283007496159,-24.0025715689449,3.79157655282255));
#21707=CARTESIAN_POINT('Ctrl Pts',(88.934059068375,-23.287740701024,3.75460883189991));
#21708=CARTESIAN_POINT('Ctrl Pts',(89.5376069996118,-21.5458537101333,3.66498005589439));
#21709=CARTESIAN_POINT('Ctrl Pts',(92.429368893546,-20.3987114188412,3.52269022480599));
#21710=CARTESIAN_POINT('Ctrl Pts',(95.2506148119859,-22.3915408673733,3.36470705955735));
#21711=CARTESIAN_POINT('Ctrl Pts',(95.1234421205799,-25.8432978095596,3.20672389430872));
#21712=CARTESIAN_POINT('Ctrl Pts',(92.1632008669202,-27.6231203956681,3.04874072906009));
#21713=CARTESIAN_POINT('Ctrl Pts',(89.4405688436026,-26.3035551797938,2.91035828189803));
#21714=CARTESIAN_POINT('Ctrl Pts',(88.9337150795902,-24.6382929511448,2.82463688981885));
#21715=CARTESIAN_POINT('Ctrl Pts',(88.930051482524,-23.9980972113707,2.79157655282254));
#21716=CARTESIAN_POINT('Origin',(92.,-24.,12.2084234471775));
#21717=CARTESIAN_POINT('',(88.9216167340283,-23.9994167252631,4.79157655282255));
#21718=CARTESIAN_POINT('',(88.9312807091126,-23.9995675532497,4.70842344717745));
#21719=CARTESIAN_POINT('',(88.9265,-23.9999999999999,12.2084234471775));
#21720=CARTESIAN_POINT('Ctrl Pts',(88.9312807091126,-23.9995675532497,4.70842344717745));
#21721=CARTESIAN_POINT('Ctrl Pts',(88.9306675557931,-23.5161929213318,4.6834865650245));
#21722=CARTESIAN_POINT('Ctrl Pts',(89.2653046726707,-22.0128431381641,4.60588862778867));
#21723=CARTESIAN_POINT('Ctrl Pts',(91.6086716990242,-20.394378610344,4.47562963546995));
#21724=CARTESIAN_POINT('Ctrl Pts',(94.8057463695968,-21.7018636398323,4.31764647022133));
#21725=CARTESIAN_POINT('Ctrl Pts',(95.4579133231718,-25.0938367815869,4.15966330497269));
#21726=CARTESIAN_POINT('Ctrl Pts',(92.9736348536358,-27.493662641186,4.00168013972405));
#21727=CARTESIAN_POINT('Ctrl Pts',(89.7675877362369,-26.761466587215,3.85126685379231));
#21728=CARTESIAN_POINT('Ctrl Pts',(88.9308960188484,-24.8663912154056,3.75351462294344));
#21729=CARTESIAN_POINT('Ctrl Pts',(88.9237791307624,-23.9977671182961,3.70842344717745));
#21730=CARTESIAN_POINT('Ctrl Pts',(88.9216167340283,-23.9994167252631,4.79157655282255));
#21731=CARTESIAN_POINT('Ctrl Pts',(88.9215321543705,-23.9672353813211,4.78990288414672));
#21732=CARTESIAN_POINT('Ctrl Pts',(88.9365123597457,-22.9225665616792,4.73556816038801));
#21733=CARTESIAN_POINT('Ctrl Pts',(90.1148106026499,-20.9016620282348,4.62857238154643));
#21734=CARTESIAN_POINT('Ctrl Pts',(93.5645420118329,-20.7280211581598,4.4705892162978));
#21735=CARTESIAN_POINT('Ctrl Pts',(95.595180415279,-23.5221767762025,4.31260605104916));
#21736=CARTESIAN_POINT('Ctrl Pts',(94.3648674705089,-26.7497343695717,4.15462288580053));
#21737=CARTESIAN_POINT('Ctrl Pts',(90.9895390126931,-27.4831890308961,3.99663972055189));
#21738=CARTESIAN_POINT('Ctrl Pts',(89.1060884403934,-25.6249316453216,3.8756242762259));
#21739=CARTESIAN_POINT('Ctrl Pts',(88.9258562597141,-24.3060276489616,3.80726988698278));
#21740=CARTESIAN_POINT('Ctrl Pts',(88.9283007496159,-24.0025715689449,3.79157655282255));
#21741=CARTESIAN_POINT('Origin',(92.,-24.,12.2084234471775));
#21742=CARTESIAN_POINT('',(88.929838025779,-23.9979746552741,5.79157655282255));
#21743=CARTESIAN_POINT('',(88.9253102843548,-24.0026322735621,5.70842344717746));
#21744=CARTESIAN_POINT('',(88.9265,-23.9999999999999,12.2084234471775));
#21745=CARTESIAN_POINT('Ctrl Pts',(88.9253102843548,-24.0026322735621,5.70842344717746));
#21746=CARTESIAN_POINT('Ctrl Pts',(88.9326787378706,-23.1866490960334,5.66611956218844));
#21747=CARTESIAN_POINT('Ctrl Pts',(89.6842660273292,-21.3429095601006,5.57115462211654));
#21748=CARTESIAN_POINT('Ctrl Pts',(92.7888215932045,-20.4600276931837,5.42352862696176));
#21749=CARTESIAN_POINT('Ctrl Pts',(95.3956989960243,-22.7260801567682,5.26554546171313));
#21750=CARTESIAN_POINT('Ctrl Pts',(94.9225615070513,-26.1476213996829,5.10756229646449));
#21751=CARTESIAN_POINT('Ctrl Pts',(91.7985609777146,-27.6211967303539,4.94957913121586));
#21752=CARTESIAN_POINT('Ctrl Pts',(89.3215407425041,-26.0960765086132,4.81653284812018));
#21753=CARTESIAN_POINT('Ctrl Pts',(88.9319623969259,-24.5369708181419,4.73614762010738));
#21754=CARTESIAN_POINT('Ctrl Pts',(88.9312807091126,-23.9995675532497,4.70842344717745));
#21755=CARTESIAN_POINT('Ctrl Pts',(88.929838025779,-23.9979746552741,5.79157655282255));
#21756=CARTESIAN_POINT('Ctrl Pts',(88.9275818676586,-23.6293267200531,5.77253588131065));
#21757=CARTESIAN_POINT('Ctrl Pts',(89.1590710242286,-22.2438421434169,5.70083415471588));
#21758=CARTESIAN_POINT('Ctrl Pts',(91.2111785923562,-20.4600285259192,5.57647137303824));
#21759=CARTESIAN_POINT('Ctrl Pts',(94.53354332288,-21.4048515492551,5.4184882077896));
#21760=CARTESIAN_POINT('Ctrl Pts',(95.5578977842681,-24.7035627953589,5.26050504254097));
#21761=CARTESIAN_POINT('Ctrl Pts',(93.3551175166525,-27.3641185720073,5.10252187729233));
#21762=CARTESIAN_POINT('Ctrl Pts',(89.9595570406981,-26.9774442566838,4.94621238071953));
#21763=CARTESIAN_POINT('Ctrl Pts',(88.924193406317,-24.9798034901964,4.8425639392296));
#21764=CARTESIAN_POINT('Ctrl Pts',(88.9216167340283,-23.9994167252631,4.79157655282255));
#21765=CARTESIAN_POINT('Origin',(92.,-24.,12.2084234471775));
#21766=CARTESIAN_POINT('',(88.9285850678455,-24.0025047919022,6.79157655282255));
#21767=CARTESIAN_POINT('',(88.9234957058127,-23.9978813008156,6.70842344717745));
#21768=CARTESIAN_POINT('',(88.9265,-23.9999999999999,12.2084234471775));
#21769=CARTESIAN_POINT('Ctrl Pts',(88.9234957058127,-23.9978813008156,6.70842344717746));
#21770=CARTESIAN_POINT('Ctrl Pts',(88.9224297712393,-23.862878283601,6.70141361443525));
#21771=CARTESIAN_POINT('Ctrl Pts',(88.9915973803182,-22.7147700696948,6.64174272661017));
#21772=CARTESIAN_POINT('Ctrl Pts',(90.4354576201273,-20.7280203884636,6.52941078370221));
#21773=CARTESIAN_POINT('Ctrl Pts',(93.8851898408184,-20.9016612993894,6.37142761845357));
#21774=CARTESIAN_POINT('Ctrl Pts',(95.6249905303983,-23.885601165237,6.21344445320494));
#21775=CARTESIAN_POINT('Ctrl Pts',(94.0768010801705,-26.9733046786334,6.0554612879563));
#21776=CARTESIAN_POINT('Ctrl Pts',(90.6448821645723,-27.3641193633755,5.89747812270767));
#21777=CARTESIAN_POINT('Ctrl Pts',(89.031950207745,-25.4159924901842,5.78179884244805));
#21778=CARTESIAN_POINT('Ctrl Pts',(88.9235062815685,-24.2024076976298,5.71878061727132));
#21779=CARTESIAN_POINT('Ctrl Pts',(88.9253102843548,-24.0026322735621,5.70842344717746));
#21780=CARTESIAN_POINT('Ctrl Pts',(88.9285850678455,-24.0025047919022,6.79157655282255));
#21781=CARTESIAN_POINT('Ctrl Pts',(88.934071295281,-23.2983382673306,6.75516887847459));
#21782=CARTESIAN_POINT('Ctrl Pts',(89.5231707262624,-21.5673495506398,6.66610014904376));
#21783=CARTESIAN_POINT('Ctrl Pts',(92.3913282089151,-20.3943794585145,6.52437036453004));
#21784=CARTESIAN_POINT('Ctrl Pts',(95.2334540881775,-22.3573156385801,6.36638719928141));
#21785=CARTESIAN_POINT('Ctrl Pts',(95.1427267432077,-25.8102226011645,6.20840403403277));
#21786=CARTESIAN_POINT('Ctrl Pts',(92.2014389749,-27.6211958785123,6.05042086878414));
#21787=CARTESIAN_POINT('Ctrl Pts',(89.4539543223964,-26.3252211924294,5.9114783750474));
#21788=CARTESIAN_POINT('Ctrl Pts',(88.933821756151,-24.6489015397087,5.82519693639353));
#21789=CARTESIAN_POINT('Ctrl Pts',(88.929838025779,-23.9979746552741,5.79157655282255));
#21790=CARTESIAN_POINT('Origin',(92.,-24.,12.2084234471775));
#21791=CARTESIAN_POINT('',(88.9215398120818,-23.9996098254745,7.79157655282255));
#21792=CARTESIAN_POINT('',(88.931225699577,-23.9993961639011,7.70842344717745));
#21793=CARTESIAN_POINT('',(88.9265,-23.9999999999999,12.2084234471775));
#21794=CARTESIAN_POINT('Ctrl Pts',(88.931225699577,-23.9993961639011,7.70842344717745));
#21795=CARTESIAN_POINT('Ctrl Pts',(88.9303878819455,-23.526898594714,7.68404661159918));
#21796=CARTESIAN_POINT('Ctrl Pts',(89.2544810105531,-22.0347579248864,7.60700872093804));
#21797=CARTESIAN_POINT('Ctrl Pts',(91.5706310054557,-20.3987105715367,7.47730977519401));
#21798=CARTESIAN_POINT('Ctrl Pts',(94.7813299086865,-21.6723730071853,7.31932660994538));
#21799=CARTESIAN_POINT('Ctrl Pts',(95.4692676579736,-25.0572726103797,7.16134344469675));
#21800=CARTESIAN_POINT('Ctrl Pts',(93.0104612250053,-27.483189850294,7.00336027944811));
#21801=CARTESIAN_POINT('Ctrl Pts',(89.7848978894953,-26.7822789631047,6.85238694694168));
#21802=CARTESIAN_POINT('Ctrl Pts',(88.9304375570666,-24.8770824147627,6.75407466951813));
#21803=CARTESIAN_POINT('Ctrl Pts',(88.9234957058127,-23.9978813008156,6.70842344717746));
#21804=CARTESIAN_POINT('Ctrl Pts',(88.9215398120818,-23.9996098254745,7.79157655282255));
#21805=CARTESIAN_POINT('Ctrl Pts',(88.921501203685,-23.9781985065647,7.79046293072141));
#21806=CARTESIAN_POINT('Ctrl Pts',(88.9313646122183,-22.9443234457007,7.73668825353739));
#21807=CARTESIAN_POINT('Ctrl Pts',(90.0822083770022,-20.9217356813897,7.63025252127048));
#21808=CARTESIAN_POINT('Ctrl Pts',(93.5299143458989,-20.7116874252053,7.47226935602185));
#21809=CARTESIAN_POINT('Ctrl Pts',(95.5899360110292,-23.4842511522573,7.31428619077322));
#21810=CARTESIAN_POINT('Ctrl Pts',(94.3937630706594,-26.7246165699189,7.15630302552457));
#21811=CARTESIAN_POINT('Ctrl Pts',(91.0263653754403,-27.4936618194068,6.99831986027595));
#21812=CARTESIAN_POINT('Ctrl Pts',(89.1145964666983,-25.6468831586791,6.87674436937527));
#21813=CARTESIAN_POINT('Ctrl Pts',(88.9261358659971,-24.3168639711034,6.80782993355747));
#21814=CARTESIAN_POINT('Ctrl Pts',(88.9285850678455,-24.0025047919022,6.79157655282255));
#21815=CARTESIAN_POINT('Origin',(92.,-24.,12.2084234471775));
#21816=CARTESIAN_POINT('',(88.9296146841086,-23.99786424691,8.79157655282255));
#21817=CARTESIAN_POINT('',(88.925632185667,-24.0026790855389,8.70842344717746));
#21818=CARTESIAN_POINT('',(88.9265,-23.9999999999999,12.2084234471775));
#21819=CARTESIAN_POINT('Ctrl Pts',(88.925632185667,-24.0026790855389,8.70842344717745));
#21820=CARTESIAN_POINT('Ctrl Pts',(88.9329424382585,-23.1972814204421,8.66667960876312));
#21821=CARTESIAN_POINT('Ctrl Pts',(89.6680869085145,-21.3640271254411,8.57227471526591));
#21822=CARTESIAN_POINT('Ctrl Pts',(92.7514084034007,-20.4518993616932,8.42520876668581));
#21823=CARTESIAN_POINT('Ctrl Pts',(95.38206161577,-22.6903039066152,8.26722560143718));
#21824=CARTESIAN_POINT('Ctrl Pts',(94.9450699403021,-26.1166502818288,8.10924243618855));
#21825=CARTESIAN_POINT('Ctrl Pts',(91.8367990946118,-27.6231212490059,7.95125927093992));
#21826=CARTESIAN_POINT('Ctrl Pts',(89.3333230992967,-26.1179253063225,7.81765294126955));
#21827=CARTESIAN_POINT('Ctrl Pts',(88.9321978117167,-24.5476307745572,7.73670766668206));
#21828=CARTESIAN_POINT('Ctrl Pts',(88.931225699577,-23.9993961639011,7.70842344717745));
#21829=CARTESIAN_POINT('Ctrl Pts',(88.9296146841086,-23.99786424691,8.79157655282255));
#21830=CARTESIAN_POINT('Ctrl Pts',(88.9272864716551,-23.6401225112663,8.77309592788534));
#21831=CARTESIAN_POINT('Ctrl Pts',(89.149833727977,-22.265786270585,8.70195424786526));
#21832=CARTESIAN_POINT('Ctrl Pts',(91.1738623478633,-20.4685627419331,8.57815151276229));
#21833=CARTESIAN_POINT('Ctrl Pts',(94.5060020988175,-21.3782461595948,8.42016834751366));
#21834=CARTESIAN_POINT('Ctrl Pts',(95.5651288739418,-24.665967239189,8.26218518226502));
#21835=CARTESIAN_POINT('Ctrl Pts',(93.3905540118639,-27.3496247591347,8.10420201701638));
#21836=CARTESIAN_POINT('Ctrl Pts',(89.9789224334285,-26.9975617834284,7.94733247386889));
#21837=CARTESIAN_POINT('Ctrl Pts',(88.9233269207872,-24.9906987464103,7.84312398580428));
#21838=CARTESIAN_POINT('Ctrl Pts',(88.9215398120818,-23.9996098254745,7.79157655282255));
#21839=CARTESIAN_POINT('Origin',(92.,-24.,12.2084234471775));
#21840=CARTESIAN_POINT('',(88.9297109890477,-24.0031050978172,9.79157655282255));
#21841=CARTESIAN_POINT('',(88.9232328435277,-23.9980626432726,9.70842344717746));
#21842=CARTESIAN_POINT('',(88.9265,-23.9999999999999,12.2084234471775));
#21843=CARTESIAN_POINT('',(91.2062007174671,-26.9692229537457,10.));
#21844=CARTESIAN_POINT('Ctrl Pts',(91.2062007174671,-26.9692229537457,10.));
#21845=CARTESIAN_POINT('Ctrl Pts',(90.2237466982397,-26.7065713079336,9.94733894491712));
#21846=CARTESIAN_POINT('Ctrl Pts',(89.1240889563566,-25.6687841901452,9.87786446252464));
#21847=CARTESIAN_POINT('Ctrl Pts',(88.9273641407895,-24.3283664602092,9.80838998013216));
#21848=CARTESIAN_POINT('Ctrl Pts',(88.9297109890477,-24.0031050978172,9.79157655282255));
#21849=CARTESIAN_POINT('',(92.7956974280508,-26.974301052007,10.));
#21850=CARTESIAN_POINT('Origin',(92.,-24.,10.));
#21851=CARTESIAN_POINT('Ctrl Pts',(92.7957018439802,-26.9743128659187,10.));
#21852=CARTESIAN_POINT('Ctrl Pts',(91.8480947973977,-27.2254055278759,9.94901908464117));
#21853=CARTESIAN_POINT('Ctrl Pts',(89.7874433743318,-26.7696547721755,9.85182690036699));
#21854=CARTESIAN_POINT('Ctrl Pts',(88.9299259678011,-24.8876740595768,9.75463471609281));
#21855=CARTESIAN_POINT('Ctrl Pts',(88.9232328435277,-23.9980626432726,9.70842344717746));
#21856=CARTESIAN_POINT('Origin',(24.,92.,5.));
#21857=CARTESIAN_POINT('',(21.4865042982783,92.0002742229179,1.38741669750802));
#21858=CARTESIAN_POINT('',(21.4843731420169,91.9964690566784,1.11258330249198));
#21859=CARTESIAN_POINT('',(21.4825,92.,5.));
#21860=CARTESIAN_POINT('',(22.086534003335,93.635987203375,0.999999999999999));
#21861=CARTESIAN_POINT('Ctrl Pts',(21.4843731420169,91.9964690566784,1.11258330249198));
#21862=CARTESIAN_POINT('Ctrl Pts',(21.4895360512898,92.5890870308544,1.07505553499465));
#21863=CARTESIAN_POINT('Ctrl Pts',(21.700778171916,93.1848035603045,1.03752776749732));
#21864=CARTESIAN_POINT('Ctrl Pts',(22.086534003335,93.635987203375,0.99999999999999));
#21865=CARTESIAN_POINT('',(21.4825,92.,1.));
#21866=CARTESIAN_POINT('Origin',(24.,92.,1.));
#21867=CARTESIAN_POINT('',(21.4825,92.,0.));
#21868=CARTESIAN_POINT('',(21.4825,92.,5.));
#21869=CARTESIAN_POINT('Origin',(24.,92.,0.));
#21870=CARTESIAN_POINT('',(25.917103468466,93.6385343514563,0.999999999999998));
#21871=CARTESIAN_POINT('Origin',(24.,92.,1.));
#21872=CARTESIAN_POINT('Ctrl Pts',(25.9171119325404,93.6385402784441,0.999999999999998));
#21873=CARTESIAN_POINT('Ctrl Pts',(25.393957270488,94.247695615171,1.05098091535882));
#21874=CARTESIAN_POINT('Ctrl Pts',(24.5534188240449,94.5878280192362,1.10196183071765));
#21875=CARTESIAN_POINT('Ctrl Pts',(23.7542642184068,94.50948576913,1.15294274607647));
#21876=CARTESIAN_POINT('Ctrl Pts',(22.9287724748585,94.4285616523478,1.20560380115935));
#21877=CARTESIAN_POINT('Ctrl Pts',(22.1474372319946,93.9011256605461,1.25826485624223));
#21878=CARTESIAN_POINT('Ctrl Pts',(21.7641117257107,93.1658537555941,1.31092591132511));
#21879=CARTESIAN_POINT('Ctrl Pts',(21.5785168283464,92.8098567987064,1.33642284005274));
#21880=CARTESIAN_POINT('Ctrl Pts',(21.4862237958222,92.4051387264905,1.36191976878038));
#21881=CARTESIAN_POINT('Ctrl Pts',(21.4865042982783,92.0002742229179,1.38741669750802));
#21882=CARTESIAN_POINT('Origin',(24.,92.,5.));
#21883=CARTESIAN_POINT('',(21.4812641621455,91.9978903848741,2.38741669750802));
#21884=CARTESIAN_POINT('',(21.4785876236681,92.0006455599548,2.11258330249197));
#21885=CARTESIAN_POINT('',(21.4825,92.,5.));
#21886=CARTESIAN_POINT('Ctrl Pts',(21.4785876236681,92.0006455599548,2.11258330249197));
#21887=CARTESIAN_POINT('Ctrl Pts',(21.4784679588297,92.0358286254365,2.11034958724146));
#21888=CARTESIAN_POINT('Ctrl Pts',(21.4791412415305,92.071006953815,2.10811587199095));
#21889=CARTESIAN_POINT('Ctrl Pts',(21.480621792432,92.1061512101347,2.10588215674043));
#21890=CARTESIAN_POINT('Ctrl Pts',(21.5155265872823,92.9346962171463,2.05322110165756));
#21891=CARTESIAN_POINT('Ctrl Pts',(21.9991161631697,93.7443037579804,2.00056004657468));
#21892=CARTESIAN_POINT('Ctrl Pts',(22.7120874500748,94.1678867011383,1.9478989914918));
#21893=CARTESIAN_POINT('Ctrl Pts',(23.4250587369799,94.5914696442962,1.89523793640892));
#21894=CARTESIAN_POINT('Ctrl Pts',(24.3674117349026,94.6290279897781,1.84257688132604));
#21895=CARTESIAN_POINT('Ctrl Pts',(25.1117466201968,94.2633574548232,1.78991582624316));
#21896=CARTESIAN_POINT('Ctrl Pts',(25.8560815054909,93.8976869198683,1.73725477116029));
#21897=CARTESIAN_POINT('Ctrl Pts',(26.4023982781565,93.1287875044767,1.68459371607741));
#21898=CARTESIAN_POINT('Ctrl Pts',(26.5029873847571,92.3057173158972,1.63193266099453));
#21899=CARTESIAN_POINT('Ctrl Pts',(26.6035764913577,91.4826471273178,1.57927160591165));
#21900=CARTESIAN_POINT('Ctrl Pts',(26.2584379318934,90.6054061655505,1.52661055082877));
#21901=CARTESIAN_POINT('Ctrl Pts',(25.6239876980049,90.0711235918099,1.4739494957459));
#21902=CARTESIAN_POINT('Ctrl Pts',(24.9895374641163,89.5368410180693,1.42128844066302));
#21903=CARTESIAN_POINT('Ctrl Pts',(24.0657755558035,89.3455168323553,1.36862738558014));
#21904=CARTESIAN_POINT('Ctrl Pts',(23.2718708195104,89.5853896272901,1.31596633049726));
#21905=CARTESIAN_POINT('Ctrl Pts',(22.4779660832173,89.8252624222249,1.26330527541438));
#21906=CARTESIAN_POINT('Ctrl Pts',(21.8139185189438,90.4963321978086,1.2106442203315));
#21907=CARTESIAN_POINT('Ctrl Pts',(21.5807319779765,91.2907318840647,1.15798316524862));
#21908=CARTESIAN_POINT('Ctrl Pts',(21.5137208066282,91.5190197315273,1.14284987766308));
#21909=CARTESIAN_POINT('Ctrl Pts',(21.4822911692267,91.7574924580249,1.12771659007753));
#21910=CARTESIAN_POINT('Ctrl Pts',(21.4843731420169,91.9964690566784,1.11258330249198));
#21911=CARTESIAN_POINT('Ctrl Pts',(21.4865042982783,92.0002742229179,1.38741669750802));
#21912=CARTESIAN_POINT('Ctrl Pts',(21.486803142278,91.5689363684933,1.41458082386326));
#21913=CARTESIAN_POINT('Ctrl Pts',(21.5921777588412,91.1374323068698,1.4417449502185));
#21914=CARTESIAN_POINT('Ctrl Pts',(21.8017473998347,90.764501991722,1.46890907657374));
#21915=CARTESIAN_POINT('Ctrl Pts',(22.2080243499465,90.0415299509042,1.52157013165662));
#21916=CARTESIAN_POINT('Ctrl Pts',(23.0058940198741,89.5386936873713,1.5742311867395));
#21917=CARTESIAN_POINT('Ctrl Pts',(23.833390176038,89.4839126258589,1.62689224182238));
#21918=CARTESIAN_POINT('Ctrl Pts',(24.6608863322019,89.4291315643466,1.67955329690525));
#21919=CARTESIAN_POINT('Ctrl Pts',(25.5180089746021,89.8224057048548,1.73221435198813));
#21920=CARTESIAN_POINT('Ctrl Pts',(26.0160964783391,90.4854399019793,1.78487540707101));
#21921=CARTESIAN_POINT('Ctrl Pts',(26.5141839820761,91.1484740991038,1.83753646215389));
#21922=CARTESIAN_POINT('Ctrl Pts',(26.6532363471501,92.0812683528444,1.89019751723676));
#21923=CARTESIAN_POINT('Ctrl Pts',(26.3701624990712,92.8607544964156,1.94285857231964));
#21924=CARTESIAN_POINT('Ctrl Pts',(26.0870886509923,93.6402406399867,1.99551962740252));
#21925=CARTESIAN_POINT('Ctrl Pts',(25.3818885897605,94.2664186733884,2.0481806824854));
#21926=CARTESIAN_POINT('Ctrl Pts',(24.5743965080577,94.4553208851494,2.10084173756828));
#21927=CARTESIAN_POINT('Ctrl Pts',(23.7669044263549,94.6442230969105,2.15350279265116));
#21928=CARTESIAN_POINT('Ctrl Pts',(22.857120324181,94.3958494870309,2.20616384773403));
#21929=CARTESIAN_POINT('Ctrl Pts',(22.2576399987561,93.8228345233925,2.25882490281691));
#21930=CARTESIAN_POINT('Ctrl Pts',(21.7696876855645,93.3564239255092,2.30168883438062));
#21931=CARTESIAN_POINT('Ctrl Pts',(21.4873206236216,92.6749290158026,2.34455276594432));
#21932=CARTESIAN_POINT('Ctrl Pts',(21.4812641621455,91.9978903848741,2.38741669750802));
#21933=CARTESIAN_POINT('Origin',(24.,92.,5.));
#21934=CARTESIAN_POINT('',(21.4802712114252,92.0018289507128,3.38741669750802));
#21935=CARTESIAN_POINT('',(21.4854088326161,92.0015585716341,3.11258330249198));
#21936=CARTESIAN_POINT('',(21.4825,92.,5.));
#21937=CARTESIAN_POINT('Ctrl Pts',(21.4854088326161,92.0015585716341,3.11258330249198));
#21938=CARTESIAN_POINT('Ctrl Pts',(21.4836296984461,92.3124536014081,3.0929825844054));
#21939=CARTESIAN_POINT('Ctrl Pts',(21.5370773572355,92.6227586333046,3.07338186631882));
#21940=CARTESIAN_POINT('Ctrl Pts',(21.6485419638298,92.910596671031,3.05378114823224));
#21941=CARTESIAN_POINT('Ctrl Pts',(21.9480128179958,93.6839282751438,3.00112009314936));
#21942=CARTESIAN_POINT('Ctrl Pts',(22.666267618347,94.2950862932019,2.94845903806648));
#21943=CARTESIAN_POINT('Ctrl Pts',(23.4775657352139,94.4669012884929,2.8957979829836));
#21944=CARTESIAN_POINT('Ctrl Pts',(24.2888638520808,94.638716283784,2.84313692790073));
#21945=CARTESIAN_POINT('Ctrl Pts',(25.1932052854634,94.371188256308,2.79047587281785));
#21946=CARTESIAN_POINT('Ctrl Pts',(25.7804553940472,93.7856433745946,2.73781481773497));
#21947=CARTESIAN_POINT('Ctrl Pts',(26.367705502631,93.2000984928813,2.68515376265209));
#21948=CARTESIAN_POINT('Ctrl Pts',(26.6378642864159,92.2965367569306,2.63249270756921));
#21949=CARTESIAN_POINT('Ctrl Pts',(26.4684108772915,91.4847436484407,2.57983165248634));
#21950=CARTESIAN_POINT('Ctrl Pts',(26.2989574681671,90.6729505399509,2.52717059740346));
#21951=CARTESIAN_POINT('Ctrl Pts',(25.6898918661334,89.9529260589219,2.47450954232058));
#21952=CARTESIAN_POINT('Ctrl Pts',(24.9174341827592,89.6512037648828,2.4218484872377));
#21953=CARTESIAN_POINT('Ctrl Pts',(24.1449764993849,89.3494814708436,2.36918743215482));
#21954=CARTESIAN_POINT('Ctrl Pts',(23.2091267346701,89.4660613637943,2.31652637707195));
#21955=CARTESIAN_POINT('Ctrl Pts',(22.5343118592193,89.9480925468641,2.26386532198907));
#21956=CARTESIAN_POINT('Ctrl Pts',(21.8881204945621,90.4096774930869,2.2134379821567));
#21957=CARTESIAN_POINT('Ctrl Pts',(21.4812891226481,91.2063686712679,2.16301064232434));
#21958=CARTESIAN_POINT('Ctrl Pts',(21.4785876236681,92.0006455599548,2.11258330249197));
#21959=CARTESIAN_POINT('Ctrl Pts',(21.4812641621455,91.9978903848741,2.38741669750802));
#21960=CARTESIAN_POINT('Ctrl Pts',(21.47987987706,91.8431441716248,2.3972138210272));
#21961=CARTESIAN_POINT('Ctrl Pts',(21.492930389882,91.6886307597355,2.40701094454637));
#21962=CARTESIAN_POINT('Ctrl Pts',(21.5212601912555,91.5369715569028,2.41680806806554));
#21963=CARTESIAN_POINT('Ctrl Pts',(21.6735372578557,90.7217798714484,2.46946912314842));
#21964=CARTESIAN_POINT('Ctrl Pts',(22.2672679397321,89.9890528179368,2.5221301782313));
#21965=CARTESIAN_POINT('Ctrl Pts',(23.0331836055545,89.6710928935685,2.57479123331418));
#21966=CARTESIAN_POINT('Ctrl Pts',(23.7990992713769,89.3531329692002,2.62745228839706));
#21967=CARTESIAN_POINT('Ctrl Pts',(24.7371999211453,89.4499401739752,2.68011334347994));
#21968=CARTESIAN_POINT('Ctrl Pts',(25.4220417006604,89.9176116335594,2.73277439856282));
#21969=CARTESIAN_POINT('Ctrl Pts',(26.1068834801755,90.3852830931436,2.78543545364569));
#21970=CARTESIAN_POINT('Ctrl Pts',(26.5384663894374,91.2238188075369,2.83809650872857));
#21971=CARTESIAN_POINT('Ctrl Pts',(26.5210598219411,92.052928105998,2.89075756381145));
#21972=CARTESIAN_POINT('Ctrl Pts',(26.5036532544449,92.8820374044591,2.94341861889433));
#21973=CARTESIAN_POINT('Ctrl Pts',(26.0372572101906,93.701720286988,2.99607967397721));
#21974=CARTESIAN_POINT('Ctrl Pts',(25.3333904465718,94.1402367801487,3.04874072906008));
#21975=CARTESIAN_POINT('Ctrl Pts',(24.6295236829529,94.5787532733095,3.10140178414296));
#21976=CARTESIAN_POINT('Ctrl Pts',(23.6881861999696,94.636103377102,3.15406283922584));
#21977=CARTESIAN_POINT('Ctrl Pts',(22.9362905172017,94.2862777415509,3.20672389430872));
#21978=CARTESIAN_POINT('Ctrl Pts',(22.1843948344338,93.9364521059997,3.2593849493916));
#21979=CARTESIAN_POINT('Ctrl Pts',(21.6219409518813,93.1794507311049,3.31204600447447));
#21980=CARTESIAN_POINT('Ctrl Pts',(21.5040113501232,92.3585867079682,3.36470705955735));
#21981=CARTESIAN_POINT('Ctrl Pts',(21.4870592998501,92.2405898015078,3.37227693887424));
#21982=CARTESIAN_POINT('Ctrl Pts',(21.4792925695015,92.1212732846669,3.37984681819113));
#21983=CARTESIAN_POINT('Ctrl Pts',(21.4802712114252,92.0018289507128,3.38741669750802));
#21984=CARTESIAN_POINT('Origin',(24.,92.,5.));
#21985=CARTESIAN_POINT('',(21.4864157451591,92.0003542166096,4.38741669750802));
#21986=CARTESIAN_POINT('',(21.4839748093506,91.9978936309448,4.11258330249198));
#21987=CARTESIAN_POINT('',(21.4825,92.,5.));
#21988=CARTESIAN_POINT('Ctrl Pts',(21.4839748093506,91.9978936309448,4.11258330249198));
#21989=CARTESIAN_POINT('Ctrl Pts',(21.4886914413751,92.5834107418754,4.07561558156933));
#21990=CARTESIAN_POINT('Ctrl Pts',(21.6925942792402,93.1718904338738,4.03864786064669));
#21991=CARTESIAN_POINT('Ctrl Pts',(22.0662148873617,93.6183374708837,4.00168013972404));
#21992=CARTESIAN_POINT('Ctrl Pts',(22.5984428671594,94.2543077557916,3.94901908464117));
#21993=CARTESIAN_POINT('Ctrl Pts',(23.4750692077561,94.6020594676884,3.89635802955829));
#21994=CARTESIAN_POINT('Ctrl Pts',(24.298528905607,94.5038812863977,3.84369697447541));
#21995=CARTESIAN_POINT('Ctrl Pts',(25.1219886034578,94.4057031051071,3.79103591939254));
#21996=CARTESIAN_POINT('Ctrl Pts',(25.8922816585629,93.8615950306291,3.73837486430965));
#21997=CARTESIAN_POINT('Ctrl Pts',(26.2600670194834,93.1183193280088,3.68571380922678));
#21998=CARTESIAN_POINT('Ctrl Pts',(26.6278523804038,92.3750436253885,3.6330527541439));
#21999=CARTESIAN_POINT('Ctrl Pts',(26.5931300471397,91.4326002946258,3.58039169906102));
#22000=CARTESIAN_POINT('Ctrl Pts',(26.1716472007571,90.7184035364296,3.52773064397814));
#22001=CARTESIAN_POINT('Ctrl Pts',(25.7501643543746,90.0042067782334,3.47506958889527));
#22002=CARTESIAN_POINT('Ctrl Pts',(24.9419209948735,89.5182565926036,3.42240853381239));
#22003=CARTESIAN_POINT('Ctrl Pts',(24.113469258178,89.4809395463902,3.36974747872951));
#22004=CARTESIAN_POINT('Ctrl Pts',(23.2850175214824,89.4436225001769,3.31708642364663));
#22005=CARTESIAN_POINT('Ctrl Pts',(22.4363574075923,89.85493859338,3.26442536856375));
#22006=CARTESIAN_POINT('Ctrl Pts',(21.9523708046376,90.5283492350653,3.21176431348087));
#22007=CARTESIAN_POINT('Ctrl Pts',(21.6485265278719,90.9511129399696,3.17870397648458));
#22008=CARTESIAN_POINT('Ctrl Pts',(21.4884096805934,91.4771750052055,3.14564363948828));
#22009=CARTESIAN_POINT('Ctrl Pts',(21.4854088326161,92.0015585716341,3.11258330249198));
#22010=CARTESIAN_POINT('Ctrl Pts',(21.4802712114252,92.0018289507128,3.38741669750802));
#22011=CARTESIAN_POINT('Ctrl Pts',(21.4861006458386,91.2903400047059,3.43250787327401));
#22012=CARTESIAN_POINT('Ctrl Pts',(21.8022313189484,90.5743158820022,3.47759904904));
#22013=CARTESIAN_POINT('Ctrl Pts',(22.335679104099,90.105645314345,3.52269022480599));
#22014=CARTESIAN_POINT('Ctrl Pts',(22.9586817807967,89.5582946152369,3.57535127988887));
#22015=CARTESIAN_POINT('Ctrl Pts',(23.8780924551558,89.3483198883991,3.62801233497174));
#22016=CARTESIAN_POINT('Ctrl Pts',(24.6769427066419,89.5709482675317,3.68067339005462));
#22017=CARTESIAN_POINT('Ctrl Pts',(25.475792958128,89.7935766466644,3.7333344451375));
#22018=CARTESIAN_POINT('Ctrl Pts',(26.154082786741,90.4488081317675,3.78599550022038));
#22019=CARTESIAN_POINT('Ctrl Pts',(26.4041961740691,91.2394840564229,3.83865655530326));
#22020=CARTESIAN_POINT('Ctrl Pts',(26.6543095613971,92.0301599810783,3.89131761038613));
#22021=CARTESIAN_POINT('Ctrl Pts',(26.4762465074402,92.9562803452861,3.94397866546901));
#22022=CARTESIAN_POINT('Ctrl Pts',(25.9507616486448,93.59783376143,3.99663972055189));
#22023=CARTESIAN_POINT('Ctrl Pts',(25.4252767898494,94.239387177574,4.04930077563477));
#22024=CARTESIAN_POINT('Ctrl Pts',(24.5523701262155,94.596373645654,4.10196183071765));
#22025=CARTESIAN_POINT('Ctrl Pts',(23.7279197254965,94.5068937086739,4.15462288580053));
#22026=CARTESIAN_POINT('Ctrl Pts',(22.9034693247774,94.4174137716938,4.2072839408834));
#22027=CARTESIAN_POINT('Ctrl Pts',(22.1274751869732,93.8814674296536,4.25994499596628));
#22028=CARTESIAN_POINT('Ctrl Pts',(21.7518638973824,93.1421154958358,4.31260605104916));
#22029=CARTESIAN_POINT('Ctrl Pts',(21.5739985954225,92.7920060646031,4.33754293320211));
#22030=CARTESIAN_POINT('Ctrl Pts',(21.4859135120177,92.3962857922303,4.36247981535507));
#22031=CARTESIAN_POINT('Ctrl Pts',(21.4864157451591,92.0003542166096,4.38741669750802));
#22032=CARTESIAN_POINT('Origin',(24.,92.,5.));
#22033=CARTESIAN_POINT('',(21.4815253774702,91.9978439079131,5.38741669750803));
#22034=CARTESIAN_POINT('',(21.4784999401586,92.000477759641,5.11258330249198));
#22035=CARTESIAN_POINT('',(21.4825,92.,5.));
#22036=CARTESIAN_POINT('Ctrl Pts',(21.4784999401586,92.000477759641,5.11258330249198));
#22037=CARTESIAN_POINT('Ctrl Pts',(21.4784306610618,92.0268374600631,5.11090963381615));
#22038=CARTESIAN_POINT('Ctrl Pts',(21.478808621275,92.0531951260584,5.10923596514032));
#22039=CARTESIAN_POINT('Ctrl Pts',(21.4796399750105,92.0795384836879,5.10756229646448));
#22040=CARTESIAN_POINT('Ctrl Pts',(21.5057980584424,92.9084175965176,5.05490124138161));
#22041=CARTESIAN_POINT('Ctrl Pts',(21.9808208362983,93.7231312660315,5.00224018629873));
#22042=CARTESIAN_POINT('Ctrl Pts',(22.6892773720314,94.1541929390351,4.94957913121586));
#22043=CARTESIAN_POINT('Ctrl Pts',(23.3977339077645,94.5852546120388,4.89691807613298));
#22044=CARTESIAN_POINT('Ctrl Pts',(24.3396242013747,94.6326642885323,4.8442570210501));
#22045=CARTESIAN_POINT('Ctrl Pts',(25.0877849303764,94.2749208713486,4.79159596596722));
#22046=CARTESIAN_POINT('Ctrl Pts',(25.8359456593782,93.9171774541649,4.73893491088434));
#22047=CARTESIAN_POINT('Ctrl Pts',(26.3903768237716,93.154280943304,4.68627385580146));
#22048=CARTESIAN_POINT('Ctrl Pts',(26.4996344284722,92.3322179256394,4.63361280071859));
#22049=CARTESIAN_POINT('Ctrl Pts',(26.6088920331728,91.5101549079748,4.58095174563571));
#22050=CARTESIAN_POINT('Ctrl Pts',(26.2729760781807,90.6289253835065,4.52829069055283));
#22051=CARTESIAN_POINT('Ctrl Pts',(25.6442301819934,90.0881819816232,4.47562963546995));
#22052=CARTESIAN_POINT('Ctrl Pts',(25.0154842858061,89.5474385797398,4.42296858038707));
#22053=CARTESIAN_POINT('Ctrl Pts',(24.0939084484235,89.3471813004415,4.37030752530419));
#22054=CARTESIAN_POINT('Ctrl Pts',(23.2974530394866,89.5782302356247,4.31764647022132));
#22055=CARTESIAN_POINT('Ctrl Pts',(22.5009976305496,89.8092791708079,4.26498541513844));
#22056=CARTESIAN_POINT('Ctrl Pts',(21.8296626500581,90.4716343204728,4.21232436005556));
#22057=CARTESIAN_POINT('Ctrl Pts',(21.5879099693117,91.2649063242647,4.15966330497268));
#22058=CARTESIAN_POINT('Ctrl Pts',(21.5158661107693,91.5013064992303,4.14396997081245));
#22059=CARTESIAN_POINT('Ctrl Pts',(21.481972530589,91.749333117907,4.12827663665221));
#22060=CARTESIAN_POINT('Ctrl Pts',(21.4839748093506,91.9978936309448,4.11258330249198));
#22061=CARTESIAN_POINT('Ctrl Pts',(21.4864157451591,92.0003542166096,4.38741669750802));
#22062=CARTESIAN_POINT('Ctrl Pts',(21.4869741148212,91.5601678531502,4.41514087043795));
#22063=CARTESIAN_POINT('Ctrl Pts',(21.5970300437705,91.1197203102036,4.44286504336787));
#22064=CARTESIAN_POINT('Ctrl Pts',(21.8149442483521,90.7413995457469,4.47058921629779));
#22065=CARTESIAN_POINT('Ctrl Pts',(22.2288643302899,90.0227930550715,4.52325027138067));
#22066=CARTESIAN_POINT('Ctrl Pts',(23.0319329355429,89.5283375993164,4.57591132646355));
#22067=CARTESIAN_POINT('Ctrl Pts',(23.8599447465539,89.4822771662391,4.62857238154643));
#22068=CARTESIAN_POINT('Ctrl Pts',(24.6879565575648,89.4362167331619,4.68123343662931));
#22069=CARTESIAN_POINT('Ctrl Pts',(25.5409115743339,89.8385513227625,4.73389449171218));
#22070=CARTESIAN_POINT('Ctrl Pts',(26.0319801400904,90.5068153323074,4.78655554679506));
#22071=CARTESIAN_POINT('Ctrl Pts',(26.523048705847,91.1750793418522,4.83921660187794));
#22072=CARTESIAN_POINT('Ctrl Pts',(26.652230820591,92.1092727713413,4.89187765696082));
#22073=CARTESIAN_POINT('Ctrl Pts',(26.3609401906912,92.8857229575282,4.9445387120437));
#22074=CARTESIAN_POINT('Ctrl Pts',(26.0696495607913,93.6621731437152,4.99719976712658));
#22075=CARTESIAN_POINT('Ctrl Pts',(25.3578861862475,94.2808800866,5.04986082220945));
#22076=CARTESIAN_POINT('Ctrl Pts',(24.5484469044027,94.461249628667,5.10252187729233));
#22077=CARTESIAN_POINT('Ctrl Pts',(23.7390076225579,94.641619170734,5.15518293237521));
#22078=CARTESIAN_POINT('Ctrl Pts',(22.8318924334121,94.3836513119832,5.20784398745809));
#22079=CARTESIAN_POINT('Ctrl Pts',(22.2384935561441,93.8043388788684,5.26050504254097));
#22080=CARTESIAN_POINT('Ctrl Pts',(21.7618020463168,93.3389633465204,5.30280892752999));
#22081=CARTESIAN_POINT('Ctrl Pts',(21.4875608688215,92.6662147404431,5.34511281251901));
#22082=CARTESIAN_POINT('Ctrl Pts',(21.4815253774702,91.9978439079131,5.38741669750803));
#22083=CARTESIAN_POINT('Origin',(24.,92.,5.));
#22084=CARTESIAN_POINT('',(21.4800390583838,92.0017354239359,6.38741669750802));
#22085=CARTESIAN_POINT('',(21.4852339904214,92.0016589574482,6.11258330249198));
#22086=CARTESIAN_POINT('',(21.4825,92.,5.));
#22087=CARTESIAN_POINT('Ctrl Pts',(21.4852339904214,92.0016589574482,6.11258330249198));
#22088=CARTESIAN_POINT('Ctrl Pts',(21.4833859739972,92.3036180412943,6.09354263098008));
#22089=CARTESIAN_POINT('Ctrl Pts',(21.5337383064256,92.6049815306727,6.07450195946819));
#22090=CARTESIAN_POINT('Ctrl Pts',(21.6390603134632,92.8857227683913,6.0554612879563));
#22091=CARTESIAN_POINT('Ctrl Pts',(21.930350881161,93.6621727887753,6.00280023287342));
#22092=CARTESIAN_POINT('Ctrl Pts',(22.6421141037151,94.2808795995417,5.95013917779054));
#22093=CARTESIAN_POINT('Ctrl Pts',(23.4515532127125,94.4612491030927,5.89747812270766));
#22094=CARTESIAN_POINT('Ctrl Pts',(24.26099232171,94.6416186066436,5.84481706762478));
#22095=CARTESIAN_POINT('Ctrl Pts',(25.1681073171508,94.3836508029792,5.7921560125419));
#22096=CARTESIAN_POINT('Ctrl Pts',(25.7615060677045,93.8043384935704,5.73949495745902));
#22097=CARTESIAN_POINT('Ctrl Pts',(26.3549048182583,93.2250261841617,5.68683390237615));
#22098=CARTESIAN_POINT('Ctrl Pts',(26.6345873239251,92.3243693690087,5.63417284729327));
#22099=CARTESIAN_POINT('Ctrl Pts',(26.4737127953066,91.5108312844465,5.58151179221039));
#22100=CARTESIAN_POINT('Ctrl Pts',(26.3128382666881,90.6972931998844,5.52885073712751));
#22101=CARTESIAN_POINT('Ctrl Pts',(25.7114067037843,89.9708738459131,5.47618968204463));
#22102=CARTESIAN_POINT('Ctrl Pts',(24.9421775844462,89.6610167966983,5.42352862696176));
#22103=CARTESIAN_POINT('Ctrl Pts',(24.1729484651081,89.3511597474835,5.37086757187888));
#22104=CARTESIAN_POINT('Ctrl Pts',(23.2359217893358,89.4578650030252,5.318206516796));
#22105=CARTESIAN_POINT('Ctrl Pts',(22.5560551459534,89.9327399088688,5.26554546171312));
#22106=CARTESIAN_POINT('Ctrl Pts',(21.8977959599792,90.3925223853337,5.21455807530607));
#22107=CARTESIAN_POINT('Ctrl Pts',(21.4806104893556,91.1974441303419,5.16357068889902));
#22108=CARTESIAN_POINT('Ctrl Pts',(21.4784999401586,92.000477759641,5.11258330249198));
#22109=CARTESIAN_POINT('Ctrl Pts',(21.4815253774702,91.9978439079131,5.38741669750803));
#22110=CARTESIAN_POINT('Ctrl Pts',(21.4800477209727,91.8342080999941,5.39777386760188));
#22111=CARTESIAN_POINT('Ctrl Pts',(21.4946464973945,91.6708346988264,5.40813103769574));
#22112=CARTESIAN_POINT('Ctrl Pts',(21.5262866764575,91.5108311799897,5.4184882077896));
#22113=CARTESIAN_POINT('Ctrl Pts',(21.6871612394291,90.6972929217049,5.47114926287248));
#22114=CARTESIAN_POINT('Ctrl Pts',(22.2885929307624,89.9708734126143,5.52381031795536));
#22115=CARTESIAN_POINT('Ctrl Pts',(23.0578222143614,89.6610162972326,5.57647137303823));
#22116=CARTESIAN_POINT('Ctrl Pts',(23.8270514979604,89.351159181851,5.62913242812111));
#22117=CARTESIAN_POINT('Ctrl Pts',(24.7640783738252,89.4578644601783,5.68179348320399));
#22118=CARTESIAN_POINT('Ctrl Pts',(25.443945162386,89.9327394674266,5.73445453828687));
#22119=CARTESIAN_POINT('Ctrl Pts',(26.1238119509469,90.407614474675,5.78711559336975));
#22120=CARTESIAN_POINT('Ctrl Pts',(26.5465186522039,91.2506592108443,5.83977664845262));
#22121=CARTESIAN_POINT('Ctrl Pts',(26.5203605631863,92.0795385006725,5.8924377035355));
#22122=CARTESIAN_POINT('Ctrl Pts',(26.4942024741688,92.9084177905007,5.94509875861838));
#22123=CARTESIAN_POINT('Ctrl Pts',(26.0191795948766,93.7231316339878,5.99775981370126));
#22124=CARTESIAN_POINT('Ctrl Pts',(25.3107229078599,94.1541933990405,6.05042086878414));
#22125=CARTESIAN_POINT('Ctrl Pts',(24.6022662208433,94.5852551640932,6.10308192386702));
#22126=CARTESIAN_POINT('Ctrl Pts',(23.6603757261022,94.6326648507116,6.1557429789499));
#22127=CARTESIAN_POINT('Ctrl Pts',(22.9122148373384,94.274921357135,6.20840403403277));
#22128=CARTESIAN_POINT('Ctrl Pts',(22.1640539485746,93.9171778635585,6.26106508911565));
#22129=CARTESIAN_POINT('Ctrl Pts',(21.6096226657882,93.154281189787,6.31372614419853));
#22130=CARTESIAN_POINT('Ctrl Pts',(21.5003650377567,92.3322179965802,6.36638719928141));
#22131=CARTESIAN_POINT('Ctrl Pts',(21.4858215065436,92.2227912963587,6.37339703202361));
#22132=CARTESIAN_POINT('Ctrl Pts',(21.4791659526657,92.1123162318432,6.38040686476582));
#22133=CARTESIAN_POINT('Ctrl Pts',(21.4800390583838,92.0017354239359,6.38741669750802));
#22134=CARTESIAN_POINT('Origin',(24.,92.,5.));
#22135=CARTESIAN_POINT('',(21.4863706869161,92.0004946014336,7.38741669750803));
#22136=CARTESIAN_POINT('',(21.4842076940747,91.9979483279393,7.11258330249198));
#22137=CARTESIAN_POINT('',(21.4825,92.,5.));
#22138=CARTESIAN_POINT('Ctrl Pts',(21.4842076940747,91.9979483279393,7.11258330249198));
#22139=CARTESIAN_POINT('Ctrl Pts',(21.4887014564203,92.5747302879618,7.07617562814402));
#22140=CARTESIAN_POINT('Ctrl Pts',(21.6859403589103,93.1542900307673,7.03976795379606));
#22141=CARTESIAN_POINT('Ctrl Pts',(22.0492387679223,93.5978334202261,7.0033602794481));
#22142=CARTESIAN_POINT('Ctrl Pts',(22.5747235145078,94.23938669937,6.95069922436522));
#22143=CARTESIAN_POINT('Ctrl Pts',(23.4476299917374,94.5963730912254,6.89803816928234));
#22144=CARTESIAN_POINT('Ctrl Pts',(24.2720802164026,94.5068931733543,6.84537711419947));
#22145=CARTESIAN_POINT('Ctrl Pts',(25.0965304410678,94.4174132554832,6.79271605911659));
#22146=CARTESIAN_POINT('Ctrl Pts',(25.8725244131687,93.8814670278857,6.74005500403371));
#22147=CARTESIAN_POINT('Ctrl Pts',(26.2481356225521,93.142115251948,6.68739394895083));
#22148=CARTESIAN_POINT('Ctrl Pts',(26.6237468319354,92.4027634760102,6.63473289386796));
#22149=CARTESIAN_POINT('Ctrl Pts',(26.5989752786013,91.4600061517323,6.58207183878508));
#22150=CARTESIAN_POINT('Ctrl Pts',(26.1850552850515,90.7413998145083,6.5294107837022));
#22151=CARTESIAN_POINT('Ctrl Pts',(25.7711352915018,90.0227934772843,6.47674972861932));
#22152=CARTESIAN_POINT('Ctrl Pts',(24.9680668577364,89.5283381271142,6.42408867353644));
#22153=CARTESIAN_POINT('Ctrl Pts',(24.1400552235389,89.4822777038725,6.37142761845356));
#22154=CARTESIAN_POINT('Ctrl Pts',(23.3120435893413,89.4362172806309,6.31876656337069));
#22155=CARTESIAN_POINT('Ctrl Pts',(22.4590887547118,89.8385517843175,6.26610550828781));
#22156=CARTESIAN_POINT('Ctrl Pts',(21.9680202938178,90.5068156511617,6.21344445320493));
#22157=CARTESIAN_POINT('Ctrl Pts',(21.6545075852538,90.9334551762256,6.17982406963395));
#22158=CARTESIAN_POINT('Ctrl Pts',(21.4884970592155,91.4684855231337,6.14620368606296));
#22159=CARTESIAN_POINT('Ctrl Pts',(21.4852339904214,92.0016589574482,6.11258330249198));
#22160=CARTESIAN_POINT('Ctrl Pts',(21.4800390583838,92.0017354239359,6.38741669750802));
#22161=CARTESIAN_POINT('Ctrl Pts',(21.4857251203391,91.2815828562451,6.4330679198487));
#22162=CARTESIAN_POINT('Ctrl Pts',(21.81071724972,90.5569454920104,6.47871914218937));
#22163=CARTESIAN_POINT('Ctrl Pts',(22.3557694668982,90.0881815733762,6.52437036453004));
#22164=CARTESIAN_POINT('Ctrl Pts',(22.9845154973476,89.5474380560209,6.57703141961292));
#22165=CARTESIAN_POINT('Ctrl Pts',(23.906091531523,89.3471807339522,6.6296924746958));
#22166=CARTESIAN_POINT('Ctrl Pts',(24.702547110535,89.578229718477,6.68235352977867));
#22167=CARTESIAN_POINT('Ctrl Pts',(25.4990026895469,89.8092787030018,6.73501458486155));
#22168=CARTESIAN_POINT('Ctrl Pts',(26.1703378133953,90.47163399412,6.78767563994444));
#22169=CARTESIAN_POINT('Ctrl Pts',(26.4120905457653,91.2649061673002,6.84033669502731));
#22170=CARTESIAN_POINT('Ctrl Pts',(26.6538432781353,92.0581783404805,6.89299775011019));
#22171=CARTESIAN_POINT('Ctrl Pts',(26.4660136190269,92.9823673957227,6.94565880519307));
#22172=CARTESIAN_POINT('Ctrl Pts',(25.933785525578,93.6183378164486,6.99831986027595));
#22173=CARTESIAN_POINT('Ctrl Pts',(25.4015574321291,94.2543082371746,7.05098091535882));
#22174=CARTESIAN_POINT('Ctrl Pts',(24.5249309043397,94.6020600233844,7.1036419704417));
#22175=CARTESIAN_POINT('Ctrl Pts',(23.7014710306461,94.5038818211034,7.15630302552458));
#22176=CARTESIAN_POINT('Ctrl Pts',(22.8780111569525,94.4057036188225,7.20896408060746));
#22177=CARTESIAN_POINT('Ctrl Pts',(22.1077179373546,93.8615954280509,7.26162513569034));
#22178=CARTESIAN_POINT('Ctrl Pts',(21.7399324979007,93.1183195667607,7.31428619077322));
#22179=CARTESIAN_POINT('Ctrl Pts',(21.5696843862451,92.7742567022501,7.33866302635149));
#22180=CARTESIAN_POINT('Ctrl Pts',(21.4856844315082,92.3875167881335,7.36303986192976));
#22181=CARTESIAN_POINT('Ctrl Pts',(21.4863706869161,92.0004946014336,7.38741669750803));
#22182=CARTESIAN_POINT('Origin',(24.,92.,5.));
#22183=CARTESIAN_POINT('',(21.481789046694,91.9978055657336,8.38741669750803));
#22184=CARTESIAN_POINT('',(21.4784369335473,92.0003195913806,8.11258330249198));
#22185=CARTESIAN_POINT('',(21.4825,92.,5.));
#22186=CARTESIAN_POINT('Ctrl Pts',(21.4784369335473,92.0003195913806,8.11258330249198));
#22187=CARTESIAN_POINT('Ctrl Pts',(21.4784053094568,92.0178575771478,8.11146968039083));
#22188=CARTESIAN_POINT('Ctrl Pts',(21.4785726200147,92.0353949438105,8.11035605828969));
#22189=CARTESIAN_POINT('Ctrl Pts',(21.4789407162088,92.0529280950311,8.10924243618854));
#22190=CARTESIAN_POINT('Ctrl Pts',(21.4963472798269,92.8820372167501,8.05658138110567));
#22191=CARTESIAN_POINT('Ctrl Pts',(21.9627432248614,93.7017199235893,8.00392032602278));
#22192=CARTESIAN_POINT('Ctrl Pts',(22.6666098382642,94.1402363229508,7.95125927093991));
#22193=CARTESIAN_POINT('Ctrl Pts',(23.3704764516669,94.5787527223123,7.89859821585703));
#22194=CARTESIAN_POINT('Ctrl Pts',(24.3118137334379,94.6361028141961,7.84593716077415));
#22195=CARTESIAN_POINT('Ctrl Pts',(25.0637092555993,94.2862772534286,7.79327610569127));
#22196=CARTESIAN_POINT('Ctrl Pts',(25.8156047777607,93.9364516926611,7.7406150506084));
#22197=CARTESIAN_POINT('Ctrl Pts',(26.3780585403126,93.1794504792422,7.68795399552551));
#22198=CARTESIAN_POINT('Ctrl Pts',(26.4959881169131,92.3585866313502,7.63529294044264));
#22199=CARTESIAN_POINT('Ctrl Pts',(26.6139176935135,91.5377227834583,7.58263188535976));
#22200=CARTESIAN_POINT('Ctrl Pts',(26.2873230841625,90.6529963010932,7.52997083027688));
#22201=CARTESIAN_POINT('Ctrl Pts',(25.6643205404874,90.1056457188879,7.477309775194));
#22202=CARTESIAN_POINT('Ctrl Pts',(25.0413179968122,89.5582951366826,7.42464872011113));
#22203=CARTESIAN_POINT('Ctrl Pts',(24.1219075188128,89.3483204546371,7.37198766502825));
#22204=CARTESIAN_POINT('Ctrl Pts',(23.3230574379199,89.5709487862187,7.31932660994537));
#22205=CARTESIAN_POINT('Ctrl Pts',(22.524207357027,89.7935771178002,7.26666555486249));
#22206=CARTESIAN_POINT('Ctrl Pts',(21.8459176732406,90.4488084630088,7.21400449977961));
#22207=CARTESIAN_POINT('Ctrl Pts',(21.595804339318,91.2394842188293,7.16134344469673));
#22208=CARTESIAN_POINT('Ctrl Pts',(21.5186090146758,91.4835194755669,7.14509006396181));
#22209=CARTESIAN_POINT('Ctrl Pts',(21.4822015557635,91.740457099368,7.1288366832269));
#22210=CARTESIAN_POINT('Ctrl Pts',(21.4842076940747,91.9979483279393,7.11258330249198));
#22211=CARTESIAN_POINT('Ctrl Pts',(21.4863706869161,92.0004946014336,7.38741669750803));
#22212=CARTESIAN_POINT('Ctrl Pts',(21.4871669427931,91.5514362957882,7.41570091701263));
#22213=CARTESIAN_POINT('Ctrl Pts',(21.6019741159521,91.1019979736551,7.44398513651724));
#22214=CARTESIAN_POINT('Ctrl Pts',(21.828352335515,90.7184032628621,7.47226935602185));
#22215=CARTESIAN_POINT('Ctrl Pts',(22.249835271893,90.0042063520624,7.52493041110472));
#22216=CARTESIAN_POINT('Ctrl Pts',(23.058078803959,89.5182560622716,7.57759146618761));
#22217=CARTESIAN_POINT('Ctrl Pts',(23.8865307175797,89.4809390082697,7.63025252127048));
#22218=CARTESIAN_POINT('Ctrl Pts',(24.7149826312004,89.4436219542678,7.68291357635336));
#22219=CARTESIAN_POINT('Ctrl Pts',(25.5636429263759,89.8549381360548,7.73557463143624));
#22220=CARTESIAN_POINT('Ctrl Pts',(26.0476296326406,90.5283489211969,7.78823568651912));
#22221=CARTESIAN_POINT('Ctrl Pts',(26.5316163389053,91.2017597063389,7.840896741602));
#22222=CARTESIAN_POINT('Ctrl Pts',(26.6509294562594,92.1372650948361,7.89355779668487));
#22223=CARTESIAN_POINT('Ctrl Pts',(26.3514585382347,92.910596864736,7.94621885176775));
#22224=CARTESIAN_POINT('Ctrl Pts',(26.05198762021,93.6839286346359,7.99887990685063));
#22225=CARTESIAN_POINT('Ctrl Pts',(25.3337326668066,94.2950867859385,8.05154096193351));
#22226=CARTESIAN_POINT('Ctrl Pts',(24.5224343764949,94.4669018166948,8.10420201701639));
#22227=CARTESIAN_POINT('Ctrl Pts',(23.7111360861833,94.6387168474512,8.15686307209927));
#22228=CARTESIAN_POINT('Ctrl Pts',(22.8067944589634,94.3711887576613,8.20952412718214));
#22229=CARTESIAN_POINT('Ctrl Pts',(22.2195442254209,93.7856437531992,8.26218518226502));
#22230=CARTESIAN_POINT('Ctrl Pts',(21.7540374326078,93.3214886766988,8.30392902067936));
#22231=CARTESIAN_POINT('Ctrl Pts',(21.4877768657504,92.6575058177296,8.34567285909369));
#22232=CARTESIAN_POINT('Ctrl Pts',(21.481789046694,91.9978055657336,8.38741669750803));
#22233=CARTESIAN_POINT('Origin',(24.,92.,5.));
#22234=CARTESIAN_POINT('',(21.4798237559162,92.0015869167785,9.38741669750802));
#22235=CARTESIAN_POINT('',(21.4850510509789,92.0017493960693,9.11258330249198));
#22236=CARTESIAN_POINT('',(21.4825,92.,5.));
#22237=CARTESIAN_POINT('',(25.9134659966651,93.6359872033749,10.));
#22238=CARTESIAN_POINT('Ctrl Pts',(21.4798237559162,92.0015869167785,9.38741669750802));
#22239=CARTESIAN_POINT('Ctrl Pts',(21.4853060534863,91.272907237615,9.43362796642338));
#22240=CARTESIAN_POINT('Ctrl Pts',(21.8192670107975,90.5399678433785,9.47983923533874));
#22241=CARTESIAN_POINT('Ctrl Pts',(22.3760117641787,90.0711228370539,9.5260505042541));
#22242=CARTESIAN_POINT('Ctrl Pts',(23.0104623389641,89.5368403279841,9.57871155933698));
#22243=CARTESIAN_POINT('Ctrl Pts',(23.9342252311204,89.3455170498785,9.63137261441985));
#22244=CARTESIAN_POINT('Ctrl Pts',(24.7281294273514,89.5853893188973,9.68403366950273));
#22245=CARTESIAN_POINT('Ctrl Pts',(25.5220336235825,89.8252615879161,9.73669472458561));
#22246=CARTESIAN_POINT('Ctrl Pts',(26.1860791238883,90.4963294040593,9.78935577966849));
#22247=CARTESIAN_POINT('Ctrl Pts',(26.4192657381557,91.2907292988926,9.84201683475137));
#22248=CARTESIAN_POINT('Ctrl Pts',(26.6524523524231,92.0851291937258,9.89467788983425));
#22249=CARTESIAN_POINT('Ctrl Pts',(26.4547800806522,93.0028611672492,9.94733894491712));
#22250=CARTESIAN_POINT('Ctrl Pts',(25.9134659966651,93.6359872033749,10.));
#22251=CARTESIAN_POINT('',(22.0828969142744,93.6385343069377,10.));
#22252=CARTESIAN_POINT('Origin',(24.,92.,10.));
#22253=CARTESIAN_POINT('Ctrl Pts',(22.082888458332,93.6385402287507,10.));
#22254=CARTESIAN_POINT('Ctrl Pts',(22.6060432359257,94.2476961579691,9.94901908464118));
#22255=CARTESIAN_POINT('Ctrl Pts',(23.4465813967719,94.5878273311312,9.89803816928235));
#22256=CARTESIAN_POINT('Ctrl Pts',(24.245735765903,94.5094848424925,9.84705725392352));
#22257=CARTESIAN_POINT('Ctrl Pts',(25.0712272651498,94.4285604793168,9.79439619884064));
#22258=CARTESIAN_POINT('Ctrl Pts',(25.8525623160909,93.9011252999797,9.74173514375777));
#22259=CARTESIAN_POINT('Ctrl Pts',(26.2358877550498,93.1658537096527,9.68907408867489));
#22260=CARTESIAN_POINT('Ctrl Pts',(26.6192131940086,92.4305821193258,9.63641303359201));
#22261=CARTESIAN_POINT('Ctrl Pts',(26.6045290209851,91.487474118009,9.58375197850913));
#22262=CARTESIAN_POINT('Ctrl Pts',(26.1982521612179,90.7645021442661,9.53109092342625));
#22263=CARTESIAN_POINT('Ctrl Pts',(25.7919753014507,90.0415301705232,9.47842986834338));
#22264=CARTESIAN_POINT('Ctrl Pts',(24.9941057549398,89.5386942243541,9.4257688132605));
#22265=CARTESIAN_POINT('Ctrl Pts',(24.1666097685101,89.4839132228271,9.37310775817762));
#22266=CARTESIAN_POINT('Ctrl Pts',(23.3391137820805,89.4291322213001,9.32044670309475));
#22267=CARTESIAN_POINT('Ctrl Pts',(22.4819913557322,89.8224061644151,9.26778564801186));
#22268=CARTESIAN_POINT('Ctrl Pts',(21.983903964328,90.4854401936108,9.21512459292898));
#22269=CARTESIAN_POINT('Ctrl Pts',(21.6606130378257,90.9157921545326,9.18094416278331));
#22270=CARTESIAN_POINT('Ctrl Pts',(21.4885781648623,91.4597899774222,9.14676373263764));
#22271=CARTESIAN_POINT('Ctrl Pts',(21.4850510509789,92.0017493960693,9.11258330249198));
#22272=CARTESIAN_POINT('Origin',(24.,92.,12.2084234471775));
#22273=CARTESIAN_POINT('',(20.9217235596202,92.0007881344673,1.79157655282254));
#22274=CARTESIAN_POINT('',(20.9313886636577,92.0003347861523,1.70842344717745));
#22275=CARTESIAN_POINT('',(20.9265,92.0000000000001,12.2084234471775));
#22276=CARTESIAN_POINT('',(24.7937992825328,89.0307770462543,0.999999999999999));
#22277=CARTESIAN_POINT('Ctrl Pts',(20.9313886636577,92.0003347861523,1.70842344717745));
#22278=CARTESIAN_POINT('Ctrl Pts',(20.9310462111061,92.494615243642,1.68292651844981));
#22279=CARTESIAN_POINT('Ctrl Pts',(21.2764428698256,94.0092287095088,1.6047685346393));
#22280=CARTESIAN_POINT('Ctrl Pts',(23.6460838412789,95.6088416124304,1.47394949574591));
#22281=CARTESIAN_POINT('Ctrl Pts',(26.8312245109703,94.2698537574842,1.31596633049727));
#22282=CARTESIAN_POINT('Ctrl Pts',(27.4433138069374,90.8667064664957,1.15798316524863));
#22283=CARTESIAN_POINT('Ctrl Pts',(25.7762533017603,89.2934286920663,1.05266105508288));
#22284=CARTESIAN_POINT('Ctrl Pts',(24.7937992825328,89.0307770462543,0.999999999999999));
#22285=CARTESIAN_POINT('',(23.2062007174671,89.0307770462543,0.999999999999999));
#22286=CARTESIAN_POINT('Origin',(24.,92.,0.999999999999999));
#22287=CARTESIAN_POINT('Ctrl Pts',(20.9217235596202,92.0007881344672,1.79157655282254));
#22288=CARTESIAN_POINT('Ctrl Pts',(20.921577466321,92.0437415214615,1.78934283757203));
#22289=CARTESIAN_POINT('Ctrl Pts',(20.9417780704225,93.09920230143,1.73444806723864));
#22290=CARTESIAN_POINT('Ctrl Pts',(22.1476051992024,95.1179528805984,1.62689224182237));
#22291=CARTESIAN_POINT('Ctrl Pts',(25.5990315417433,95.2555126520043,1.46890907657374));
#22292=CARTESIAN_POINT('Ctrl Pts',(27.5999506290771,92.4393708209745,1.3109259113251));
#22293=CARTESIAN_POINT('Ctrl Pts',(26.3493027558931,89.2605908411105,1.15462288580052));
#22294=CARTESIAN_POINT('Ctrl Pts',(24.1519058776304,88.7745943222177,1.05098091535882));
#22295=CARTESIAN_POINT('Ctrl Pts',(23.2042984301043,89.0256873776387,1.));
#22296=CARTESIAN_POINT('Origin',(24.,92.,12.2084234471775));
#22297=CARTESIAN_POINT('',(20.9300512599983,92.001902788448,2.79157655282254));
#22298=CARTESIAN_POINT('',(20.924991222385,91.997424467889,2.70842344717745));
#22299=CARTESIAN_POINT('',(20.9265,92.0000000000001,12.2084234471775));
#22300=CARTESIAN_POINT('Ctrl Pts',(20.924991222385,91.997424467889,2.70842344717745));
#22301=CARTESIAN_POINT('Ctrl Pts',(20.9323852777363,92.823989803404,2.66555951561375));
#22302=CARTESIAN_POINT('Ctrl Pts',(21.7006356086326,94.6781674340518,2.57003452896717));
#22303=CARTESIAN_POINT('Ctrl Pts',(24.8261379115922,95.5314383230663,2.42184848723771));
#22304=CARTESIAN_POINT('Ctrl Pts',(27.4089769044768,93.2380224116542,2.26386532198907));
#22305=CARTESIAN_POINT('Ctrl Pts',(26.8996889870333,89.8216055629486,2.10588215674044));
#22306=CARTESIAN_POINT('Ctrl Pts',(23.760424111462,88.3812146145649,1.94789899149181));
#22307=CARTESIAN_POINT('Ctrl Pts',(21.3097988736992,89.9256563753203,1.81541275497081));
#22308=CARTESIAN_POINT('Ctrl Pts',(20.9317535085566,91.473734231803,1.73558757353269));
#22309=CARTESIAN_POINT('Ctrl Pts',(20.9313886636577,92.0003347861523,1.70842344717745));
#22310=CARTESIAN_POINT('Ctrl Pts',(20.9300512599983,92.001902788448,2.79157655282254));
#22311=CARTESIAN_POINT('Ctrl Pts',(20.9278791968914,92.3814602359198,2.77197583473597));
#22312=CARTESIAN_POINT('Ctrl Pts',(21.1684423216004,93.77811538933,2.69971406156651));
#22313=CARTESIAN_POINT('Ctrl Pts',(23.2485917195109,95.548100055872,2.57479123331418));
#22314=CARTESIAN_POINT('Ctrl Pts',(26.5607983477153,94.5682620509693,2.41680806806554));
#22315=CARTESIAN_POINT('Ctrl Pts',(27.5502716608787,91.2589111130016,2.25882490281691));
#22316=CARTESIAN_POINT('Ctrl Pts',(25.3195310914441,88.6217767625239,2.10084173756827));
#22317=CARTESIAN_POINT('Ctrl Pts',(21.9403860022537,89.042720793944,1.94509228757015));
#22318=CARTESIAN_POINT('Ctrl Pts',(20.9250216955149,91.0310920004536,1.84200389265491));
#22319=CARTESIAN_POINT('Ctrl Pts',(20.9217235596202,92.0007881344672,1.79157655282254));
#22320=CARTESIAN_POINT('Origin',(24.,92.,12.2084234471775));
#22321=CARTESIAN_POINT('',(20.9283005269272,91.9974284308675,3.79157655282254));
#22322=CARTESIAN_POINT('',(20.9237789745046,92.0022328818336,3.70842344717745));
#22323=CARTESIAN_POINT('',(20.9265,92.0000000000001,12.2084234471775));
#22324=CARTESIAN_POINT('Ctrl Pts',(20.9237789745046,92.0022328818336,3.70842344717745));
#22325=CARTESIAN_POINT('Ctrl Pts',(20.9225841955761,92.1480569773283,3.70085356786056));
#22326=CARTESIAN_POINT('Ctrl Pts',(20.9980295686384,93.3070877047366,3.6406226334608));
#22327=CARTESIAN_POINT('Ctrl Pts',(22.47008521615,95.288313514808,3.52773064397815));
#22328=CARTESIAN_POINT('Ctrl Pts',(25.9177921721966,95.0782652002028,3.36974747872952));
#22329=CARTESIAN_POINT('Ctrl Pts',(27.625996631401,92.0761257688787,3.21176431348088));
#22330=CARTESIAN_POINT('Ctrl Pts',(26.0452974398026,89.0049366707406,3.05378114823225));
#22331=CARTESIAN_POINT('Ctrl Pts',(22.6094455863014,88.6503742748602,2.89579798298361));
#22332=CARTESIAN_POINT('Ctrl Pts',(21.0248750936135,90.6059034459642,2.78067874929868));
#22333=CARTESIAN_POINT('Ctrl Pts',(20.923301212371,91.808501931078,2.71822057069663));
#22334=CARTESIAN_POINT('Ctrl Pts',(20.924991222385,91.997424467889,2.70842344717745));
#22335=CARTESIAN_POINT('Ctrl Pts',(20.9283005269272,91.9974284308675,3.79157655282254));
#22336=CARTESIAN_POINT('Ctrl Pts',(20.9340588461039,92.7122593506074,3.7546088318999));
#22337=CARTESIAN_POINT('Ctrl Pts',(21.5376068210963,94.4541464677684,3.66498005589438));
#22338=CARTESIAN_POINT('Ctrl Pts',(24.4293689246723,95.601288842286,3.52269022480598));
#22339=CARTESIAN_POINT('Ctrl Pts',(27.2506150476498,93.6084592491481,3.36470705955735));
#22340=CARTESIAN_POINT('Ctrl Pts',(27.1234423470096,90.1567020569745,3.20672389430872));
#22341=CARTESIAN_POINT('Ctrl Pts',(24.1632008787755,88.3768793413442,3.04874072906008));
#22342=CARTESIAN_POINT('Ctrl Pts',(21.4405686580064,89.6964446537074,2.91035828189802));
#22343=CARTESIAN_POINT('Ctrl Pts',(20.9337148573203,91.361707002383,2.82463688981884));
#22344=CARTESIAN_POINT('Ctrl Pts',(20.9300512599983,92.001902788448,2.79157655282254));
#22345=CARTESIAN_POINT('Origin',(24.,92.,12.2084234471775));
#22346=CARTESIAN_POINT('',(20.921616510855,92.0005832747793,4.79157655282255));
#22347=CARTESIAN_POINT('',(20.931280553226,92.0004324467725,4.70842344717745));
#22348=CARTESIAN_POINT('',(20.9265,92.0000000000001,12.2084234471775));
#22349=CARTESIAN_POINT('Ctrl Pts',(20.931280553226,92.0004324467725,4.70842344717745));
#22350=CARTESIAN_POINT('Ctrl Pts',(20.9306673998754,92.4838071032452,4.6834865650245));
#22351=CARTESIAN_POINT('Ctrl Pts',(21.2653045337522,93.9871569627812,4.60588862778867));
#22352=CARTESIAN_POINT('Ctrl Pts',(23.608671679144,95.6056215728149,4.47562963546996));
#22353=CARTESIAN_POINT('Ctrl Pts',(26.8057465121274,94.2981364769134,4.31764647022132));
#22354=CARTESIAN_POINT('Ctrl Pts',(27.4579134988245,90.9061631628407,4.15966330497269));
#22355=CARTESIAN_POINT('Ctrl Pts',(24.973634903104,88.5063371813541,4.00168013972405));
#22356=CARTESIAN_POINT('Ctrl Pts',(21.7675876228179,89.2385332724819,3.85126685379231));
#22357=CARTESIAN_POINT('Ctrl Pts',(20.9308958629532,91.1336087406012,3.75351462294344));
#22358=CARTESIAN_POINT('Ctrl Pts',(20.9237789745046,92.0022328818336,3.70842344717745));
#22359=CARTESIAN_POINT('Ctrl Pts',(20.921616510855,92.0005832747793,4.79157655282255));
#22360=CARTESIAN_POINT('Ctrl Pts',(20.921531931191,92.0327646210543,4.78990288414672));
#22361=CARTESIAN_POINT('Ctrl Pts',(20.9365121376523,93.0774335164315,4.73556816038801));
#22362=CARTESIAN_POINT('Ctrl Pts',(22.1148104659795,95.0983381963849,4.62857238154642));
#22363=CARTESIAN_POINT('Ctrl Pts',(25.5645421252575,95.2719790790493,4.47058921629779));
#22364=CARTESIAN_POINT('Ctrl Pts',(27.5951806759185,92.4778232584365,4.31260605104916));
#22365=CARTESIAN_POINT('Ctrl Pts',(26.3648676419543,89.2502654310841,4.15462288580052));
#22366=CARTESIAN_POINT('Ctrl Pts',(22.9895389394378,88.5168107165773,3.99663972055189));
#22367=CARTESIAN_POINT('Ctrl Pts',(21.1060882305935,90.3750682368836,3.87562427622589));
#22368=CARTESIAN_POINT('Ctrl Pts',(20.9258560368481,91.693972328853,3.80726988698278));
#22369=CARTESIAN_POINT('Ctrl Pts',(20.9283005269272,91.9974284308675,3.79157655282254));
#22370=CARTESIAN_POINT('Origin',(24.,92.,12.2084234471775));
#22371=CARTESIAN_POINT('',(20.9298378032017,92.0020253448728,5.79157655282255));
#22372=CARTESIAN_POINT('',(20.9253101281647,91.9973677263042,5.70842344717746));
#22373=CARTESIAN_POINT('',(20.9265,92.0000000000001,12.2084234471775));
#22374=CARTESIAN_POINT('Ctrl Pts',(20.9253101281647,91.9973677263042,5.70842344717746));
#22375=CARTESIAN_POINT('Ctrl Pts',(20.9326785820548,92.8133509452838,5.66611956218844));
#22376=CARTESIAN_POINT('Ctrl Pts',(21.6842659096931,94.6570905748761,5.57115462211654));
#22377=CARTESIAN_POINT('Ctrl Pts',(24.7888216332756,95.5399724866421,5.42352862696176));
#22378=CARTESIAN_POINT('Ctrl Pts',(27.3956991685213,93.2739199079453,5.26554546171313));
#22379=CARTESIAN_POINT('Ctrl Pts',(26.9225616555133,89.8523784912207,5.1075622964645));
#22380=CARTESIAN_POINT('Ctrl Pts',(23.798560967482,88.3788030856943,4.94957913121586));
#22381=CARTESIAN_POINT('Ctrl Pts',(21.3215406064417,89.9039233849086,4.81653284812018));
#22382=CARTESIAN_POINT('Ctrl Pts',(20.9319622410737,91.4630291545808,4.73614762010738));
#22383=CARTESIAN_POINT('Ctrl Pts',(20.931280553226,92.0004324467725,4.70842344717745));
#22384=CARTESIAN_POINT('Ctrl Pts',(20.9298378032017,92.0020253448728,5.79157655282255));
#22385=CARTESIAN_POINT('Ctrl Pts',(20.9275816449178,92.3706733068195,5.77253588131066));
#22386=CARTESIAN_POINT('Ctrl Pts',(21.15907081827,93.7561579838992,5.70083415471589));
#22387=CARTESIAN_POINT('Ctrl Pts',(23.2111785351691,95.5399717307178,5.57647137303823));
#22388=CARTESIAN_POINT('Ctrl Pts',(26.5335435065542,94.5951486388852,5.4184882077896));
#22389=CARTESIAN_POINT('Ctrl Pts',(27.5578980422048,91.2964371536349,5.26050504254097));
#22390=CARTESIAN_POINT('Ctrl Pts',(25.3551176148943,88.6358811841043,5.10252187729233));
#22391=CARTESIAN_POINT('Ctrl Pts',(21.9595568927721,89.0225555274607,4.94621238071952));
#22392=CARTESIAN_POINT('Ctrl Pts',(20.9241931833304,91.0201964387709,4.8425639392296));
#22393=CARTESIAN_POINT('Ctrl Pts',(20.921616510855,92.0005832747793,4.79157655282255));
#22394=CARTESIAN_POINT('Origin',(24.,92.,12.2084234471775));
#22395=CARTESIAN_POINT('',(20.9285848451792,91.9974952079133,6.79157655282254));
#22396=CARTESIAN_POINT('',(20.9234955495304,92.0021186992919,6.70842344717746));
#22397=CARTESIAN_POINT('',(20.9265,92.0000000000001,12.2084234471775));
#22398=CARTESIAN_POINT('Ctrl Pts',(20.9234955495304,92.0021186992918,6.70842344717746));
#22399=CARTESIAN_POINT('Ctrl Pts',(20.9224296149028,92.1371217233644,6.70141361443525));
#22400=CARTESIAN_POINT('Ctrl Pts',(20.9915972274954,93.2852299955925,6.64174272661017));
#22401=CARTESIAN_POINT('Ctrl Pts',(22.4354575406508,95.2719797777492,6.5294107837022));
#22402=CARTESIAN_POINT('Ctrl Pts',(25.8851899365834,95.0983388580017,6.37142761845357));
#22403=CARTESIAN_POINT('Ctrl Pts',(27.624990714543,92.1143988405745,6.21344445320494));
#22404=CARTESIAN_POINT('Ctrl Pts',(26.0768011856691,89.0266951703267,6.0554612879563));
#22405=CARTESIAN_POINT('Ctrl Pts',(22.6448820957342,88.6358804657318,5.89747812270767));
#22406=CARTESIAN_POINT('Ctrl Pts',(21.031950056972,90.5840074378853,5.78179884244805));
#22407=CARTESIAN_POINT('Ctrl Pts',(20.9235061252868,91.7975922920882,5.71878061727132));
#22408=CARTESIAN_POINT('Ctrl Pts',(20.9253101281647,91.9973677263042,5.70842344717746));
#22409=CARTESIAN_POINT('Ctrl Pts',(20.9285848451792,91.9974952079133,6.79157655282254));
#22410=CARTESIAN_POINT('Ctrl Pts',(20.934071073012,92.7016617835356,6.75516887847459));
#22411=CARTESIAN_POINT('Ctrl Pts',(21.5231705466971,94.4326506257242,6.66610014904376));
#22412=CARTESIAN_POINT('Ctrl Pts',(24.3913282372869,95.6056208028792,6.52437036453004));
#22413=CARTESIAN_POINT('Ctrl Pts',(27.2334543225922,93.6426844805108,6.36638719928141));
#22414=CARTESIAN_POINT('Ctrl Pts',(27.1427269710462,90.1897772675991,6.20840403403277));
#22415=CARTESIAN_POINT('Ctrl Pts',(24.2014389895034,88.3788038589624,6.05042086878413));
#22416=CARTESIAN_POINT('Ctrl Pts',(21.453954137816,89.6747786389992,5.9114783750474));
#22417=CARTESIAN_POINT('Ctrl Pts',(20.9338215338625,91.3510984132479,5.82519693639353));
#22418=CARTESIAN_POINT('Ctrl Pts',(20.9298378032017,92.0020253448728,5.79157655282255));
#22419=CARTESIAN_POINT('Origin',(24.,92.,12.2084234471775));
#22420=CARTESIAN_POINT('',(20.9215395889802,92.0003901744224,7.79157655282255));
#22421=CARTESIAN_POINT('',(20.9312255436888,92.0006038361494,7.70842344717746));
#22422=CARTESIAN_POINT('',(20.9265,92.0000000000001,12.2084234471775));
#22423=CARTESIAN_POINT('Ctrl Pts',(20.9312255436888,92.0006038361494,7.70842344717745));
#22424=CARTESIAN_POINT('Ctrl Pts',(20.9303877260141,92.473101429326,7.68404661159919));
#22425=CARTESIAN_POINT('Ctrl Pts',(21.2544808710823,93.9652421749014,7.60700872093804));
#22426=CARTESIAN_POINT('Ctrl Pts',(23.5706309836456,95.601289611435,7.47730977519401));
#22427=CARTESIAN_POINT('Ctrl Pts',(26.7813300499739,94.327627111039,7.31932660994538));
#22428=CARTESIAN_POINT('Ctrl Pts',(27.4692678342079,90.9427273359204,7.16134344469674));
#22429=CARTESIAN_POINT('Ctrl Pts',(25.0104612763354,88.5168099727604,7.00336027944811));
#22430=CARTESIAN_POINT('Ctrl Pts',(21.7848977769712,89.2177208955611,6.85238694694168));
#22431=CARTESIAN_POINT('Ctrl Pts',(20.9304374011369,91.1229175406829,6.75407466951813));
#22432=CARTESIAN_POINT('Ctrl Pts',(20.9234955495304,92.0021186992918,6.70842344717746));
#22433=CARTESIAN_POINT('Ctrl Pts',(20.9215395889802,92.0003901744224,7.79157655282255));
#22434=CARTESIAN_POINT('Ctrl Pts',(20.9215009805821,92.0218014948814,7.7904629307214));
#22435=CARTESIAN_POINT('Ctrl Pts',(20.931364389904,93.0556766305594,7.73668825353738));
#22436=CARTESIAN_POINT('Ctrl Pts',(22.0822082378054,95.0782645420543,7.63025252127048));
#22437=CARTESIAN_POINT('Ctrl Pts',(25.5299144568995,95.2883128130433,7.47226935602185));
#22438=CARTESIAN_POINT('Ctrl Pts',(27.5899362712429,92.5157488852068,7.31428619077321));
#22439=CARTESIAN_POINT('Ctrl Pts',(26.3937632442238,89.2753832325168,7.15630302552458));
#22440=CARTESIAN_POINT('Ctrl Pts',(23.0263653048422,88.5063379273328,6.99831986027595));
#22441=CARTESIAN_POINT('Ctrl Pts',(21.1145962575175,90.3531167219238,6.87674436937527));
#22442=CARTESIAN_POINT('Ctrl Pts',(20.9261356431535,91.6831360059216,6.80782993355747));
#22443=CARTESIAN_POINT('Ctrl Pts',(20.9285848451792,91.9974952079133,6.79157655282254));
#22444=CARTESIAN_POINT('Origin',(24.,92.,12.2084234471775));
#22445=CARTESIAN_POINT('',(20.9296144608475,92.002135757227,8.79157655282255));
#22446=CARTESIAN_POINT('',(20.925632029797,91.9973209161002,8.70842344717745));
#22447=CARTESIAN_POINT('',(20.9265,92.0000000000001,12.2084234471775));
#22448=CARTESIAN_POINT('Ctrl Pts',(20.925632029797,91.9973209161002,8.70842344717745));
#22449=CARTESIAN_POINT('Ctrl Pts',(20.9329422827742,92.802718621963,8.66667960876312));
#22450=CARTESIAN_POINT('Ctrl Pts',(21.6680867896664,94.6359730058285,8.57227471526591));
#22451=CARTESIAN_POINT('Ctrl Pts',(24.7514084417654,95.5481008201034,8.42520876668582));
#22452=CARTESIAN_POINT('Ctrl Pts',(27.382061787488,93.3096961590962,8.26722560143718));
#22453=CARTESIAN_POINT('Ctrl Pts',(26.9450700899455,89.8833496110771,8.10924243618856));
#22454=CARTESIAN_POINT('Ctrl Pts',(23.8367990863051,88.3768785667208,7.95125927093992));
#22455=CARTESIAN_POINT('Ctrl Pts',(21.3333229638364,89.8820745861535,7.81765294126955));
#22456=CARTESIAN_POINT('Ctrl Pts',(20.9321976558787,91.4523691976585,7.73670766668206));
#22457=CARTESIAN_POINT('Ctrl Pts',(20.9312255436888,92.0006038361494,7.70842344717745));
#22458=CARTESIAN_POINT('Ctrl Pts',(20.9296144608475,92.0021357572271,8.79157655282255));
#22459=CARTESIAN_POINT('Ctrl Pts',(20.927286249777,92.3598775143589,8.77309592788534));
#22460=CARTESIAN_POINT('Ctrl Pts',(21.1498335279144,93.734213837484,8.70195424786525));
#22461=CARTESIAN_POINT('Ctrl Pts',(23.1738622820844,95.5314375280541,8.57815151276229));
#22462=CARTESIAN_POINT('Ctrl Pts',(26.5060022838615,94.621754023121,8.42016834751365));
#22463=CARTESIAN_POINT('Ctrl Pts',(27.5651291305171,91.3340327163824,8.26218518226502));
#22464=CARTESIAN_POINT('Ctrl Pts',(25.3905541137142,88.6503749960184,8.10420201701638));
#22465=CARTESIAN_POINT('Ctrl Pts',(21.9789222863521,89.0024380002803,7.9473324738689));
#22466=CARTESIAN_POINT('Ctrl Pts',(20.9233266977404,91.0093011817766,7.84312398580428));
#22467=CARTESIAN_POINT('Ctrl Pts',(20.9215395889802,92.0003901744224,7.79157655282255));
#22468=CARTESIAN_POINT('Origin',(24.,92.,12.2084234471775));
#22469=CARTESIAN_POINT('',(20.929711085108,91.9968960951898,9.79157655282254));
#22470=CARTESIAN_POINT('',(20.9232326966468,92.0019373937314,9.70842344717745));
#22471=CARTESIAN_POINT('',(20.9265,92.0000000000001,12.2084234471775));
#22472=CARTESIAN_POINT('',(23.2062007174671,89.0307770462543,10.));
#22473=CARTESIAN_POINT('Ctrl Pts',(23.2062007174671,89.0307770462543,10.));
#22474=CARTESIAN_POINT('Ctrl Pts',(22.2237466982397,89.2934286920664,9.94733894491712));
#22475=CARTESIAN_POINT('Ctrl Pts',(21.1240892170206,90.3312175686103,9.87786446252463));
#22476=CARTESIAN_POINT('Ctrl Pts',(20.9273642764696,91.6716348903192,9.80838998013215));
#22477=CARTESIAN_POINT('Ctrl Pts',(20.929711085108,91.9968960951898,9.79157655282254));
#22478=CARTESIAN_POINT('',(24.7956975117795,89.0256988737941,10.));
#22479=CARTESIAN_POINT('Origin',(24.,92.,10.));
#22480=CARTESIAN_POINT('Ctrl Pts',(24.7957019287906,89.0256870573369,10.));
#22481=CARTESIAN_POINT('Ctrl Pts',(23.8480950072444,88.7745945181247,9.94901908464118));
#22482=CARTESIAN_POINT('Ctrl Pts',(21.7874430689301,89.2303448029462,9.851826900367));
#22483=CARTESIAN_POINT('Ctrl Pts',(20.9299257816843,91.1123258767864,9.75463471609281));
#22484=CARTESIAN_POINT('Ctrl Pts',(20.9232326966468,92.0019373937314,9.70842344717745));
#22485=CARTESIAN_POINT('Origin',(24.,-92.,5.));
#22486=CARTESIAN_POINT('',(21.486504426694,-91.9997257424662,1.38741669750802));
#22487=CARTESIAN_POINT('',(21.4843725317804,-92.0035302714346,1.11258330249198));
#22488=CARTESIAN_POINT('',(21.4825,-92.,5.));
#22489=CARTESIAN_POINT('',(22.086534003335,-90.364012796625,0.999999999999999));
#22490=CARTESIAN_POINT('Ctrl Pts',(21.4843725317804,-92.0035302714346,1.11258330249198));
#22491=CARTESIAN_POINT('Ctrl Pts',(21.4895356694446,-91.4109125587033,1.07505553499465));
#22492=CARTESIAN_POINT('Ctrl Pts',(21.700778171916,-90.8151964396955,1.03752776749732));
#22493=CARTESIAN_POINT('Ctrl Pts',(22.086534003335,-90.364012796625,0.999999999999996));
#22494=CARTESIAN_POINT('',(21.4825,-92.,1.));
#22495=CARTESIAN_POINT('Origin',(24.,-92.,1.));
#22496=CARTESIAN_POINT('',(21.4825,-92.,0.));
#22497=CARTESIAN_POINT('',(21.4825,-92.,5.));
#22498=CARTESIAN_POINT('Origin',(24.,-92.,0.));
#22499=CARTESIAN_POINT('',(25.9171033775212,-90.3614656597817,0.999999999999999));
#22500=CARTESIAN_POINT('Origin',(24.,-92.,1.));
#22501=CARTESIAN_POINT('Ctrl Pts',(25.9171118396844,-90.3614597340102,0.999999999999999));
#22502=CARTESIAN_POINT('Ctrl Pts',(25.3939571501801,-89.7523042564146,1.05098091535882));
#22503=CARTESIAN_POINT('Ctrl Pts',(24.5534187715749,-89.4121721444715,1.10196183071765));
#22504=CARTESIAN_POINT('Ctrl Pts',(23.7542642221519,-89.4905144511518,1.15294274607647));
#22505=CARTESIAN_POINT('Ctrl Pts',(22.9287725366714,-89.5714386263726,1.20560380115935));
#22506=CARTESIAN_POINT('Ctrl Pts',(22.147437339474,-90.0988744252836,1.25826485624223));
#22507=CARTESIAN_POINT('Ctrl Pts',(21.7641118492188,-90.8341462554665,1.31092591132511));
#22508=CARTESIAN_POINT('Ctrl Pts',(21.578516959615,-91.1901431761531,1.33642284005274));
#22509=CARTESIAN_POINT('Ctrl Pts',(21.4862239279038,-91.5948612398581,1.36191976878038));
#22510=CARTESIAN_POINT('Ctrl Pts',(21.486504426694,-91.9997257424662,1.38741669750802));
#22511=CARTESIAN_POINT('Origin',(24.,-92.,5.));
#22512=CARTESIAN_POINT('',(21.4812642899864,-92.0021096151708,2.38741669750802));
#22513=CARTESIAN_POINT('',(21.4785878033439,-91.999354427872,2.11258330249198));
#22514=CARTESIAN_POINT('',(21.4825,-92.,5.));
#22515=CARTESIAN_POINT('Ctrl Pts',(21.4785878033439,-91.999354427872,2.11258330249198));
#22516=CARTESIAN_POINT('Ctrl Pts',(21.4784681386269,-91.9641713652006,2.11034958724146));
#22517=CARTESIAN_POINT('Ctrl Pts',(21.4791414214071,-91.928993039682,2.10811587199095));
#22518=CARTESIAN_POINT('Ctrl Pts',(21.480621972346,-91.8938487862731,2.10588215674044));
#22519=CARTESIAN_POINT('Ctrl Pts',(21.5155267680805,-91.0653038478858,2.05322110165756));
#22520=CARTESIAN_POINT('Ctrl Pts',(21.9991163215578,-90.2556964040098,2.00056004657468));
#22521=CARTESIAN_POINT('Ctrl Pts',(22.712087549401,-89.8321134766477,1.9478989914918));
#22522=CARTESIAN_POINT('Ctrl Pts',(23.4250587772441,-89.4085305492857,1.89523793640892));
#22523=CARTESIAN_POINT('Ctrl Pts',(24.3674116794533,-89.3709721384377,1.84257688132605));
#22524=CARTESIAN_POINT('Ctrl Pts',(25.1117465266451,-89.7366426720986,1.78991582624317));
#22525=CARTESIAN_POINT('Ctrl Pts',(25.8560813738369,-90.1023132057595,1.73725477116029));
#22526=CARTESIAN_POINT('Ctrl Pts',(26.4023981660114,-90.8712126839294,1.68459371607741));
#22527=CARTESIAN_POINT('Ctrl Pts',(26.502987230808,-91.6942827713944,1.63193266099453));
#22528=CARTESIAN_POINT('Ctrl Pts',(26.6035762956046,-92.5173528588593,1.57927160591166));
#22529=CARTESIAN_POINT('Ctrl Pts',(26.2584376330233,-93.3945935556194,1.52661055082878));
#22530=CARTESIAN_POINT('Ctrl Pts',(25.6239875152205,-93.9288761516103,1.4739494957459));
#22531=CARTESIAN_POINT('Ctrl Pts',(24.9895373974178,-94.4631587476011,1.42128844066302));
#22532=CARTESIAN_POINT('Ctrl Pts',(24.0657758243935,-94.6544832428229,1.36862738558014));
#22533=CARTESIAN_POINT('Ctrl Pts',(23.2718709044643,-94.4146102691233,1.31596633049727));
#22534=CARTESIAN_POINT('Ctrl Pts',(22.4779659845352,-94.1747372954238,1.26330527541439));
#22535=CARTESIAN_POINT('Ctrl Pts',(21.8139177177011,-93.503666852803,1.21064422033151));
#22536=CARTESIAN_POINT('Ctrl Pts',(21.5807312014042,-92.7092672371347,1.15798316524863));
#22537=CARTESIAN_POINT('Ctrl Pts',(21.5137200371456,-92.480979409957,1.14284987766308));
#22538=CARTESIAN_POINT('Ctrl Pts',(21.4822904668902,-92.2425067646591,1.12771659007753));
#22539=CARTESIAN_POINT('Ctrl Pts',(21.4843725317804,-92.0035302714346,1.11258330249198));
#22540=CARTESIAN_POINT('Ctrl Pts',(21.486504426694,-91.9997257424662,1.38741669750802));
#22541=CARTESIAN_POINT('Ctrl Pts',(21.4868032667881,-92.4310635958632,1.41458082386326));
#22542=CARTESIAN_POINT('Ctrl Pts',(21.5921778743622,-92.8625676650245,1.4417449502185));
#22543=CARTESIAN_POINT('Ctrl Pts',(21.8017475042685,-93.2354979719165,1.46890907657374));
#22544=CARTESIAN_POINT('Ctrl Pts',(22.2080244328865,-93.958469996729,1.52157013165662));
#22545=CARTESIAN_POINT('Ctrl Pts',(23.0058940734354,-94.4613061848995,1.57423118673949));
#22546=CARTESIAN_POINT('Ctrl Pts',(23.8333901892196,-94.5160872321709,1.62689224182237));
#22547=CARTESIAN_POINT('Ctrl Pts',(24.6608863050039,-94.5708682794422,1.67955329690525));
#22548=CARTESIAN_POINT('Ctrl Pts',(25.5180088960235,-94.1775941858145,1.73221435198813));
#22549=CARTESIAN_POINT('Ctrl Pts',(26.0160963730402,-93.5145600286215,1.78487540707101));
#22550=CARTESIAN_POINT('Ctrl Pts',(26.5141838500568,-92.8515258714286,1.83753646215389));
#22551=CARTESIAN_POINT('Ctrl Pts',(26.6532362130706,-91.9187316506704,1.89019751723677));
#22552=CARTESIAN_POINT('Ctrl Pts',(26.3701623803631,-91.1392455433219,1.94285857231964));
#22553=CARTESIAN_POINT('Ctrl Pts',(26.0870885476557,-90.3597594359734,1.99551962740252));
#22554=CARTESIAN_POINT('Ctrl Pts',(25.3818885192271,-89.7335814420344,2.0481806824854));
#22555=CARTESIAN_POINT('Ctrl Pts',(24.5743964779126,-89.5446792416752,2.10084173756828));
#22556=CARTESIAN_POINT('Ctrl Pts',(23.7669044365982,-89.3557770413159,2.15350279265115));
#22557=CARTESIAN_POINT('Ctrl Pts',(22.857120382398,-89.6041506345363,2.20616384773403));
#22558=CARTESIAN_POINT('Ctrl Pts',(22.2576400878061,-90.1771655681069,2.25882490281691));
#22559=CARTESIAN_POINT('Ctrl Pts',(21.7696877997114,-90.6435761415163,2.30168883438061));
#22560=CARTESIAN_POINT('Ctrl Pts',(21.4873207515092,-91.3250710178653,2.34455276594432));
#22561=CARTESIAN_POINT('Ctrl Pts',(21.4812642899864,-92.0021096151708,2.38741669750802));
#22562=CARTESIAN_POINT('Origin',(24.,-92.,5.));
#22563=CARTESIAN_POINT('',(21.4802713394158,-91.9981710493934,3.38741669750802));
#22564=CARTESIAN_POINT('',(21.4854090148867,-91.9984414282173,3.11258330249198));
#22565=CARTESIAN_POINT('',(21.4825,-92.,5.));
#22566=CARTESIAN_POINT('Ctrl Pts',(21.4854090148867,-91.9984414282173,3.11258330249198));
#22567=CARTESIAN_POINT('Ctrl Pts',(21.4836298808409,-91.6875464209233,3.0929825844054));
#22568=CARTESIAN_POINT('Ctrl Pts',(21.5370775357559,-91.3772414115068,3.07338186631883));
#22569=CARTESIAN_POINT('Ctrl Pts',(21.6485421342809,-91.0894033947304,3.05378114823225));
#22570=CARTESIAN_POINT('Ctrl Pts',(21.9480129667671,-90.3160718469037,3.00112009314937));
#22571=CARTESIAN_POINT('Ctrl Pts',(22.666267715158,-89.704913874088,2.94845903806649));
#22572=CARTESIAN_POINT('Ctrl Pts',(23.4775657731397,-89.5330988908351,2.89579798298361));
#22573=CARTESIAN_POINT('Ctrl Pts',(24.2888638311213,-89.3612839075822,2.84313692790073));
#22574=CARTESIAN_POINT('Ctrl Pts',(25.1932051986936,-89.6288119138921,2.79047587281785));
#22575=CARTESIAN_POINT('Ctrl Pts',(25.780455264855,-90.2143567539364,2.73781481773498));
#22576=CARTESIAN_POINT('Ctrl Pts',(26.3677053310164,-90.7999015939806,2.6851537626521));
#22577=CARTESIAN_POINT('Ctrl Pts',(26.6378640957668,-91.7034632677594,2.63249270756922));
#22578=CARTESIAN_POINT('Ctrl Pts',(26.4684106985951,-92.5152563159492,2.57983165248634));
#22579=CARTESIAN_POINT('Ctrl Pts',(26.2989573014234,-93.3270493641389,2.52717059740346));
#22580=CARTESIAN_POINT('Ctrl Pts',(25.6898917423295,-94.0470737867398,2.47450954232059));
#22581=CARTESIAN_POINT('Ctrl Pts',(24.9174341156813,-94.3487960615597,2.42184848723771));
#22582=CARTESIAN_POINT('Ctrl Pts',(24.1449764890331,-94.6505183363795,2.36918743215483));
#22583=CARTESIAN_POINT('Ctrl Pts',(23.2091267948305,-94.5339384634185,2.31652637707195));
#22584=CARTESIAN_POINT('Ctrl Pts',(22.5343119667251,-94.0519073104887,2.26386532198907));
#22585=CARTESIAN_POINT('Ctrl Pts',(21.8881206474051,-93.5903223931276,2.21343798215671));
#22586=CARTESIAN_POINT('Ctrl Pts',(21.4812892995851,-92.7936312531158,2.16301064232434));
#22587=CARTESIAN_POINT('Ctrl Pts',(21.4785878033439,-91.999354427872,2.11258330249198));
#22588=CARTESIAN_POINT('Ctrl Pts',(21.4812642899864,-92.0021096151708,2.38741669750802));
#22589=CARTESIAN_POINT('Ctrl Pts',(21.4798800048902,-92.1568558207351,2.39721382102719));
#22590=CARTESIAN_POINT('Ctrl Pts',(21.4929305169812,-92.3113692249255,2.40701094454637));
#22591=CARTESIAN_POINT('Ctrl Pts',(21.5212603168746,-92.4630284201484,2.41680806806555));
#22592=CARTESIAN_POINT('Ctrl Pts',(21.6735373755183,-93.2782200646987,2.46946912314842));
#22593=CARTESIAN_POINT('Ctrl Pts',(22.2672680277891,-94.0109470798785,2.5221301782313));
#22594=CARTESIAN_POINT('Ctrl Pts',(23.0331836548293,-94.3289069878288,2.57479123331418));
#22595=CARTESIAN_POINT('Ctrl Pts',(23.7990992818695,-94.6468668957792,2.62745228839706));
#22596=CARTESIAN_POINT('Ctrl Pts',(24.7371998836791,-94.5500596964999,2.68011334347994));
#22597=CARTESIAN_POINT('Ctrl Pts',(25.4220416283354,-94.0823882608119,2.73277439856281));
#22598=CARTESIAN_POINT('Ctrl Pts',(26.1068833729918,-93.6147168251238,2.78543545364569));
#22599=CARTESIAN_POINT('Ctrl Pts',(26.538466260495,-92.776181153027,2.83809650872857));
#22600=CARTESIAN_POINT('Ctrl Pts',(26.5210596939212,-91.9470718966112,2.89075756381145));
#22601=CARTESIAN_POINT('Ctrl Pts',(26.5036531273474,-91.1179626401953,2.94341861889433));
#22602=CARTESIAN_POINT('Ctrl Pts',(26.0372571066966,-90.2982797994603,2.9960796739772));
#22603=CARTESIAN_POINT('Ctrl Pts',(25.3333903788126,-89.8597633286133,3.04874072906008));
#22604=CARTESIAN_POINT('Ctrl Pts',(24.6295236509285,-89.4212468577661,3.10140178414296));
#22605=CARTESIAN_POINT('Ctrl Pts',(23.6881862158112,-89.3638967568069,3.15406283922584));
#22606=CARTESIAN_POINT('Ctrl Pts',(22.9362905712497,-89.7137223745679,3.20672389430872));
#22607=CARTESIAN_POINT('Ctrl Pts',(22.1843949266883,-90.063547992329,3.2593849493916));
#22608=CARTESIAN_POINT('Ctrl Pts',(21.6219410726826,-90.8205493288104,3.31204600447447));
#22609=CARTESIAN_POINT('Ctrl Pts',(21.5040114769092,-91.6414133102583,3.36470705955735));
#22610=CARTESIAN_POINT('Ctrl Pts',(21.4870594274965,-91.759410210726,3.37227693887424));
#22611=CARTESIAN_POINT('Ctrl Pts',(21.4792926975419,-91.8787267215066,3.37984681819113));
#22612=CARTESIAN_POINT('Ctrl Pts',(21.4802713394158,-91.9981710493934,3.38741669750802));
#22613=CARTESIAN_POINT('Origin',(24.,-92.,5.));
#22614=CARTESIAN_POINT('',(21.4864158728456,-91.9996457834086,4.38741669750802));
#22615=CARTESIAN_POINT('',(21.4839749917546,-92.0021063689016,4.11258330249198));
#22616=CARTESIAN_POINT('',(21.4825,-92.,5.));
#22617=CARTESIAN_POINT('Ctrl Pts',(21.4839749917546,-92.0021063689016,4.11258330249198));
#22618=CARTESIAN_POINT('Ctrl Pts',(21.4886916234371,-91.4165893004159,4.07561558156934));
#22619=CARTESIAN_POINT('Ctrl Pts',(21.6925944465197,-90.8281096510767,4.0386478606467));
#22620=CARTESIAN_POINT('Ctrl Pts',(22.066215027555,-90.3816626464359,4.00168013972405));
#22621=CARTESIAN_POINT('Ctrl Pts',(22.598442968768,-89.7456924076384,3.94901908464118));
#22622=CARTESIAN_POINT('Ctrl Pts',(23.4750692458127,-89.3979407209711,3.8963580295583));
#22623=CARTESIAN_POINT('Ctrl Pts',(24.2985288839648,-89.4961188951354,3.84369697447542));
#22624=CARTESIAN_POINT('Ctrl Pts',(25.1219885221169,-89.5942970692997,3.79103591939254));
#22625=CARTESIAN_POINT('Ctrl Pts',(25.8922815213764,-90.1384051042956,3.73837486430966));
#22626=CARTESIAN_POINT('Ctrl Pts',(26.2600668556347,-90.8816807530475,3.68571380922678));
#22627=CARTESIAN_POINT('Ctrl Pts',(26.627852189893,-91.6249564017994,3.6330527541439));
#22628=CARTESIAN_POINT('Ctrl Pts',(26.5931298591502,-92.5673996643073,3.58039169906103));
#22629=CARTESIAN_POINT('Ctrl Pts',(26.1716470433212,-93.2815963706942,3.52773064397815));
#22630=CARTESIAN_POINT('Ctrl Pts',(25.7501642274921,-93.9957930770812,3.47506958889527));
#22631=CARTESIAN_POINT('Ctrl Pts',(24.9419209265769,-94.4817432273472,3.42240853381239));
#22632=CARTESIAN_POINT('Ctrl Pts',(24.1134692499477,-94.5190602709168,3.36974747872951));
#22633=CARTESIAN_POINT('Ctrl Pts',(23.2850175733184,-94.5563773144863,3.31708642364664));
#22634=CARTESIAN_POINT('Ctrl Pts',(22.4363575209751,-94.1450612513594,3.26442536856376));
#22635=CARTESIAN_POINT('Ctrl Pts',(21.9523709530942,-93.4716506583771,3.21176431348088));
#22636=CARTESIAN_POINT('Ctrl Pts',(21.6485266983476,-93.0488869840482,3.17870397648458));
#22637=CARTESIAN_POINT('Ctrl Pts',(21.4884098626544,-92.5228249567292,3.14564363948828));
#22638=CARTESIAN_POINT('Ctrl Pts',(21.4854090148867,-91.9984414282173,3.11258330249198));
#22639=CARTESIAN_POINT('Ctrl Pts',(21.4802713394158,-91.9981710493934,3.38741669750802));
#22640=CARTESIAN_POINT('Ctrl Pts',(21.4861007735321,-92.7096599592594,3.43250787327401));
#22641=CARTESIAN_POINT('Ctrl Pts',(21.802231430593,-93.4256840455739,3.47759904904));
#22642=CARTESIAN_POINT('Ctrl Pts',(22.3356791886479,-93.8943545894189,3.52269022480599));
#22643=CARTESIAN_POINT('Ctrl Pts',(22.958681833701,-94.4417052607172,3.57535127988886));
#22644=CARTESIAN_POINT('Ctrl Pts',(23.8780924613484,-94.6516799768993,3.62801233497174));
#22645=CARTESIAN_POINT('Ctrl Pts',(24.6769426722523,-94.4290516090785,3.68067339005462));
#22646=CARTESIAN_POINT('Ctrl Pts',(25.4757928831562,-94.2064232412577,3.7333344451375));
#22647=CARTESIAN_POINT('Ctrl Pts',(26.1540826773166,-93.5511917894339,3.78599550022038));
#22648=CARTESIAN_POINT('Ctrl Pts',(26.4041960519401,-92.7605159049424,3.83865655530326));
#22649=CARTESIAN_POINT('Ctrl Pts',(26.6543094265636,-91.9698400204509,3.89131761038614));
#22650=CARTESIAN_POINT('Ctrl Pts',(26.4762463816501,-91.0437197032917,3.94397866546901));
#22651=CARTESIAN_POINT('Ctrl Pts',(25.9507615495482,-90.4021663197385,3.99663972055189));
#22652=CARTESIAN_POINT('Ctrl Pts',(25.4252767174463,-89.7606129361853,4.04930077563477));
#22653=CARTESIAN_POINT('Ctrl Pts',(24.5523700981559,-89.4036264862382,4.10196183071765));
#22654=CARTESIAN_POINT('Ctrl Pts',(23.727919739318,-89.4931064186725,4.15462288580053));
#22655=CARTESIAN_POINT('Ctrl Pts',(22.9034693804802,-89.5825863511067,4.2072839408834));
#22656=CARTESIAN_POINT('Ctrl Pts',(22.1274752820949,-90.1185326659223,4.25994499596628));
#22657=CARTESIAN_POINT('Ctrl Pts',(21.7518640115845,-90.8578845621824,4.31260605104916));
#22658=CARTESIAN_POINT('Ctrl Pts',(21.5739987186599,-91.20799397563,4.33754293320211));
#22659=CARTESIAN_POINT('Ctrl Pts',(21.4859136397297,-91.6037142279008,4.36247981535507));
#22660=CARTESIAN_POINT('Ctrl Pts',(21.4864158728456,-91.9996457834086,4.38741669750802));
#22661=CARTESIAN_POINT('Origin',(24.,-92.,5.));
#22662=CARTESIAN_POINT('',(21.4815255054053,-92.0021560919774,5.38741669750802));
#22663=CARTESIAN_POINT('',(21.4785001229596,-91.9995222403937,5.11258330249198));
#22664=CARTESIAN_POINT('',(21.4825,-92.,5.));
#22665=CARTESIAN_POINT('Ctrl Pts',(21.4785001229596,-91.9995222403937,5.11258330249198));
#22666=CARTESIAN_POINT('Ctrl Pts',(21.4784308438678,-91.9731625418826,5.11090963381615));
#22667=CARTESIAN_POINT('Ctrl Pts',(21.4788088040536,-91.9468048777982,5.10923596514032));
#22668=CARTESIAN_POINT('Ctrl Pts',(21.4796401577289,-91.9204615220785,5.10756229646449));
#22669=CARTESIAN_POINT('Ctrl Pts',(21.5057982392643,-91.0915824693399,5.05490124138162));
#22670=CARTESIAN_POINT('Ctrl Pts',(21.9808209826826,-90.2768688588901,5.00224018629874));
#22671=CARTESIAN_POINT('Ctrl Pts',(22.6892774670547,-89.8458072171371,4.94957913121586));
#22672=CARTESIAN_POINT('Ctrl Pts',(23.3977339514269,-89.4147455753841,4.89691807613298));
#22673=CARTESIAN_POINT('Ctrl Pts',(24.3396241767529,-89.367335902328,4.8442570210501));
#22674=CARTESIAN_POINT('Ctrl Pts',(25.0877848515153,-89.7250792935763,4.79159596596723));
#22675=CARTESIAN_POINT('Ctrl Pts',(25.8359455262777,-90.0828226848246,4.73893491088435));
#22676=CARTESIAN_POINT('Ctrl Pts',(26.3903766504766,-90.8457191403772,4.68627385580147));
#22677=CARTESIAN_POINT('Ctrl Pts',(26.4996342472564,-91.6677820984451,4.63361280071859));
#22678=CARTESIAN_POINT('Ctrl Pts',(26.6088918440362,-92.4898450565129,4.58095174563571));
#22679=CARTESIAN_POINT('Ctrl Pts',(26.2729759133969,-93.371074517096,4.52829069055283));
#22680=CARTESIAN_POINT('Ctrl Pts',(25.6442300627918,-93.9118178797764,4.47562963546995));
#22681=CARTESIAN_POINT('Ctrl Pts',(25.0154842121866,-94.4525612424569,4.42296858038708));
#22682=CARTESIAN_POINT('Ctrl Pts',(24.0939084416155,-94.6528185072348,4.3703075253042));
#22683=CARTESIAN_POINT('Ctrl Pts',(23.2974530904191,-94.4217695888032,4.31764647022132));
#22684=CARTESIAN_POINT('Ctrl Pts',(22.5009977392227,-94.1907206703715,4.26498541513844));
#22685=CARTESIAN_POINT('Ctrl Pts',(21.8296628074011,-93.5283655687303,4.21232436005556));
#22686=CARTESIAN_POINT('Ctrl Pts',(21.5879101441809,-92.7350936224457,4.15966330497269));
#22687=CARTESIAN_POINT('Ctrl Pts',(21.5158662908614,-92.4986934646177,4.14396997081245));
#22688=CARTESIAN_POINT('Ctrl Pts',(21.4819727131382,-92.2506668639209,4.12827663665222));
#22689=CARTESIAN_POINT('Ctrl Pts',(21.4839749917546,-92.0021063689016,4.11258330249198));
#22690=CARTESIAN_POINT('Ctrl Pts',(21.4864158728456,-91.9996457834086,4.38741669750802));
#22691=CARTESIAN_POINT('Ctrl Pts',(21.4869742424795,-92.4398321245071,4.41514087043795));
#22692=CARTESIAN_POINT('Ctrl Pts',(21.5970301658382,-92.8802796450794,4.44286504336787));
#22693=CARTESIAN_POINT('Ctrl Pts',(21.8149443593501,-93.2586003903179,4.47058921629779));
#22694=CARTESIAN_POINT('Ctrl Pts',(22.2288644202614,-93.9772068444889,4.52325027138067));
#22695=CARTESIAN_POINT('Ctrl Pts',(23.0319329847194,-94.4716622751266,4.57591132646355));
#22696=CARTESIAN_POINT('Ctrl Pts',(23.8599447536685,-94.517722705864,4.62857238154643));
#22697=CARTESIAN_POINT('Ctrl Pts',(24.6879565226175,-94.5637831366015,4.68123343662931));
#22698=CARTESIAN_POINT('Ctrl Pts',(25.5409114960577,-94.1614485674387,4.73389449171218));
#22699=CARTESIAN_POINT('Ctrl Pts',(26.0319800368686,-93.4931845918408,4.78655554679506));
#22700=CARTESIAN_POINT('Ctrl Pts',(26.5230485776795,-92.8249206162428,4.83921660187794));
#22701=CARTESIAN_POINT('Ctrl Pts',(26.6522306858613,-91.8907272342096,4.89187765696082));
#22702=CARTESIAN_POINT('Ctrl Pts',(26.3609400707586,-91.1142770874653,4.9445387120437));
#22703=CARTESIAN_POINT('Ctrl Pts',(26.0696494556558,-90.337826940721,4.99719976712657));
#22704=CARTESIAN_POINT('Ctrl Pts',(25.3578861172687,-89.7191200292656,5.04986082220945));
#22705=CARTESIAN_POINT('Ctrl Pts',(24.5484468765423,-89.5387504963611,5.10252187729233));
#22706=CARTESIAN_POINT('Ctrl Pts',(23.7390076358159,-89.3583809634566,5.15518293237521));
#22707=CARTESIAN_POINT('Ctrl Pts',(22.8318924927503,-89.616348809103,5.20784398745809));
#22708=CARTESIAN_POINT('Ctrl Pts',(22.2384936456262,-90.1956612127896,5.26050504254097));
#22709=CARTESIAN_POINT('Ctrl Pts',(21.7618021600142,-90.6610367214971,5.30280892752998));
#22710=CARTESIAN_POINT('Ctrl Pts',(21.48756099645,-91.3337852933997,5.345112812519));
#22711=CARTESIAN_POINT('Ctrl Pts',(21.4815255054053,-92.0021560919774,5.38741669750802));
#22712=CARTESIAN_POINT('Origin',(24.,-92.,5.));
#22713=CARTESIAN_POINT('',(21.4800391863945,-91.998264576152,6.38741669750802));
#22714=CARTESIAN_POINT('',(21.4852341727342,-91.998341042672,6.11258330249198));
#22715=CARTESIAN_POINT('',(21.4825,-92.,5.));
#22716=CARTESIAN_POINT('Ctrl Pts',(21.4852341727342,-91.998341042672,6.11258330249198));
#22717=CARTESIAN_POINT('Ctrl Pts',(21.483386156444,-91.696381980717,6.09354263098009));
#22718=CARTESIAN_POINT('Ctrl Pts',(21.533738485222,-91.3950185131866,6.07450195946819));
#22719=CARTESIAN_POINT('Ctrl Pts',(21.6390604846241,-91.1142772958209,6.0554612879563));
#22720=CARTESIAN_POINT('Ctrl Pts',(21.9303510312042,-90.3378273317271,6.00280023287342));
#22721=CARTESIAN_POINT('Ctrl Pts',(22.6421142021576,-89.719120565815,5.95013917779055));
#22722=CARTESIAN_POINT('Ctrl Pts',(23.4515532524732,-89.5387510753403,5.89747812270767));
#22723=CARTESIAN_POINT('Ctrl Pts',(24.2609923027888,-89.3583815848656,5.84481706762479));
#22724=CARTESIAN_POINT('Ctrl Pts',(25.1681072324665,-89.6163493698282,5.79215601254191));
#22725=CARTESIAN_POINT('Ctrl Pts',(25.7615059400007,-90.1956616372385,5.73949495745904));
#22726=CARTESIAN_POINT('Ctrl Pts',(26.3549046475349,-90.7749739046489,5.68683390237615));
#22727=CARTESIAN_POINT('Ctrl Pts',(26.6345871329256,-91.675630654507,5.63417284729328));
#22728=CARTESIAN_POINT('Ctrl Pts',(26.47371261597,-92.4891686800902,5.5815117922104));
#22729=CARTESIAN_POINT('Ctrl Pts',(26.3128380990145,-93.3027067056733,5.52885073712752));
#22730=CARTESIAN_POINT('Ctrl Pts',(25.7114065797126,-94.0291260069815,5.47618968204464));
#22731=CARTESIAN_POINT('Ctrl Pts',(24.9421775161413,-94.3389830337326,5.42352862696176));
#22732=CARTESIAN_POINT('Ctrl Pts',(24.17294845257,-94.6488400604838,5.37086757187889));
#22733=CARTESIAN_POINT('Ctrl Pts',(23.2359218447291,-94.5421348126778,5.31820651679601));
#22734=CARTESIAN_POINT('Ctrl Pts',(22.556055250635,-94.0672599412612,5.26554546171313));
#22735=CARTESIAN_POINT('Ctrl Pts',(21.8977961123825,-93.6074774981291,5.21455807530608));
#22736=CARTESIAN_POINT('Ctrl Pts',(21.4806106720036,-92.8025558114754,5.16357068889903));
#22737=CARTESIAN_POINT('Ctrl Pts',(21.4785001229596,-91.9995222403937,5.11258330249198));
#22738=CARTESIAN_POINT('Ctrl Pts',(21.4815255054053,-92.0021560919774,5.38741669750802));
#22739=CARTESIAN_POINT('Ctrl Pts',(21.4800478489828,-92.1657918915838,5.39777386760188));
#22740=CARTESIAN_POINT('Ctrl Pts',(21.494646624663,-92.3291652844524,5.40813103769574));
#22741=CARTESIAN_POINT('Ctrl Pts',(21.5262868021188,-92.4891687951612,5.4184882077896));
#22742=CARTESIAN_POINT('Ctrl Pts',(21.6871613569182,-93.3027070121194,5.47114926287248));
#22743=CARTESIAN_POINT('Ctrl Pts',(22.2885930176996,-94.0291264843089,5.52381031795536));
#22744=CARTESIAN_POINT('Ctrl Pts',(23.0578222622228,-94.3389835839502,5.57647137303824));
#22745=CARTESIAN_POINT('Ctrl Pts',(23.827051506746,-94.6488406835915,5.62913242812111));
#22746=CARTESIAN_POINT('Ctrl Pts',(24.7640783350111,-94.5421354106846,5.68179348320399));
#22747=CARTESIAN_POINT('Ctrl Pts',(25.4439450890356,-94.0672604275592,5.73445453828687));
#22748=CARTESIAN_POINT('Ctrl Pts',(26.1238118430602,-93.5923854444339,5.78711559336975));
#22749=CARTESIAN_POINT('Ctrl Pts',(26.5465185228442,-92.7493407510902,5.83977664845263));
#22750=CARTESIAN_POINT('Ctrl Pts',(26.5203604351554,-91.9204615033679,5.8924377035355));
#22751=CARTESIAN_POINT('Ctrl Pts',(26.4942023474666,-91.0915822556456,5.94509875861838));
#22752=CARTESIAN_POINT('Ctrl Pts',(26.019179492305,-90.2768684535448,5.99775981370126));
#22753=CARTESIAN_POINT('Ctrl Pts',(25.310722841277,-89.8458067103895,6.05042086878414));
#22754=CARTESIAN_POINT('Ctrl Pts',(24.602266190249,-89.4147449672342,6.10308192386702));
#22755=CARTESIAN_POINT('Ctrl Pts',(23.6603757433546,-89.3673352830245,6.15574297894989));
#22756=CARTESIAN_POINT('Ctrl Pts',(22.9122148925964,-89.7250787584281,6.20840403403277));
#22757=CARTESIAN_POINT('Ctrl Pts',(22.1640540418382,-90.0828222338316,6.26106508911565));
#22758=CARTESIAN_POINT('Ctrl Pts',(21.6096227872161,-90.8457188688485,6.31372614419853));
#22759=CARTESIAN_POINT('Ctrl Pts',(21.5003651647348,-91.6677820202957,6.36638719928141));
#22760=CARTESIAN_POINT('Ctrl Pts',(21.4858216342605,-91.7772087149585,6.37339703202361));
#22761=CARTESIAN_POINT('Ctrl Pts',(21.4791660807206,-91.8876837738621,6.38040686476582));
#22762=CARTESIAN_POINT('Ctrl Pts',(21.4800391863945,-91.998264576152,6.38741669750802));
#22763=CARTESIAN_POINT('Origin',(24.,-92.,5.));
#22764=CARTESIAN_POINT('',(21.4863708146038,-91.9995053986078,7.38741669750802));
#22765=CARTESIAN_POINT('',(21.4842078764603,-92.0020516719096,7.11258330249198));
#22766=CARTESIAN_POINT('',(21.4825,-92.,5.));
#22767=CARTESIAN_POINT('Ctrl Pts',(21.4842078764603,-92.0020516719096,7.11258330249198));
#22768=CARTESIAN_POINT('Ctrl Pts',(21.4887016384805,-91.4252697537026,7.07617562814403));
#22769=CARTESIAN_POINT('Ctrl Pts',(21.6859405266728,-90.8457100529155,7.03976795379607));
#22770=CARTESIAN_POINT('Ctrl Pts',(22.0492389093472,-90.402166695613,7.00336027944811));
#22771=CARTESIAN_POINT('Ctrl Pts',(22.5747236178373,-89.7606134629807,6.95069922436523));
#22772=CARTESIAN_POINT('Ctrl Pts',(23.4476300317824,-89.4036270970037,6.89803816928235));
#22773=CARTESIAN_POINT('Ctrl Pts',(24.2720801966772,-89.4931070083872,6.84537711419947));
#22774=CARTESIAN_POINT('Ctrl Pts',(25.096530361572,-89.5825869197707,6.79271605911659));
#22775=CARTESIAN_POINT('Ctrl Pts',(25.8725242774164,-90.1185331085148,6.74005500403372));
#22776=CARTESIAN_POINT('Ctrl Pts',(26.2481354595693,-90.8578848308521,6.68739394895084));
#22777=CARTESIAN_POINT('Ctrl Pts',(26.6237466417222,-91.5972365531893,6.63473289386796));
#22778=CARTESIAN_POINT('Ctrl Pts',(26.5989750901836,-92.5399938091198,6.58207183878508));
#22779=CARTESIAN_POINT('Ctrl Pts',(26.1850551266417,-93.2586000942469,6.52941078370221));
#22780=CARTESIAN_POINT('Ctrl Pts',(25.7711351630998,-93.9772063793741,6.47674972861933));
#22781=CARTESIAN_POINT('Ctrl Pts',(24.9680667875545,-94.4716616936979,6.42408867353644));
#22782=CARTESIAN_POINT('Ctrl Pts',(24.1400552133854,-94.5177221136004,6.37142761845357));
#22783=CARTESIAN_POINT('Ctrl Pts',(23.3120436392162,-94.5637825335029,6.31876656337069));
#22784=CARTESIAN_POINT('Ctrl Pts',(22.4590888664231,-94.1614480589841,6.26610550828782));
#22785=CARTESIAN_POINT('Ctrl Pts',(21.96802044113,-93.4931842405871,6.21344445320494));
#22786=CARTESIAN_POINT('Ctrl Pts',(21.6545077552948,-93.0665447464531,6.17982406963395));
#22787=CARTESIAN_POINT('Ctrl Pts',(21.4884972412917,-92.5315144383331,6.14620368606297));
#22788=CARTESIAN_POINT('Ctrl Pts',(21.4852341727342,-91.998341042672,6.11258330249198));
#22789=CARTESIAN_POINT('Ctrl Pts',(21.4800391863945,-91.998264576152,6.38741669750802));
#22790=CARTESIAN_POINT('Ctrl Pts',(21.4857252480609,-92.7184171072604,6.4330679198487));
#22791=CARTESIAN_POINT('Ctrl Pts',(21.8107173609326,-93.4430544346852,6.47871914218937));
#22792=CARTESIAN_POINT('Ctrl Pts',(22.3557695504229,-93.9118183295065,6.52437036453004));
#22793=CARTESIAN_POINT('Ctrl Pts',(22.9845155489329,-94.4525618193924,6.57703141961292));
#22794=CARTESIAN_POINT('Ctrl Pts',(23.9060915362935,-94.6528191312864,6.6296924746958));
#22795=CARTESIAN_POINT('Ctrl Pts',(24.7025470748465,-94.4217701584994,6.68235352977868));
#22796=CARTESIAN_POINT('Ctrl Pts',(25.4990026133996,-94.1907211857124,6.73501458486155));
#22797=CARTESIAN_POINT('Ctrl Pts',(26.170337703145,-93.5283659282443,6.78767563994443));
#22798=CARTESIAN_POINT('Ctrl Pts',(26.4120904232343,-92.7350937953596,6.84033669502731));
#22799=CARTESIAN_POINT('Ctrl Pts',(26.6538431433236,-91.941821662475,6.89299775011019));
#22800=CARTESIAN_POINT('Ctrl Pts',(26.4660134937569,-91.0176326541737,6.94565880519307));
#22801=CARTESIAN_POINT('Ctrl Pts',(25.9337854273443,-90.3816622657573,6.99831986027595));
#22802=CARTESIAN_POINT('Ctrl Pts',(25.4015573609318,-89.7456918773409,7.05098091535883));
#22803=CARTESIAN_POINT('Ctrl Pts',(24.5249308776734,-89.3979401088093,7.1036419704417));
#22804=CARTESIAN_POINT('Ctrl Pts',(23.7014710458108,-89.4961183060969,7.15630302552458));
#22805=CARTESIAN_POINT('Ctrl Pts',(22.8780112139481,-89.5942965033845,7.20896408060746));
#22806=CARTESIAN_POINT('Ctrl Pts',(22.1077180334812,-90.1384046664913,7.26162513569034));
#22807=CARTESIAN_POINT('Ctrl Pts',(21.7399326127095,-90.8816804900357,7.31428619077321));
#22808=CARTESIAN_POINT('Ctrl Pts',(21.569684509702,-91.2257433370738,7.33866302635148));
#22809=CARTESIAN_POINT('Ctrl Pts',(21.4856845592314,-91.6124832315577,7.36303986192975));
#22810=CARTESIAN_POINT('Ctrl Pts',(21.4863708146038,-91.9995053986078,7.38741669750802));
#22811=CARTESIAN_POINT('Origin',(24.,-92.,5.));
#22812=CARTESIAN_POINT('',(21.4817891743669,-92.002194435609,8.38741669750802));
#22813=CARTESIAN_POINT('',(21.4784371162896,-91.9996804085349,8.11258330249198));
#22814=CARTESIAN_POINT('',(21.4825,-92.,5.));
#22815=CARTESIAN_POINT('Ctrl Pts',(21.4784371162896,-91.9996804085349,8.11258330249198));
#22816=CARTESIAN_POINT('Ctrl Pts',(21.4784054922,-91.9821424240367,8.11146968039084));
#22817=CARTESIAN_POINT('Ctrl Pts',(21.4785728027446,-91.9646050586431,8.11035605828969));
#22818=CARTESIAN_POINT('Ctrl Pts',(21.4789408989108,-91.9470719086913,8.10924243618855));
#22819=CARTESIAN_POINT('Ctrl Pts',(21.496347461212,-91.1179628469758,8.05658138110567));
#22820=CARTESIAN_POINT('Ctrl Pts',(21.9627433725619,-90.298280199785,8.00392032602279));
#22821=CARTESIAN_POINT('Ctrl Pts',(22.6666099349663,-89.8597638322688,7.95125927093991));
#22822=CARTESIAN_POINT('Ctrl Pts',(23.3704764973707,-89.4212474647526,7.89859821585703));
#22823=CARTESIAN_POINT('Ctrl Pts',(24.3118137108296,-89.3638973769109,7.84593716077416));
#22824=CARTESIAN_POINT('Ctrl Pts',(25.0637091784649,-89.7137229122891,7.79327610569128));
#22825=CARTESIAN_POINT('Ctrl Pts',(25.8156046461002,-90.0635484476673,7.7406150506084));
#22826=CARTESIAN_POINT('Ctrl Pts',(26.378058367912,-90.8205496062653,7.68795399552553));
#22827=CARTESIAN_POINT('Ctrl Pts',(26.4959879359715,-91.6414133946616,7.63529294044265));
#22828=CARTESIAN_POINT('Ctrl Pts',(26.6139175040309,-92.462277183058,7.58263188535977));
#22829=CARTESIAN_POINT('Ctrl Pts',(26.2873229183381,-93.3470036012526,7.52997083027689));
#22830=CARTESIAN_POINT('Ctrl Pts',(25.6643204198242,-93.8943541437692,7.47730977519401));
#22831=CARTESIAN_POINT('Ctrl Pts',(25.0413179213102,-94.4417046862858,7.42464872011113));
#22832=CARTESIAN_POINT('Ctrl Pts',(24.1219075099752,-94.6516793531244,7.37198766502826));
#22833=CARTESIAN_POINT('Ctrl Pts',(23.3230574869989,-94.4290510376866,7.31932660994538));
#22834=CARTESIAN_POINT('Ctrl Pts',(22.5242074640225,-94.2064227222488,7.2666655548625));
#22835=CARTESIAN_POINT('Ctrl Pts',(21.8459178294048,-93.5511914245345,7.21400449977962));
#22836=CARTESIAN_POINT('Ctrl Pts',(21.5958045136134,-92.7605157260336,7.16134344469674));
#22837=CARTESIAN_POINT('Ctrl Pts',(21.5186091945673,-92.5164804869872,7.14509006396182));
#22838=CARTESIAN_POINT('Ctrl Pts',(21.4822017382943,-92.2595428818133,7.1288366832269));
#22839=CARTESIAN_POINT('Ctrl Pts',(21.4842078764603,-92.0020516719096,7.11258330249198));
#22840=CARTESIAN_POINT('Ctrl Pts',(21.4863708146038,-91.9995053986078,7.38741669750802));
#22841=CARTESIAN_POINT('Ctrl Pts',(21.4871670704398,-92.4485636814537,7.41570091701263));
#22842=CARTESIAN_POINT('Ctrl Pts',(21.6019742377664,-92.8980019807643,7.44398513651724));
#22843=CARTESIAN_POINT('Ctrl Pts',(21.8283524458306,-93.2815966720593,7.47226935602185));
#22844=CARTESIAN_POINT('Ctrl Pts',(22.2498353607997,-93.9957935465564,7.52493041110473));
#22845=CARTESIAN_POINT('Ctrl Pts',(23.0580788518144,-94.4817438115688,7.57759146618761));
#22846=CARTESIAN_POINT('Ctrl Pts',(23.8865307233467,-94.5190608637177,7.63025252127049));
#22847=CARTESIAN_POINT('Ctrl Pts',(24.714982594879,-94.5563779158666,7.68291357635336));
#22848=CARTESIAN_POINT('Ctrl Pts',(25.5636428469288,-94.1450617551521,7.73557463143624));
#22849=CARTESIAN_POINT('Ctrl Pts',(26.0476295286171,-93.4716510041371,7.78823568651912));
#22850=CARTESIAN_POINT('Ctrl Pts',(26.5316162103055,-92.798240253122,7.840896741602));
#22851=CARTESIAN_POINT('Ctrl Pts',(26.6509293216325,-91.8627349118065,7.89355779668488));
#22852=CARTESIAN_POINT('Ctrl Pts',(26.3514584187992,-91.0894031813449,7.94621885176775));
#22853=CARTESIAN_POINT('Ctrl Pts',(26.0519875159658,-90.3160714508833,7.99887990685063));
#22854=CARTESIAN_POINT('Ctrl Pts',(25.3337325989722,-89.7049133312758,8.0515409619335));
#22855=CARTESIAN_POINT('Ctrl Pts',(24.5224343499209,-89.5330983089572,8.10420201701638));
#22856=CARTESIAN_POINT('Ctrl Pts',(23.7111361008695,-89.3612832866386,8.15686307209926));
#22857=CARTESIAN_POINT('Ctrl Pts',(22.8067945197604,-89.6288113616089,8.20952412718214));
#22858=CARTESIAN_POINT('Ctrl Pts',(22.2195443159446,-90.2143563368687,8.26218518226502));
#22859=CARTESIAN_POINT('Ctrl Pts',(21.7540375466957,-90.6785113902208,8.30392902067935));
#22860=CARTESIAN_POINT('Ctrl Pts',(21.4877769931074,-91.3424942170044,8.34567285909369));
#22861=CARTESIAN_POINT('Ctrl Pts',(21.4817891743669,-92.002194435609,8.38741669750802));
#22862=CARTESIAN_POINT('Origin',(24.,-92.,5.));
#22863=CARTESIAN_POINT('',(21.4798238762261,-91.9984131135315,9.38741669750802));
#22864=CARTESIAN_POINT('',(21.4850512338518,-91.9982506073194,9.11258330249198));
#22865=CARTESIAN_POINT('',(21.4825,-92.,5.));
#22866=CARTESIAN_POINT('',(25.913465996665,-90.364012796625,10.));
#22867=CARTESIAN_POINT('Ctrl Pts',(21.4798238762261,-91.9984131135315,9.38741669750802));
#22868=CARTESIAN_POINT('Ctrl Pts',(21.4853062059344,-92.7270927102602,9.43362796642338));
#22869=CARTESIAN_POINT('Ctrl Pts',(21.8192672097013,-93.4600319638108,9.47983923533874));
#22870=CARTESIAN_POINT('Ctrl Pts',(22.3760118920419,-93.9288769835329,9.5260505042541));
#22871=CARTESIAN_POINT('Ctrl Pts',(23.0104623858715,-94.4631595078699,9.57871155933697));
#22872=CARTESIAN_POINT('Ctrl Pts',(23.9342250444886,-94.6544830013391,9.63137261441985));
#22873=CARTESIAN_POINT('Ctrl Pts',(24.7281293690809,-94.4146106072968,9.68403366950273));
#22874=CARTESIAN_POINT('Ctrl Pts',(25.5220336936733,-94.1747382132545,9.73669472458561));
#22875=CARTESIAN_POINT('Ctrl Pts',(26.186079684241,-93.5036699317008,9.78935577966849));
#22876=CARTESIAN_POINT('Ctrl Pts',(26.4192662809857,-92.7092700865749,9.84201683475137));
#22877=CARTESIAN_POINT('Ctrl Pts',(26.6524528777304,-91.9148702414489,9.89467788983425));
#22878=CARTESIAN_POINT('Ctrl Pts',(26.4547800806522,-90.9971388327508,9.94733894491712));
#22879=CARTESIAN_POINT('Ctrl Pts',(25.913465996665,-90.364012796625,10.));
#22880=CARTESIAN_POINT('',(22.0828970444786,-90.361465706548,10.));
#22881=CARTESIAN_POINT('Origin',(24.,-92.,10.));
#22882=CARTESIAN_POINT('Ctrl Pts',(22.0828885913556,-90.3614597865289,10.));
#22883=CARTESIAN_POINT('Ctrl Pts',(22.6060434082611,-89.752303655963,9.94901908464118));
#22884=CARTESIAN_POINT('Ctrl Pts',(23.4465814718894,-89.4121729024441,9.89803816928235));
#22885=CARTESIAN_POINT('Ctrl Pts',(24.2457357606074,-89.490515472492,9.84705725392353));
#22886=CARTESIAN_POINT('Ctrl Pts',(25.0712271767912,-89.57143991976,9.79439619884065));
#22887=CARTESIAN_POINT('Ctrl Pts',(25.8525621626002,-90.0988748222943,9.74173514375777));
#22888=CARTESIAN_POINT('Ctrl Pts',(26.2358875787344,-90.8341463056131,9.68907408867489));
#22889=CARTESIAN_POINT('Ctrl Pts',(26.6192129948686,-91.5694177889319,9.63641303359202));
#22890=CARTESIAN_POINT('Ctrl Pts',(26.6045288413281,-92.5125258530351,9.58375197850914));
#22891=CARTESIAN_POINT('Ctrl Pts',(26.1982520122281,-93.235497804129,9.53109092342626));
#22892=CARTESIAN_POINT('Ctrl Pts',(25.7919751831282,-93.9584697552228,9.47842986834338));
#22893=CARTESIAN_POINT('Ctrl Pts',(24.9941056784689,-94.4613055933072,9.4257688132605));
#22894=CARTESIAN_POINT('Ctrl Pts',(24.1666097496597,-94.5160865743966,9.37310775817762));
#22895=CARTESIAN_POINT('Ctrl Pts',(23.3391138208506,-94.5708675554859,9.32044670309475));
#22896=CARTESIAN_POINT('Ctrl Pts',(22.4819914678916,-94.1775936795802,9.26778564801187));
#22897=CARTESIAN_POINT('Ctrl Pts',(21.9839041146304,-93.5145597074388,9.21512459292899));
#22898=CARTESIAN_POINT('Ctrl Pts',(21.6606132128853,-93.0842077835489,9.18094416278332));
#22899=CARTESIAN_POINT('Ctrl Pts',(21.4885783498304,-92.5402099934131,9.14676373263765));
#22900=CARTESIAN_POINT('Ctrl Pts',(21.4850512338518,-91.9982506073194,9.11258330249198));
#22901=CARTESIAN_POINT('Origin',(24.,-92.,12.2084234471775));
#22902=CARTESIAN_POINT('',(20.9217237789782,-91.9992118506711,1.79157655282254));
#22903=CARTESIAN_POINT('',(20.9313888204345,-91.9996651715868,1.70842344717745));
#22904=CARTESIAN_POINT('',(20.9265,-91.9999999999999,12.2084234471775));
#22905=CARTESIAN_POINT('',(24.7937992825329,-94.9692229537457,0.999999999999999));
#22906=CARTESIAN_POINT('Ctrl Pts',(20.9313888204345,-91.9996651715868,1.70842344717745));
#22907=CARTESIAN_POINT('Ctrl Pts',(20.9310463723584,-91.5053847152746,1.68292651844981));
#22908=CARTESIAN_POINT('Ctrl Pts',(21.2764430280356,-89.9907712812588,1.6047685346393));
#22909=CARTESIAN_POINT('Ctrl Pts',(23.6460838609915,-88.3911589633379,1.4739494957459));
#22910=CARTESIAN_POINT('Ctrl Pts',(26.8312242725849,-89.7301456837401,1.31596633049727));
#22911=CARTESIAN_POINT('Ctrl Pts',(27.4433140827682,-93.1332953965992,1.15798316524863));
#22912=CARTESIAN_POINT('Ctrl Pts',(25.7762533017603,-94.7065713079336,1.05266105508288));
#22913=CARTESIAN_POINT('Ctrl Pts',(24.7937992825328,-94.9692229537457,0.999999999999999));
#22914=CARTESIAN_POINT('',(23.2062007174671,-94.9692229537457,0.999999999999999));
#22915=CARTESIAN_POINT('Origin',(24.,-92.,0.999999999999999));
#22916=CARTESIAN_POINT('Ctrl Pts',(20.9217237789782,-91.9992118506711,1.79157655282254));
#22917=CARTESIAN_POINT('Ctrl Pts',(20.9215776858271,-91.9562584671078,1.78934283757203));
#22918=CARTESIAN_POINT('Ctrl Pts',(20.9417782923113,-90.9007977729437,1.73444806723864));
#22919=CARTESIAN_POINT('Ctrl Pts',(22.1476053652116,-88.8820474355396,1.62689224182237));
#22920=CARTESIAN_POINT('Ctrl Pts',(25.5990313571955,-88.7444874247256,1.46890907657374));
#22921=CARTESIAN_POINT('Ctrl Pts',(27.5999505159819,-91.5606294856851,1.3109259113251));
#22922=CARTESIAN_POINT('Ctrl Pts',(26.3493022691421,-94.7394085052657,1.15462288580052));
#22923=CARTESIAN_POINT('Ctrl Pts',(24.1519061796922,-95.2254057458095,1.05098091535882));
#22924=CARTESIAN_POINT('Ctrl Pts',(23.2042985533737,-94.9743125149969,1.));
#22925=CARTESIAN_POINT('Origin',(24.,-92.,12.2084234471775));
#22926=CARTESIAN_POINT('',(20.930051482524,-91.9980972113707,2.79157655282254));
#22927=CARTESIAN_POINT('',(20.9249913784601,-92.002575532166,2.70842344717745));
#22928=CARTESIAN_POINT('',(20.9265,-91.9999999999999,12.2084234471775));
#22929=CARTESIAN_POINT('Ctrl Pts',(20.9249913784601,-92.002575532166,2.70842344717745));
#22930=CARTESIAN_POINT('Ctrl Pts',(20.9323854338683,-91.1760102376998,2.66555951561375));
#22931=CARTESIAN_POINT('Ctrl Pts',(21.7006357273797,-89.3218326978092,2.57003452896717));
#22932=CARTESIAN_POINT('Ctrl Pts',(24.8261378655289,-88.4685618660265,2.42184848723771));
#22933=CARTESIAN_POINT('Ctrl Pts',(27.4089767382702,-90.7619776329038,2.26386532198907));
#22934=CARTESIAN_POINT('Ctrl Pts',(26.8996888283721,-94.1783943608088,2.10588215674044));
#22935=CARTESIAN_POINT('Ctrl Pts',(23.7604241409854,-95.6187851374897,1.9478989914918));
#22936=CARTESIAN_POINT('Ctrl Pts',(21.309798993458,-94.0743436082074,1.81541275497081));
#22937=CARTESIAN_POINT('Ctrl Pts',(20.9317536605653,-92.5262657246815,1.73558757353269));
#22938=CARTESIAN_POINT('Ctrl Pts',(20.9313888204345,-91.9996651715868,1.70842344717745));
#22939=CARTESIAN_POINT('Ctrl Pts',(20.930051482524,-91.9980972113706,2.79157655282254));
#22940=CARTESIAN_POINT('Ctrl Pts',(20.9278794195688,-91.6185397913436,2.77197583473597));
#22941=CARTESIAN_POINT('Ctrl Pts',(21.1684425268396,-90.2218847391137,2.69971406156651));
#22942=CARTESIAN_POINT('Ctrl Pts',(23.2485917742673,-88.4519002035991,2.57479123331418));
#22943=CARTESIAN_POINT('Ctrl Pts',(26.5607981614372,-89.4317381309793,2.41680806806554));
#22944=CARTESIAN_POINT('Ctrl Pts',(27.5502714048858,-92.7410888412383,2.25882490281691));
#22945=CARTESIAN_POINT('Ctrl Pts',(25.3195309927208,-95.3782229777193,2.10084173756827));
#22946=CARTESIAN_POINT('Ctrl Pts',(21.9403861581344,-94.9572790184773,1.94509228757015));
#22947=CARTESIAN_POINT('Ctrl Pts',(20.9250219115291,-92.96890790723,1.84200389265491));
#22948=CARTESIAN_POINT('Ctrl Pts',(20.9217237789782,-91.9992118506711,1.79157655282254));
#22949=CARTESIAN_POINT('Origin',(24.,-92.,12.2084234471775));
#22950=CARTESIAN_POINT('',(20.9283007496159,-92.002571568945,3.79157655282255));
#22951=CARTESIAN_POINT('',(20.9237791307624,-91.9977671182961,3.70842344717745));
#22952=CARTESIAN_POINT('',(20.9265,-91.9999999999999,12.2084234471775));
#22953=CARTESIAN_POINT('Ctrl Pts',(20.9237791307624,-91.9977671182962,3.70842344717745));
#22954=CARTESIAN_POINT('Ctrl Pts',(20.9225843518948,-91.8519430302088,3.70085356786056));
#22955=CARTESIAN_POINT('Ctrl Pts',(20.9980297211289,-90.6929123616699,3.6406226334608));
#22956=CARTESIAN_POINT('Ctrl Pts',(22.4700852939276,-88.7116866521341,3.52773064397815));
#22957=CARTESIAN_POINT('Ctrl Pts',(25.9177920746621,-88.9217349563625,3.36974747872952));
#22958=CARTESIAN_POINT('Ctrl Pts',(27.6259964474171,-91.9238742346134,3.21176431348088));
#22959=CARTESIAN_POINT('Ctrl Pts',(26.0452973355111,-94.9950631778383,3.05378114823225));
#22960=CARTESIAN_POINT('Ctrl Pts',(22.6094456576622,-95.3496255535895,2.89579798298361));
#22961=CARTESIAN_POINT('Ctrl Pts',(21.0248752439865,-93.3940964847872,2.78067874929868));
#22962=CARTESIAN_POINT('Ctrl Pts',(20.923301368433,-92.1914980595947,2.71822057069663));
#22963=CARTESIAN_POINT('Ctrl Pts',(20.9249913784601,-92.002575532166,2.70842344717745));
#22964=CARTESIAN_POINT('Ctrl Pts',(20.9283007496159,-92.002571568945,3.79157655282255));
#22965=CARTESIAN_POINT('Ctrl Pts',(20.934059068375,-91.2877407010241,3.7546088318999));
#22966=CARTESIAN_POINT('Ctrl Pts',(21.5376069996117,-89.5458537101333,3.66498005589438));
#22967=CARTESIAN_POINT('Ctrl Pts',(24.429368893546,-88.3987114188411,3.52269022480599));
#22968=CARTESIAN_POINT('Ctrl Pts',(27.2506148119859,-90.3915408673734,3.36470705955735));
#22969=CARTESIAN_POINT('Ctrl Pts',(27.1234421205799,-93.8432978095595,3.20672389430872));
#22970=CARTESIAN_POINT('Ctrl Pts',(24.1632008669201,-95.6231203956682,3.04874072906008));
#22971=CARTESIAN_POINT('Ctrl Pts',(21.4405688436026,-94.3035551797938,2.91035828189803));
#22972=CARTESIAN_POINT('Ctrl Pts',(20.9337150795902,-92.6382929511448,2.82463688981885));
#22973=CARTESIAN_POINT('Ctrl Pts',(20.930051482524,-91.9980972113706,2.79157655282254));
#22974=CARTESIAN_POINT('Origin',(24.,-92.,12.2084234471775));
#22975=CARTESIAN_POINT('',(20.9216167340284,-91.9994167252631,4.79157655282255));
#22976=CARTESIAN_POINT('',(20.9312807091126,-91.9995675532498,4.70842344717745));
#22977=CARTESIAN_POINT('',(20.9265,-91.9999999999999,12.2084234471775));
#22978=CARTESIAN_POINT('Ctrl Pts',(20.9312807091126,-91.9995675532498,4.70842344717746));
#22979=CARTESIAN_POINT('Ctrl Pts',(20.9306675557931,-91.5161929213319,4.6834865650245));
#22980=CARTESIAN_POINT('Ctrl Pts',(21.2653046726707,-90.0128431381642,4.60588862778867));
#22981=CARTESIAN_POINT('Ctrl Pts',(23.6086716990241,-88.3943786103439,4.47562963546995));
#22982=CARTESIAN_POINT('Ctrl Pts',(26.8057463695968,-89.7018636398323,4.31764647022133));
#22983=CARTESIAN_POINT('Ctrl Pts',(27.4579133231717,-93.0938367815869,4.15966330497269));
#22984=CARTESIAN_POINT('Ctrl Pts',(24.9736348536359,-95.4936626411861,4.00168013972405));
#22985=CARTESIAN_POINT('Ctrl Pts',(21.7675877362369,-94.761466587215,3.85126685379231));
#22986=CARTESIAN_POINT('Ctrl Pts',(20.9308960188484,-92.8663912154057,3.75351462294344));
#22987=CARTESIAN_POINT('Ctrl Pts',(20.9237791307624,-91.9977671182962,3.70842344717745));
#22988=CARTESIAN_POINT('Ctrl Pts',(20.9216167340284,-91.9994167252631,4.79157655282255));
#22989=CARTESIAN_POINT('Ctrl Pts',(20.9215321543705,-91.9672353813212,4.78990288414672));
#22990=CARTESIAN_POINT('Ctrl Pts',(20.9365123597457,-90.9225665616792,4.73556816038801));
#22991=CARTESIAN_POINT('Ctrl Pts',(22.1148106026499,-88.9016620282347,4.62857238154642));
#22992=CARTESIAN_POINT('Ctrl Pts',(25.564542011833,-88.7280211581599,4.4705892162978));
#22993=CARTESIAN_POINT('Ctrl Pts',(27.595180415279,-91.5221767762026,4.31260605104916));
#22994=CARTESIAN_POINT('Ctrl Pts',(26.3648674705088,-94.7497343695717,4.15462288580052));
#22995=CARTESIAN_POINT('Ctrl Pts',(22.9895390126931,-95.4831890308962,3.99663972055189));
#22996=CARTESIAN_POINT('Ctrl Pts',(21.1060884403934,-93.6249316453216,3.8756242762259));
#22997=CARTESIAN_POINT('Ctrl Pts',(20.9258562597141,-92.3060276489616,3.80726988698278));
#22998=CARTESIAN_POINT('Ctrl Pts',(20.9283007496159,-92.002571568945,3.79157655282255));
#22999=CARTESIAN_POINT('Origin',(24.,-92.,12.2084234471775));
#23000=CARTESIAN_POINT('',(20.929838025779,-91.9979746552741,5.79157655282255));
#23001=CARTESIAN_POINT('',(20.9253102843548,-92.0026322735622,5.70842344717746));
#23002=CARTESIAN_POINT('',(20.9265,-91.9999999999999,12.2084234471775));
#23003=CARTESIAN_POINT('Ctrl Pts',(20.9253102843548,-92.0026322735622,5.70842344717746));
#23004=CARTESIAN_POINT('Ctrl Pts',(20.9326787378706,-91.1866490960334,5.66611956218844));
#23005=CARTESIAN_POINT('Ctrl Pts',(21.6842660273292,-89.3429095601005,5.57115462211654));
#23006=CARTESIAN_POINT('Ctrl Pts',(24.7888215932045,-88.4600276931838,5.42352862696176));
#23007=CARTESIAN_POINT('Ctrl Pts',(27.3956989960243,-90.726080156768,5.26554546171313));
#23008=CARTESIAN_POINT('Ctrl Pts',(26.9225615070512,-94.1476213996829,5.10756229646449));
#23009=CARTESIAN_POINT('Ctrl Pts',(23.7985609777147,-95.6211967303539,4.94957913121586));
#23010=CARTESIAN_POINT('Ctrl Pts',(21.3215407425041,-94.0960765086133,4.81653284812018));
#23011=CARTESIAN_POINT('Ctrl Pts',(20.9319623969258,-92.536970818142,4.73614762010738));
#23012=CARTESIAN_POINT('Ctrl Pts',(20.9312807091126,-91.9995675532498,4.70842344717746));
#23013=CARTESIAN_POINT('Ctrl Pts',(20.929838025779,-91.9979746552741,5.79157655282255));
#23014=CARTESIAN_POINT('Ctrl Pts',(20.9275818676586,-91.6293267200531,5.77253588131065));
#23015=CARTESIAN_POINT('Ctrl Pts',(21.1590710242286,-90.2438421434169,5.70083415471588));
#23016=CARTESIAN_POINT('Ctrl Pts',(23.2111785923562,-88.4600285259193,5.57647137303824));
#23017=CARTESIAN_POINT('Ctrl Pts',(26.53354332288,-89.404851549255,5.4184882077896));
#23018=CARTESIAN_POINT('Ctrl Pts',(27.5578977842682,-92.7035627953589,5.26050504254097));
#23019=CARTESIAN_POINT('Ctrl Pts',(25.3551175166524,-95.3641185720074,5.10252187729234));
#23020=CARTESIAN_POINT('Ctrl Pts',(21.959557040698,-94.9774442566837,4.94621238071952));
#23021=CARTESIAN_POINT('Ctrl Pts',(20.924193406317,-92.9798034901965,4.8425639392296));
#23022=CARTESIAN_POINT('Ctrl Pts',(20.9216167340284,-91.9994167252631,4.79157655282255));
#23023=CARTESIAN_POINT('Origin',(24.,-92.,12.2084234471775));
#23024=CARTESIAN_POINT('',(20.9285850678454,-92.0025047919022,6.79157655282255));
#23025=CARTESIAN_POINT('',(20.9234957058127,-91.9978813008157,6.70842344717746));
#23026=CARTESIAN_POINT('',(20.9265,-91.9999999999999,12.2084234471775));
#23027=CARTESIAN_POINT('Ctrl Pts',(20.9234957058127,-91.9978813008157,6.70842344717746));
#23028=CARTESIAN_POINT('Ctrl Pts',(20.9224297712393,-91.862878283601,6.70141361443525));
#23029=CARTESIAN_POINT('Ctrl Pts',(20.9915973803182,-90.7147700696949,6.64174272661017));
#23030=CARTESIAN_POINT('Ctrl Pts',(22.4354576201274,-88.7280203884636,6.52941078370221));
#23031=CARTESIAN_POINT('Ctrl Pts',(25.8851898408183,-88.9016612993893,6.37142761845357));
#23032=CARTESIAN_POINT('Ctrl Pts',(27.6249905303984,-91.885601165237,6.21344445320494));
#23033=CARTESIAN_POINT('Ctrl Pts',(26.0768010801705,-94.9733046786333,6.0554612879563));
#23034=CARTESIAN_POINT('Ctrl Pts',(22.6448821645724,-95.3641193633754,5.89747812270767));
#23035=CARTESIAN_POINT('Ctrl Pts',(21.031950207745,-93.4159924901843,5.78179884244805));
#23036=CARTESIAN_POINT('Ctrl Pts',(20.9235062815685,-92.2024076976298,5.71878061727132));
#23037=CARTESIAN_POINT('Ctrl Pts',(20.9253102843548,-92.0026322735622,5.70842344717746));
#23038=CARTESIAN_POINT('Ctrl Pts',(20.9285850678454,-92.0025047919022,6.79157655282255));
#23039=CARTESIAN_POINT('Ctrl Pts',(20.934071295281,-91.2983382673306,6.75516887847459));
#23040=CARTESIAN_POINT('Ctrl Pts',(21.5231707262624,-89.5673495506398,6.66610014904376));
#23041=CARTESIAN_POINT('Ctrl Pts',(24.3913282089151,-88.3943794585145,6.52437036453004));
#23042=CARTESIAN_POINT('Ctrl Pts',(27.2334540881776,-90.35731563858,6.3663871992814));
#23043=CARTESIAN_POINT('Ctrl Pts',(27.1427267432077,-93.8102226011646,6.20840403403277));
#23044=CARTESIAN_POINT('Ctrl Pts',(24.2014389748999,-95.6211958785123,6.05042086878413));
#23045=CARTESIAN_POINT('Ctrl Pts',(21.4539543223964,-94.3252211924294,5.9114783750474));
#23046=CARTESIAN_POINT('Ctrl Pts',(20.933821756151,-92.6489015397087,5.82519693639353));
#23047=CARTESIAN_POINT('Ctrl Pts',(20.929838025779,-91.9979746552741,5.79157655282255));
#23048=CARTESIAN_POINT('Origin',(24.,-92.,12.2084234471775));
#23049=CARTESIAN_POINT('',(20.9215398120818,-91.9996098254746,7.79157655282255));
#23050=CARTESIAN_POINT('',(20.9312256995769,-91.9993961639011,7.70842344717745));
#23051=CARTESIAN_POINT('',(20.9265,-91.9999999999999,12.2084234471775));
#23052=CARTESIAN_POINT('Ctrl Pts',(20.9312256995769,-91.9993961639011,7.70842344717745));
#23053=CARTESIAN_POINT('Ctrl Pts',(20.9303878819454,-91.5268985947141,7.68404661159918));
#23054=CARTESIAN_POINT('Ctrl Pts',(21.2544810105531,-90.0347579248865,7.60700872093804));
#23055=CARTESIAN_POINT('Ctrl Pts',(23.5706310054557,-88.3987105715367,7.47730977519401));
#23056=CARTESIAN_POINT('Ctrl Pts',(26.7813299086865,-89.6723730071853,7.31932660994538));
#23057=CARTESIAN_POINT('Ctrl Pts',(27.4692676579736,-93.0572726103796,7.16134344469675));
#23058=CARTESIAN_POINT('Ctrl Pts',(25.0104612250054,-95.483189850294,7.00336027944811));
#23059=CARTESIAN_POINT('Ctrl Pts',(21.7848978894954,-94.7822789631047,6.85238694694168));
#23060=CARTESIAN_POINT('Ctrl Pts',(20.9304375570666,-92.8770824147627,6.75407466951813));
#23061=CARTESIAN_POINT('Ctrl Pts',(20.9234957058127,-91.9978813008157,6.70842344717746));
#23062=CARTESIAN_POINT('Ctrl Pts',(20.9215398120818,-91.9996098254745,7.79157655282255));
#23063=CARTESIAN_POINT('Ctrl Pts',(20.9215012036849,-91.9781985065648,7.7904629307214));
#23064=CARTESIAN_POINT('Ctrl Pts',(20.9313646122183,-90.9443234457007,7.73668825353738));
#23065=CARTESIAN_POINT('Ctrl Pts',(22.0822083770023,-88.9217356813896,7.63025252127048));
#23066=CARTESIAN_POINT('Ctrl Pts',(25.5299143458989,-88.7116874252054,7.47226935602185));
#23067=CARTESIAN_POINT('Ctrl Pts',(27.5899360110292,-91.4842511522572,7.31428619077322));
#23068=CARTESIAN_POINT('Ctrl Pts',(26.3937630706594,-94.724616569919,7.15630302552458));
#23069=CARTESIAN_POINT('Ctrl Pts',(23.0263653754403,-95.4936618194068,6.99831986027594));
#23070=CARTESIAN_POINT('Ctrl Pts',(21.1145964666983,-93.6468831586791,6.87674436937527));
#23071=CARTESIAN_POINT('Ctrl Pts',(20.9261358659971,-92.3168639711034,6.80782993355747));
#23072=CARTESIAN_POINT('Ctrl Pts',(20.9285850678454,-92.0025047919022,6.79157655282255));
#23073=CARTESIAN_POINT('Origin',(24.,-92.,12.2084234471775));
#23074=CARTESIAN_POINT('',(20.9296146841086,-91.99786424691,8.79157655282255));
#23075=CARTESIAN_POINT('',(20.925632185667,-92.002679085539,8.70842344717746));
#23076=CARTESIAN_POINT('',(20.9265,-91.9999999999999,12.2084234471775));
#23077=CARTESIAN_POINT('Ctrl Pts',(20.925632185667,-92.002679085539,8.70842344717746));
#23078=CARTESIAN_POINT('Ctrl Pts',(20.9329424382584,-91.1972814204422,8.66667960876312));
#23079=CARTESIAN_POINT('Ctrl Pts',(21.6680869085146,-89.3640271254411,8.57227471526591));
#23080=CARTESIAN_POINT('Ctrl Pts',(24.7514084034007,-88.4518993616932,8.42520876668581));
#23081=CARTESIAN_POINT('Ctrl Pts',(27.3820616157699,-90.6903039066151,8.26722560143718));
#23082=CARTESIAN_POINT('Ctrl Pts',(26.9450699403022,-94.1166502818289,8.10924243618855));
#23083=CARTESIAN_POINT('Ctrl Pts',(23.8367990946118,-95.6231212490058,7.95125927093992));
#23084=CARTESIAN_POINT('Ctrl Pts',(21.3333230992967,-94.1179253063224,7.81765294126955));
#23085=CARTESIAN_POINT('Ctrl Pts',(20.9321978117167,-92.5476307745573,7.73670766668206));
#23086=CARTESIAN_POINT('Ctrl Pts',(20.9312256995769,-91.9993961639011,7.70842344717745));
#23087=CARTESIAN_POINT('Ctrl Pts',(20.9296146841086,-91.99786424691,8.79157655282255));
#23088=CARTESIAN_POINT('Ctrl Pts',(20.9272864716551,-91.6401225112664,8.77309592788534));
#23089=CARTESIAN_POINT('Ctrl Pts',(21.149833727977,-90.265786270585,8.70195424786525));
#23090=CARTESIAN_POINT('Ctrl Pts',(23.1738623478633,-88.4685627419331,8.57815151276229));
#23091=CARTESIAN_POINT('Ctrl Pts',(26.5060020988177,-89.3782461595948,8.42016834751365));
#23092=CARTESIAN_POINT('Ctrl Pts',(27.5651288739417,-92.6659672391889,8.26218518226502));
#23093=CARTESIAN_POINT('Ctrl Pts',(25.3905540118639,-95.3496247591348,8.10420201701639));
#23094=CARTESIAN_POINT('Ctrl Pts',(21.9789224334286,-94.9975617834283,7.94733247386889));
#23095=CARTESIAN_POINT('Ctrl Pts',(20.9233269207871,-92.9906987464103,7.84312398580428));
#23096=CARTESIAN_POINT('Ctrl Pts',(20.9215398120818,-91.9996098254745,7.79157655282255));
#23097=CARTESIAN_POINT('Origin',(24.,-92.,12.2084234471775));
#23098=CARTESIAN_POINT('',(20.9297109890477,-92.0031050978172,9.79157655282255));
#23099=CARTESIAN_POINT('',(20.9232328435277,-91.9980626432727,9.70842344717746));
#23100=CARTESIAN_POINT('',(20.9265,-91.9999999999999,12.2084234471775));
#23101=CARTESIAN_POINT('',(23.2062007174671,-94.9692229537457,10.));
#23102=CARTESIAN_POINT('Ctrl Pts',(23.2062007174671,-94.9692229537457,10.));
#23103=CARTESIAN_POINT('Ctrl Pts',(22.2237466982397,-94.7065713079336,9.94733894491712));
#23104=CARTESIAN_POINT('Ctrl Pts',(21.1240889563567,-93.6687841901452,9.87786446252464));
#23105=CARTESIAN_POINT('Ctrl Pts',(20.9273641407895,-92.3283664602092,9.80838998013216));
#23106=CARTESIAN_POINT('Ctrl Pts',(20.9297109890477,-92.0031050978172,9.79157655282255));
#23107=CARTESIAN_POINT('',(24.7956974280508,-94.9743010520069,10.));
#23108=CARTESIAN_POINT('Origin',(24.,-92.,10.));
#23109=CARTESIAN_POINT('Ctrl Pts',(24.7957018439802,-94.9743128659187,10.));
#23110=CARTESIAN_POINT('Ctrl Pts',(23.8480947973978,-95.2254055278759,9.94901908464117));
#23111=CARTESIAN_POINT('Ctrl Pts',(21.7874433743319,-94.7696547721756,9.85182690036699));
#23112=CARTESIAN_POINT('Ctrl Pts',(20.9299259678012,-92.8876740595769,9.75463471609281));
#23113=CARTESIAN_POINT('Ctrl Pts',(20.9232328435277,-91.9980626432727,9.70842344717746));
#23114=CARTESIAN_POINT('Origin',(-92.,24.,5.));
#23115=CARTESIAN_POINT('',(-94.5134952662832,24.0002743405048,1.38741669750802));
#23116=CARTESIAN_POINT('',(-94.515626303127,23.9964684456989,1.11258330249198));
#23117=CARTESIAN_POINT('',(-94.5175,24.,5.));
#23118=CARTESIAN_POINT('',(-93.913465996665,25.635987203375,0.999999999999999));
#23119=CARTESIAN_POINT('Ctrl Pts',(-94.515626303127,23.9964684456989,1.11258330249198));
#23120=CARTESIAN_POINT('Ctrl Pts',(-94.5104636015443,24.5890866576526,1.07505553499465));
#23121=CARTESIAN_POINT('Ctrl Pts',(-94.299221828084,25.1848035603044,1.03752776749732));
#23122=CARTESIAN_POINT('Ctrl Pts',(-93.913465996665,25.635987203375,0.999999999999995));
#23123=CARTESIAN_POINT('',(-94.5175,24.,1.));
#23124=CARTESIAN_POINT('Origin',(-92.,24.,1.));
#23125=CARTESIAN_POINT('',(-94.5175,24.,0.));
#23126=CARTESIAN_POINT('',(-94.5175,24.,5.));
#23127=CARTESIAN_POINT('Origin',(-92.,24.,0.));
#23128=CARTESIAN_POINT('',(-90.0828968401885,25.638534314987,1.));
#23129=CARTESIAN_POINT('Origin',(-92.,24.,1.));
#23130=CARTESIAN_POINT('Ctrl Pts',(-90.0828883826538,25.6385402378131,1.));
#23131=CARTESIAN_POINT('Ctrl Pts',(-90.6060431378804,26.2476960524168,1.05098091535882));
#23132=CARTESIAN_POINT('Ctrl Pts',(-91.4465813540296,26.5878274641506,1.10196183071765));
#23133=CARTESIAN_POINT('Ctrl Pts',(-92.2457357689255,26.5094850217743,1.15294274607647));
#23134=CARTESIAN_POINT('Ctrl Pts',(-93.0712273154455,26.4285607063854,1.20560380115935));
#23135=CARTESIAN_POINT('Ctrl Pts',(-93.8525624034825,25.9011253696412,1.25826485624222));
#23136=CARTESIAN_POINT('Ctrl Pts',(-94.2358878554464,25.1658537184213,1.3109259113251));
#23137=CARTESIAN_POINT('Ctrl Pts',(-94.4214827265106,24.8098568843833,1.33642284005274));
#23138=CARTESIAN_POINT('Ctrl Pts',(-94.5137757562955,24.4051388409379,1.36191976878038));
#23139=CARTESIAN_POINT('Ctrl Pts',(-94.5134952662832,24.0002743405048,1.38741669750802));
#23140=CARTESIAN_POINT('Origin',(-92.,24.,5.));
#23141=CARTESIAN_POINT('',(-94.5187354043534,23.9978903847199,2.38741669750802));
#23142=CARTESIAN_POINT('',(-94.5214125398479,24.0006455489044,2.11258330249198));
#23143=CARTESIAN_POINT('',(-94.5175,24.,5.));
#23144=CARTESIAN_POINT('Ctrl Pts',(-94.5214125398479,24.0006455489044,2.11258330249198));
#23145=CARTESIAN_POINT('Ctrl Pts',(-94.5215322047964,24.0358286169429,2.11034958724147));
#23146=CARTESIAN_POINT('Ctrl Pts',(-94.5208589221676,24.0710069479233,2.10811587199095));
#23147=CARTESIAN_POINT('Ctrl Pts',(-94.5193783712999,24.1061512068912,2.10588215674044));
#23148=CARTESIAN_POINT('Ctrl Pts',(-94.4844735772458,24.9346962763345,2.05322110165756));
#23149=CARTESIAN_POINT('Ctrl Pts',(-94.0008839809308,25.7443039053207,2.00056004657469));
#23150=CARTESIAN_POINT('Ctrl Pts',(-93.2879126402955,26.1678868628806,1.94789899149181));
#23151=CARTESIAN_POINT('Ctrl Pts',(-92.5749412996603,26.5914698204405,1.89523793640893));
#23152=CARTESIAN_POINT('Ctrl Pts',(-91.6325882147046,26.629028106574,1.84257688132605));
#23153=CARTESIAN_POINT('Ctrl Pts',(-90.8882532947046,26.2633575703982,1.78991582624317));
#23154=CARTESIAN_POINT('Ctrl Pts',(-90.1439183747045,25.8976870342223,1.73725477116029));
#23155=CARTESIAN_POINT('Ctrl Pts',(-89.59760161966,25.128787675737,1.68459371607741));
#23156=CARTESIAN_POINT('Ctrl Pts',(-89.4970124750772,24.3057173952046,1.63193266099454));
#23157=CARTESIAN_POINT('Ctrl Pts',(-89.3964233304945,23.4826471146723,1.57927160591166));
#23158=CARTESIAN_POINT('Ctrl Pts',(-89.7415617963736,22.6054059120929,1.52661055082878));
#23159=CARTESIAN_POINT('Ctrl Pts',(-90.3760121357463,22.0711233584703,1.4739494957459));
#23160=CARTESIAN_POINT('Ctrl Pts',(-91.010462475119,21.5368408048477,1.42128844066303));
#23161=CARTESIAN_POINT('Ctrl Pts',(-91.9342246879853,21.3455169001819,1.36862738558015));
#23162=CARTESIAN_POINT('Ctrl Pts',(-92.7281292572936,21.5853895325345,1.31596633049727));
#23163=CARTESIAN_POINT('Ctrl Pts',(-93.5220338266019,21.8252621648871,1.26330527541439));
#23164=CARTESIAN_POINT('Ctrl Pts',(-94.1860807523522,22.4963313342582,1.21064422033151));
#23165=CARTESIAN_POINT('Ctrl Pts',(-94.4192673158648,23.2907310848487,1.15798316524863));
#23166=CARTESIAN_POINT('Ctrl Pts',(-94.4862784936919,23.5190189507993,1.14284987766308));
#23167=CARTESIAN_POINT('Ctrl Pts',(-94.5177081921648,23.7574917511602,1.12771659007753));
#23168=CARTESIAN_POINT('Ctrl Pts',(-94.515626303127,23.9964684456989,1.11258330249198));
#23169=CARTESIAN_POINT('Ctrl Pts',(-94.5134952662832,24.0002743405048,1.38741669750802));
#23170=CARTESIAN_POINT('Ctrl Pts',(-94.5131964355411,23.5689364894249,1.41458082386326));
#23171=CARTESIAN_POINT('Ctrl Pts',(-94.4078218494689,23.1374324020536,1.4417449502185));
#23172=CARTESIAN_POINT('Ctrl Pts',(-94.1982522460689,22.7645021148375,1.46890907657374));
#23173=CARTESIAN_POINT('Ctrl Pts',(-93.7919753688369,22.041530128169,1.52157013165662));
#23174=CARTESIAN_POINT('Ctrl Pts',(-92.9941057984822,21.5386941205273,1.57423118673949));
#23175=CARTESIAN_POINT('Ctrl Pts',(-92.1666097792392,21.4839131073784,1.62689224182237));
#23176=CARTESIAN_POINT('Ctrl Pts',(-91.3391137599961,21.4291320942294,1.67955329690525));
#23177=CARTESIAN_POINT('Ctrl Pts',(-90.4819912918646,21.8224060755732,1.73221435198813));
#23178=CARTESIAN_POINT('Ctrl Pts',(-89.9839038787409,22.4854401372494,1.78487540707101));
#23179=CARTESIAN_POINT('Ctrl Pts',(-89.4858164656172,23.1484741989255,1.83753646215389));
#23180=CARTESIAN_POINT('Ctrl Pts',(-89.3467641075012,24.081268340934,1.89019751723676));
#23181=CARTESIAN_POINT('Ctrl Pts',(-89.6298379034513,24.8607543617003,1.94285857231964));
#23182=CARTESIAN_POINT('Ctrl Pts',(-89.9129116994015,25.6402403824667,1.99551962740252));
#23183=CARTESIAN_POINT('Ctrl Pts',(-90.6181116494178,26.2664182819909,2.0481806824854));
#23184=CARTESIAN_POINT('Ctrl Pts',(-91.4256035941691,26.4553204550754,2.10084173756828));
#23185=CARTESIAN_POINT('Ctrl Pts',(-92.2330955389203,26.64422262816,2.15350279265116));
#23186=CARTESIAN_POINT('Ctrl Pts',(-93.1428794784065,26.3958490748049,2.20616384773403));
#23187=CARTESIAN_POINT('Ctrl Pts',(-93.7423596992758,25.8228342131325,2.25882490281691));
#23188=CARTESIAN_POINT('Ctrl Pts',(-94.2303119273634,25.3564236982452,2.30168883438061));
#23189=CARTESIAN_POINT('Ctrl Pts',(-94.5126789427165,24.674928901641,2.34455276594432));
#23190=CARTESIAN_POINT('Ctrl Pts',(-94.5187354043534,23.9978903847199,2.38741669750802));
#23191=CARTESIAN_POINT('Origin',(-92.,24.,5.));
#23192=CARTESIAN_POINT('',(-94.5197283545653,24.0018289503525,3.38741669750802));
#23193=CARTESIAN_POINT('',(-94.5145913332515,24.0015585714996,3.11258330249198));
#23194=CARTESIAN_POINT('',(-94.5175,24.,5.));
#23195=CARTESIAN_POINT('Ctrl Pts',(-94.5145913332515,24.0015585714996,3.11258330249198));
#23196=CARTESIAN_POINT('Ctrl Pts',(-94.5163704675347,24.3124536217307,3.0929825844054));
#23197=CARTESIAN_POINT('Ctrl Pts',(-94.4629228052196,24.6227586740842,3.07338186631882));
#23198=CARTESIAN_POINT('Ctrl Pts',(-94.3514581912821,24.9105967308751,3.05378114823225));
#23199=CARTESIAN_POINT('Ctrl Pts',(-94.0519873173872,25.6839283862082,3.00112009314937));
#23200=CARTESIAN_POINT('Ctrl Pts',(-93.3337324697514,26.2950864454346,2.94845903806649));
#23201=CARTESIAN_POINT('Ctrl Pts',(-92.5224342992987,26.4669014516815,2.89579798298361));
#23202=CARTESIAN_POINT('Ctrl Pts',(-91.711136128846,26.6387164579284,2.84313692790074));
#23203=CARTESIAN_POINT('Ctrl Pts',(-90.8067946355765,26.3711884111957,2.79047587281786));
#23204=CARTESIAN_POINT('Ctrl Pts',(-90.2195444883874,25.7856434915614,2.73781481773498));
#23205=CARTESIAN_POINT('Ctrl Pts',(-89.6322943411984,25.200098571927,2.6851537626521));
#23206=CARTESIAN_POINT('Ctrl Pts',(-89.3621355400899,24.2965367793909,2.63249270756922));
#23207=CARTESIAN_POINT('Ctrl Pts',(-89.5315889600924,23.4847436160309,2.57983165248634));
#23208=CARTESIAN_POINT('Ctrl Pts',(-89.7010423800949,22.6729504526708,2.52717059740347));
#23209=CARTESIAN_POINT('Ctrl Pts',(-90.3101080212083,21.9529259184869,2.47450954232059));
#23210=CARTESIAN_POINT('Ctrl Pts',(-91.0825657562014,21.6512036069522,2.42184848723771));
#23211=CARTESIAN_POINT('Ctrl Pts',(-91.8550234911946,21.3494812954175,2.36918743215483));
#23212=CARTESIAN_POINT('Ctrl Pts',(-92.7908733200675,21.466061206532,2.31652637707195));
#23213=CARTESIAN_POINT('Ctrl Pts',(-93.4656882386074,21.9480924170396,2.26386532198907));
#23214=CARTESIAN_POINT('Ctrl Pts',(-94.1118796445259,22.4096773895362,2.21343798215671));
#23215=CARTESIAN_POINT('Ctrl Pts',(-94.5187110383817,23.2063686024949,2.16301064232434));
#23216=CARTESIAN_POINT('Ctrl Pts',(-94.5214125398479,24.0006455489044,2.11258330249198));
#23217=CARTESIAN_POINT('Ctrl Pts',(-94.5187354043534,23.9978903847199,2.38741669750802));
#23218=CARTESIAN_POINT('Ctrl Pts',(-94.5201196894756,23.8431441975285,2.3972138210272));
#23219=CARTESIAN_POINT('Ctrl Pts',(-94.5070691791327,23.6886308117444,2.40701094454637));
#23220=CARTESIAN_POINT('Ctrl Pts',(-94.4787393827788,23.5369716347155,2.41680806806555));
#23221=CARTESIAN_POINT('Ctrl Pts',(-94.3264623431602,22.7217800879606,2.46946912314842));
#23222=CARTESIAN_POINT('Ctrl Pts',(-93.7327317616706,21.9890531644405,2.5221301782313));
#23223=CARTESIAN_POINT('Ctrl Pts',(-92.9668162273558,21.6710932957471,2.57479123331418));
#23224=CARTESIAN_POINT('Ctrl Pts',(-92.2009006930409,21.3531334270537,2.62745228839706));
#23225=CARTESIAN_POINT('Ctrl Pts',(-91.2628002059009,21.449940613187,2.68011334347994));
#23226=CARTESIAN_POINT('Ctrl Pts',(-90.5779585445906,21.9176119917392,2.73277439856282));
#23227=CARTESIAN_POINT('Ctrl Pts',(-89.8931168832802,22.3852833702914,2.78543545364569));
#23228=CARTESIAN_POINT('Ctrl Pts',(-89.4615340477996,23.2238189412625,2.83809650872857));
#23229=CARTESIAN_POINT('Ctrl Pts',(-89.4789406121676,24.0529280971511,2.89075756381145));
#23230=CARTESIAN_POINT('Ctrl Pts',(-89.4963471765355,24.8820372530396,2.94341861889433));
#23231=CARTESIAN_POINT('Ctrl Pts',(-89.9627431407521,25.7017199938457,2.99607967397721));
#23232=CARTESIAN_POINT('Ctrl Pts',(-90.6666097831963,26.1402364113417,3.04874072906009));
#23233=CARTESIAN_POINT('Ctrl Pts',(-91.3704764256404,26.5787528288377,3.10140178414296));
#23234=CARTESIAN_POINT('Ctrl Pts',(-92.3118137463122,26.6361029230235,3.15406283922584));
#23235=CARTESIAN_POINT('Ctrl Pts',(-93.063709299524,26.2862773477979,3.20672389430872));
#23236=CARTESIAN_POINT('Ctrl Pts',(-93.8156048527357,25.9364517725724,3.2593849493916));
#23237=CARTESIAN_POINT('Ctrl Pts',(-94.3780586384875,25.1794505279353,3.31204600447447));
#23238=CARTESIAN_POINT('Ctrl Pts',(-94.4959882199517,24.358586646163,3.36470705955735));
#23239=CARTESIAN_POINT('Ctrl Pts',(-94.5129402673076,24.2405897600233,3.37227693887424));
#23240=CARTESIAN_POINT('Ctrl Pts',(-94.5207069963199,24.1212732637326,3.37984681819113));
#23241=CARTESIAN_POINT('Ctrl Pts',(-94.5197283545653,24.0018289503525,3.38741669750802));
#23242=CARTESIAN_POINT('Origin',(-92.,24.,5.));
#23243=CARTESIAN_POINT('',(-94.5135838218621,24.000354216548,4.38741669750802));
#23244=CARTESIAN_POINT('',(-94.5160253566384,23.9978936308049,4.11258330249198));
#23245=CARTESIAN_POINT('',(-94.5175,24.,5.));
#23246=CARTESIAN_POINT('Ctrl Pts',(-94.5160253566384,23.9978936308049,4.11258330249198));
#23247=CARTESIAN_POINT('Ctrl Pts',(-94.5113087243027,24.5834107803607,4.07561558156934));
#23248=CARTESIAN_POINT('Ctrl Pts',(-94.3074058729855,25.1718905111793,4.03864786064669));
#23249=CARTESIAN_POINT('Ctrl Pts',(-93.9337852402154,25.6183375776454,4.00168013972405));
#23250=CARTESIAN_POINT('Ctrl Pts',(-93.4015572253053,26.2543079045141,3.94901908464117));
#23251=CARTESIAN_POINT('Ctrl Pts',(-92.5249308268757,26.6020596393699,3.8963580295583));
#23252=CARTESIAN_POINT('Ctrl Pts',(-91.7014710746985,26.5038814515943,3.84369697447542));
#23253=CARTESIAN_POINT('Ctrl Pts',(-90.8780113225213,26.4057032638187,3.79103591939254));
#23254=CARTESIAN_POINT('Ctrl Pts',(-90.1077182165965,25.8615951534119,3.73837486430966));
#23255=CARTESIAN_POINT('Ctrl Pts',(-89.7399328314132,25.1183194017708,3.68571380922678));
#23256=CARTESIAN_POINT('Ctrl Pts',(-89.3721474462299,24.3750436501297,3.6330527541439));
#23257=CARTESIAN_POINT('Ctrl Pts',(-89.4068697817883,23.4326002572544,3.58039169906103));
#23258=CARTESIAN_POINT('Ctrl Pts',(-89.8283526559748,22.7184034519114,3.52773064397815));
#23259=CARTESIAN_POINT('Ctrl Pts',(-90.2498355301613,22.0042066465685,3.47506958889527));
#23260=CARTESIAN_POINT('Ctrl Pts',(-91.058078942976,21.518256428758,3.42240853381239));
#23261=CARTESIAN_POINT('Ctrl Pts',(-91.8865307343323,21.4809393801385,3.36974747872952));
#23262=CARTESIAN_POINT('Ctrl Pts',(-92.7149825256887,21.4436223315191,3.31708642364664));
#23263=CARTESIAN_POINT('Ctrl Pts',(-93.5636426955868,21.8549384520908,3.26442536856376));
#23264=CARTESIAN_POINT('Ctrl Pts',(-94.0476293304588,22.5283491380965,3.21176431348088));
#23265=CARTESIAN_POINT('Ctrl Pts',(-94.3514736272621,22.951112870825,3.17870397648458));
#23266=CARTESIAN_POINT('Ctrl Pts',(-94.5115904850835,23.4771749705661,3.14564363948828));
#23267=CARTESIAN_POINT('Ctrl Pts',(-94.5145913332515,24.0015585714996,3.11258330249198));
#23268=CARTESIAN_POINT('Ctrl Pts',(-94.5197283545653,24.0018289503525,3.38741669750802));
#23269=CARTESIAN_POINT('Ctrl Pts',(-94.5138989211591,23.2903401268977,3.43250787327401));
#23270=CARTESIAN_POINT('Ctrl Pts',(-94.1977683024704,22.5743161275881,3.47759904904));
#23271=CARTESIAN_POINT('Ctrl Pts',(-93.6643206092001,22.105645640677,3.52269022480599));
#23272=CARTESIAN_POINT('Ctrl Pts',(-93.0413180398075,21.5582950358707,3.57535127988887));
#23273=CARTESIAN_POINT('Ctrl Pts',(-92.1219075238456,21.3483203451655,3.62801233497174));
#23274=CARTESIAN_POINT('Ctrl Pts',(-91.3230574099717,21.5709486859402,3.68067339005462));
#23275=CARTESIAN_POINT('Ctrl Pts',(-90.5242072960977,21.7935770267148,3.7333344451375));
#23276=CARTESIAN_POINT('Ctrl Pts',(-89.8459175843116,22.4488083989694,3.78599550022038));
#23277=CARTESIAN_POINT('Ctrl Pts',(-89.5958042400641,23.239484187431,3.83865655530326));
#23278=CARTESIAN_POINT('Ctrl Pts',(-89.3456908958165,24.0301599758926,3.89131761038613));
#23279=CARTESIAN_POINT('Ctrl Pts',(-89.5237539191075,24.9562801805613,3.94397866546901));
#23280=CARTESIAN_POINT('Ctrl Pts',(-90.0492386873867,25.5978334861916,3.99663972055189));
#23281=CARTESIAN_POINT('Ctrl Pts',(-90.5747234556659,26.2393867918219,4.04930077563477));
#23282=CARTESIAN_POINT('Ctrl Pts',(-91.4476299689333,26.5963731984139,4.10196183071765));
#23283=CARTESIAN_POINT('Ctrl Pts',(-92.2720802276353,26.5068932768485,4.15462288580053));
#23284=CARTESIAN_POINT('Ctrl Pts',(-93.0965304863372,26.417413355283,4.2072839408834));
#23285=CARTESIAN_POINT('Ctrl Pts',(-93.8725244904738,25.8814671055602,4.25994499596628));
#23286=CARTESIAN_POINT('Ctrl Pts',(-94.2481357153638,25.1421152990992,4.31260605104916));
#23287=CARTESIAN_POINT('Ctrl Pts',(-94.4260009866856,24.7920059281746,4.33754293320211));
#23288=CARTESIAN_POINT('Ctrl Pts',(-94.5140860549172,24.396285723967,4.36247981535507));
#23289=CARTESIAN_POINT('Ctrl Pts',(-94.5135838218621,24.000354216548,4.38741669750802));
#23290=CARTESIAN_POINT('Origin',(-92.,24.,5.));
#23291=CARTESIAN_POINT('',(-94.5184741887081,23.9978439082845,5.38741669750803));
#23292=CARTESIAN_POINT('',(-94.5215002261916,24.0004777596726,5.11258330249198));
#23293=CARTESIAN_POINT('',(-94.5175,24.,5.));
#23294=CARTESIAN_POINT('Ctrl Pts',(-94.5215002261916,24.0004777596726,5.11258330249198));
#23295=CARTESIAN_POINT('Ctrl Pts',(-94.521569505293,24.0268374618337,5.11090963381616));
#23296=CARTESIAN_POINT('Ctrl Pts',(-94.5211915450548,24.0531951295678,5.10923596514032));
#23297=CARTESIAN_POINT('Ctrl Pts',(-94.5203601912645,24.0795384889352,5.1075622964645));
#23298=CARTESIAN_POINT('Ctrl Pts',(-94.494202106107,24.9084176564483,5.05490124138162));
#23299=CARTESIAN_POINT('Ctrl Pts',(-94.0191792969125,25.723131379711,5.00224018629874));
#23300=CARTESIAN_POINT('Ctrl Pts',(-93.3107227144406,26.1541930811531,4.94957913121586));
#23301=CARTESIAN_POINT('Ctrl Pts',(-92.6022661319687,26.5852547825952,4.89691807613298));
#23302=CARTESIAN_POINT('Ctrl Pts',(-91.6603757762195,26.6326644622167,4.84425702105011));
#23303=CARTESIAN_POINT('Ctrl Pts',(-90.9122149978595,26.2749210214316,4.79159596596723));
#23304=CARTESIAN_POINT('Ctrl Pts',(-90.1640542194994,25.9171775806464,4.73893491088435));
#23305=CARTESIAN_POINT('Ctrl Pts',(-89.6096230185287,25.1542810194546,4.68627385580147));
#23306=CARTESIAN_POINT('Ctrl Pts',(-89.50036540662,24.3322179475565,4.63361280071859));
#23307=CARTESIAN_POINT('Ctrl Pts',(-89.3911077947114,23.5101548756584,4.58095174563571));
#23308=CARTESIAN_POINT('Ctrl Pts',(-89.7270237718648,22.6289252930542,4.52829069055284));
#23309=CARTESIAN_POINT('Ctrl Pts',(-90.3557697095322,22.0881818554959,4.47562963546996));
#23310=CARTESIAN_POINT('Ctrl Pts',(-90.9845156471996,21.5474384179377,4.42296858038708));
#23311=CARTESIAN_POINT('Ctrl Pts',(-91.9060915453809,21.3471811254255,4.3703075253042));
#23312=CARTESIAN_POINT('Ctrl Pts',(-92.7025470068623,21.5782300758527,4.31764647022132));
#23313=CARTESIAN_POINT('Ctrl Pts',(-93.4990024683437,21.80927902628,4.26498541513844));
#23314=CARTESIAN_POINT('Ctrl Pts',(-94.1703374931251,22.4716342196466,4.21232436005557));
#23315=CARTESIAN_POINT('Ctrl Pts',(-94.4120901898205,23.2649062757708,4.15966330497269));
#23316=CARTESIAN_POINT('Ctrl Pts',(-94.4841340531159,23.5013064663318,4.14396997081245));
#23317=CARTESIAN_POINT('Ctrl Pts',(-94.5180276355322,23.7493331013702,4.12827663665222));
#23318=CARTESIAN_POINT('Ctrl Pts',(-94.5160253566384,23.9978936308049,4.11258330249198));
#23319=CARTESIAN_POINT('Ctrl Pts',(-94.5135838218621,24.000354216548,4.38741669750802));
#23320=CARTESIAN_POINT('Ctrl Pts',(-94.5130254522959,23.5601679289135,4.41514087043795));
#23321=CARTESIAN_POINT('Ctrl Pts',(-94.4029695423041,23.1197204618369,4.44286504336787));
#23322=CARTESIAN_POINT('Ctrl Pts',(-94.1850553752593,22.7413997625482,4.47058921629779));
#23323=CARTESIAN_POINT('Ctrl Pts',(-93.7711353646214,22.0227933956572,4.52325027138067));
#23324=CARTESIAN_POINT('Ctrl Pts',(-92.968066897702,21.5283380250743,4.57591132646355));
#23325=CARTESIAN_POINT('Ctrl Pts',(-92.1400552293209,21.4822775999311,4.62857238154643));
#23326=CARTESIAN_POINT('Ctrl Pts',(-91.3120435609398,21.4362171747878,4.6812334366293));
#23327=CARTESIAN_POINT('Ctrl Pts',(-90.4590886910969,21.8385516950844,4.73389449171218));
#23328=CARTESIAN_POINT('Ctrl Pts',(-89.9680202099297,22.506815589517,4.78655554679506));
#23329=CARTESIAN_POINT('Ctrl Pts',(-89.4769517287624,23.1750794839497,4.83921660187794));
#23330=CARTESIAN_POINT('Ctrl Pts',(-89.3477696362708,24.1092727525185,4.89187765696082));
#23331=CARTESIAN_POINT('Ctrl Pts',(-89.6390602159942,24.8857228049574,4.9445387120437));
#23332=CARTESIAN_POINT('Ctrl Pts',(-89.9303507957177,25.6621728573963,4.99719976712658));
#23333=CARTESIAN_POINT('Ctrl Pts',(-90.6421140476561,26.2808796937054,5.04986082220945));
#23334=CARTESIAN_POINT('Ctrl Pts',(-91.4515531900703,26.4612492047028,5.10252187729233));
#23335=CARTESIAN_POINT('Ctrl Pts',(-92.2609923324846,26.6416187157001,5.15518293237521));
#23336=CARTESIAN_POINT('Ctrl Pts',(-93.1681073653747,26.3836509013857,5.20784398745809));
#23337=CARTESIAN_POINT('Ctrl Pts',(-93.7615061404264,25.8043385680607,5.26050504254097));
#23338=CARTESIAN_POINT('Ctrl Pts',(-94.2381975681409,25.3389631158763,5.30280892752999));
#23339=CARTESIAN_POINT('Ctrl Pts',(-94.5124386983965,24.6662146256838,5.34511281251901));
#23340=CARTESIAN_POINT('Ctrl Pts',(-94.5184741887081,23.9978439082845,5.38741669750803));
#23341=CARTESIAN_POINT('Origin',(-92.,24.,5.));
#23342=CARTESIAN_POINT('',(-94.5199605075385,24.0017354236374,6.38741669750802));
#23343=CARTESIAN_POINT('',(-94.5147661754846,24.0016589575576,6.11258330249198));
#23344=CARTESIAN_POINT('',(-94.5175,24.,5.));
#23345=CARTESIAN_POINT('Ctrl Pts',(-94.5147661754846,24.0016589575576,6.11258330249198));
#23346=CARTESIAN_POINT('Ctrl Pts',(-94.5166141920307,24.3036180613248,6.09354263098009));
#23347=CARTESIAN_POINT('Ctrl Pts',(-94.4662618562805,24.604981570585,6.07450195946819));
#23348=CARTESIAN_POINT('Ctrl Pts',(-94.3609398422945,24.8857228268249,6.0554612879563));
#23349=CARTESIAN_POINT('Ctrl Pts',(-94.0696492553794,25.6621728984334,6.00280023287342));
#23350=CARTESIAN_POINT('Ctrl Pts',(-93.3578859858684,26.2808797500176,5.95013917779055));
#23351=CARTESIAN_POINT('Ctrl Pts',(-92.5484468234701,26.4612492654681,5.89747812270767));
#23352=CARTESIAN_POINT('Ctrl Pts',(-91.7390076610717,26.6416187809185,5.84481706762479));
#23353=CARTESIAN_POINT('Ctrl Pts',(-90.8318926057861,26.3836509602352,5.79215601254191));
#23354=CARTESIAN_POINT('Ctrl Pts',(-90.2384938160841,25.8043386126076,5.73949495745903));
#23355=CARTESIAN_POINT('Ctrl Pts',(-89.6450950263822,25.2250262649801,5.68683390237615));
#23356=CARTESIAN_POINT('Ctrl Pts',(-89.3654125022639,24.3243693904083,5.63417284729328));
#23357=CARTESIAN_POINT('Ctrl Pts',(-89.5262870414957,23.5108312521748,5.5815117922104));
#23358=CARTESIAN_POINT('Ctrl Pts',(-89.6871615807275,22.6972931139413,5.52885073712752));
#23359=CARTESIAN_POINT('Ctrl Pts',(-90.2885931833094,21.9708737120461,5.47618968204464));
#23360=CARTESIAN_POINT('Ctrl Pts',(-91.0578223533957,21.6610166423891,5.42352862696177));
#23361=CARTESIAN_POINT('Ctrl Pts',(-91.8270515234819,21.3511595727322,5.37086757187889));
#23362=CARTESIAN_POINT('Ctrl Pts',(-92.7640782610725,21.4578648353135,5.31820651679601));
#23363=CARTESIAN_POINT('Ctrl Pts',(-93.4439449493075,21.932739772486,5.26554546171313));
#23364=CARTESIAN_POINT('Ctrl Pts',(-94.1022041787089,22.392522279284,5.21455807530608));
#23365=CARTESIAN_POINT('Ctrl Pts',(-94.5193896768554,23.1974440773951,5.16357068889903));
#23366=CARTESIAN_POINT('Ctrl Pts',(-94.5215002261916,24.0004777596726,5.11258330249198));
#23367=CARTESIAN_POINT('Ctrl Pts',(-94.5184741887081,23.9978439082845,5.38741669750803));
#23368=CARTESIAN_POINT('Ctrl Pts',(-94.5199518449512,23.8342081285527,5.39777386760188));
#23369=CARTESIAN_POINT('Ctrl Pts',(-94.5053530710441,23.6708347555271,5.40813103769574));
#23370=CARTESIAN_POINT('Ctrl Pts',(-94.4737128974312,23.5108312642518,5.4184882077896));
#23371=CARTESIAN_POINT('Ctrl Pts',(-94.3128383621712,22.6972931461036,5.47114926287248));
#23372=CARTESIAN_POINT('Ctrl Pts',(-93.7114067744379,21.9708737621428,5.52381031795536));
#23373=CARTESIAN_POINT('Ctrl Pts',(-92.9421776233431,21.6610167001358,5.57647137303824));
#23374=CARTESIAN_POINT('Ctrl Pts',(-92.1729484722482,21.3511596381289,5.62913242812112));
#23375=CARTESIAN_POINT('Ctrl Pts',(-91.2359217577917,21.4578648980758,5.68179348320399));
#23376=CARTESIAN_POINT('Ctrl Pts',(-90.5560550863417,21.9327398235241,5.73445453828687));
#23377=CARTESIAN_POINT('Ctrl Pts',(-89.8761884148917,22.4076147489725,5.78711559336975));
#23378=CARTESIAN_POINT('Ctrl Pts',(-89.4534817864484,23.2506593399223,5.83977664845262));
#23379=CARTESIAN_POINT('Ctrl Pts',(-89.4796398709601,24.0795384869714,5.8924377035355));
#23380=CARTESIAN_POINT('Ctrl Pts',(-89.5057979554718,24.9084176340206,5.94509875861838));
#23381=CARTESIAN_POINT('Ctrl Pts',(-89.9808207529386,25.723131337169,5.99775981370126));
#23382=CARTESIAN_POINT('Ctrl Pts',(-90.6892773179196,26.1541930279687,6.05042086878414));
#23383=CARTESIAN_POINT('Ctrl Pts',(-91.3977338829005,26.5852547187684,6.10308192386702));
#23384=CARTESIAN_POINT('Ctrl Pts',(-92.3396242153956,26.6326643972193,6.15574297894989));
#23385=CARTESIAN_POINT('Ctrl Pts',(-93.0877849752844,26.2749209652664,6.20840403403277));
#23386=CARTESIAN_POINT('Ctrl Pts',(-93.8359457351732,25.9171775333136,6.26106508911565));
#23387=CARTESIAN_POINT('Ctrl Pts',(-94.3903769224557,25.154280990957,6.31372614419853));
#23388=CARTESIAN_POINT('Ctrl Pts',(-94.499634531667,24.3322179393546,6.36638719928141));
#23389=CARTESIAN_POINT('Ctrl Pts',(-94.5141780603748,24.2227912579823,6.37339703202361));
#23390=CARTESIAN_POINT('Ctrl Pts',(-94.5208336131063,24.1123162124966,6.38040686476582));
#23391=CARTESIAN_POINT('Ctrl Pts',(-94.5199605075385,24.0017354236374,6.38741669750802));
#23392=CARTESIAN_POINT('Origin',(-92.,24.,5.));
#23393=CARTESIAN_POINT('',(-94.5136288801011,24.0004946012931,7.38741669750802));
#23394=CARTESIAN_POINT('',(-94.5157924718976,23.9979483278017,7.11258330249199));
#23395=CARTESIAN_POINT('',(-94.5175,24.,5.));
#23396=CARTESIAN_POINT('Ctrl Pts',(-94.5157924718976,23.9979483278017,7.11258330249199));
#23397=CARTESIAN_POINT('Ctrl Pts',(-94.511298709256,24.5747303258767,7.07617562814403));
#23398=CARTESIAN_POINT('Ctrl Pts',(-94.3140597937548,25.1542901069194,7.03976795379607));
#23399=CARTESIAN_POINT('Ctrl Pts',(-93.9507613607754,25.5978335256406,7.00336027944811));
#23400=CARTESIAN_POINT('Ctrl Pts',(-93.4252765795229,26.2393868471104,6.95069922436523));
#23401=CARTESIAN_POINT('Ctrl Pts',(-92.552370044704,26.5963732625152,6.89803816928236));
#23402=CARTESIAN_POINT('Ctrl Pts',(-91.7279197656473,26.5068933387405,6.84537711419948));
#23403=CARTESIAN_POINT('Ctrl Pts',(-90.9034694865905,26.4174134149657,6.7927160591166));
#23404=CARTESIAN_POINT('Ctrl Pts',(-90.1274754632958,25.8814671520113,6.74005500403372));
#23405=CARTESIAN_POINT('Ctrl Pts',(-89.7518642291325,25.1421153272968,6.68739394895084));
#23406=CARTESIAN_POINT('Ctrl Pts',(-89.3762529949691,24.4027635025822,6.63473289386796));
#23407=CARTESIAN_POINT('Ctrl Pts',(-89.4010245499371,23.4600061161074,6.58207183878508));
#23408=CARTESIAN_POINT('Ctrl Pts',(-89.8149445707942,22.7413997314749,6.52941078370221));
#23409=CARTESIAN_POINT('Ctrl Pts',(-90.2288645916513,22.0227933468423,6.47674972861933));
#23410=CARTESIAN_POINT('Ctrl Pts',(-91.0319330783976,21.5283379640519,6.42408867353645));
#23411=CARTESIAN_POINT('Ctrl Pts',(-91.8599447672213,21.4822775377715,6.37142761845357));
#23412=CARTESIAN_POINT('Ctrl Pts',(-92.6879564560451,21.4362171114912,6.31876656337069));
#23413=CARTESIAN_POINT('Ctrl Pts',(-93.5409113469464,21.8385516417208,6.26610550828782));
#23414=CARTESIAN_POINT('Ctrl Pts',(-94.0319798402375,22.5068155526521,6.21344445320494));
#23415=CARTESIAN_POINT('Ctrl Pts',(-94.3454925694847,22.9334551058627,6.17982406963395));
#23416=CARTESIAN_POINT('Ctrl Pts',(-94.5115031064752,23.4684854880682,6.14620368606297));
#23417=CARTESIAN_POINT('Ctrl Pts',(-94.5147661754846,24.0016589575576,6.11258330249198));
#23418=CARTESIAN_POINT('Ctrl Pts',(-94.5199605075385,24.0017354236374,6.38741669750802));
#23419=CARTESIAN_POINT('Ctrl Pts',(-94.5142744465628,23.2815829799959,6.4330679198487));
#23420=CARTESIAN_POINT('Ctrl Pts',(-94.1892823731636,22.556945740582,6.47871914218937));
#23421=CARTESIAN_POINT('Ctrl Pts',(-93.6442302498737,22.0881819026962,6.52437036453004));
#23422=CARTESIAN_POINT('Ctrl Pts',(-93.0154843277293,21.5474384784885,6.57703141961292));
#23423=CARTESIAN_POINT('Ctrl Pts',(-92.0939084523006,21.3471811909213,6.6296924746958));
#23424=CARTESIAN_POINT('Ctrl Pts',(-91.2974530104828,21.5782301356438,6.68235352977868));
#23425=CARTESIAN_POINT('Ctrl Pts',(-90.500997568665,21.8092790803663,6.73501458486156));
#23426=CARTESIAN_POINT('Ctrl Pts',(-89.829662560458,22.4716342573785,6.78767563994443));
#23427=CARTESIAN_POINT('Ctrl Pts',(-89.5879098697311,23.2649062939185,6.84033669502731));
#23428=CARTESIAN_POINT('Ctrl Pts',(-89.3461571790042,24.0581783304585,6.89299775011019));
#23429=CARTESIAN_POINT('Ctrl Pts',(-89.5339868057573,24.9823672265264,6.94565880519307));
#23430=CARTESIAN_POINT('Ctrl Pts',(-90.0662148075274,25.6183375376923,6.99831986027595));
#23431=CARTESIAN_POINT('Ctrl Pts',(-90.5984428092974,26.2543078488581,7.05098091535882));
#23432=CARTESIAN_POINT('Ctrl Pts',(-91.4750691860844,26.602059575122,7.1036419704417));
#23433=CARTESIAN_POINT('Ctrl Pts',(-92.2985289179312,26.5038813897733,7.15630302552458));
#23434=CARTESIAN_POINT('Ctrl Pts',(-93.121988649778,26.4057032044245,7.20896408060746));
#23435=CARTESIAN_POINT('Ctrl Pts',(-93.8922817366847,25.8615951074633,7.26162513569034));
#23436=CARTESIAN_POINT('Ctrl Pts',(-94.2600671127882,25.1183193741671,7.31428619077321));
#23437=CARTESIAN_POINT('Ctrl Pts',(-94.4303151951188,24.774256568905,7.33866302635148));
#23438=CARTESIAN_POINT('Ctrl Pts',(-94.5143151353889,24.3875167213616,7.36303986192975));
#23439=CARTESIAN_POINT('Ctrl Pts',(-94.5136288801011,24.0004946012931,7.38741669750802));
#23440=CARTESIAN_POINT('Origin',(-92.,24.,5.));
#23441=CARTESIAN_POINT('',(-94.5182105203766,23.9978055611691,8.38741669750802));
#23442=CARTESIAN_POINT('',(-94.5215632327497,24.0003195913041,8.11258330249198));
#23443=CARTESIAN_POINT('',(-94.5175,24.,5.));
#23444=CARTESIAN_POINT('Ctrl Pts',(-94.5215632327497,24.0003195913041,8.11258330249198));
#23445=CARTESIAN_POINT('Ctrl Pts',(-94.5215948568411,24.0178575782261,8.11146968039084));
#23446=CARTESIAN_POINT('Ctrl Pts',(-94.521427546271,24.0353949460436,8.11035605828969));
#23447=CARTESIAN_POINT('Ctrl Pts',(-94.5210594500516,24.0529280984189,8.10924243618855));
#23448=CARTESIAN_POINT('Ctrl Pts',(-94.5036528852352,24.8820372747418,8.05658138110567));
#23449=CARTESIAN_POINT('Ctrl Pts',(-94.0372569095472,25.7017200358608,8.0039203260228));
#23450=CARTESIAN_POINT('Ctrl Pts',(-93.3333902497356,26.1402364642016,7.95125927093992));
#23451=CARTESIAN_POINT('Ctrl Pts',(-92.6295235899239,26.5787528925424,7.89859821585704));
#23452=CARTESIAN_POINT('Ctrl Pts',(-91.6881862459885,26.636102988105,7.84593716077416));
#23453=CARTESIAN_POINT('Ctrl Pts',(-90.9362906742079,26.2862774042331,7.79327610569128));
#23454=CARTESIAN_POINT('Ctrl Pts',(-90.1843951024273,25.9364518203612,7.7406150506084));
#23455=CARTESIAN_POINT('Ctrl Pts',(-89.6219413028015,25.1794505570548,7.68795399552552));
#23456=CARTESIAN_POINT('Ctrl Pts',(-89.5040117184286,24.3585866550213,7.63529294044265));
#23457=CARTESIAN_POINT('Ctrl Pts',(-89.3860821340558,23.5377227529879,7.58263188535977));
#23458=CARTESIAN_POINT('Ctrl Pts',(-89.7126767649358,22.6529962122272,7.52997083027689));
#23459=CARTESIAN_POINT('Ctrl Pts',(-90.3356793497081,22.105645593905,7.47730977519401));
#23460=CARTESIAN_POINT('Ctrl Pts',(-90.9586819344803,21.5582949755827,7.42464872011113));
#23461=CARTESIAN_POINT('Ctrl Pts',(-91.8780924731448,21.3483202796988,7.37198766502825));
#23462=CARTESIAN_POINT('Ctrl Pts',(-92.6769426067422,21.5709486259712,7.31932660994538));
#23463=CARTESIAN_POINT('Ctrl Pts',(-93.4757927403396,21.7935769722436,7.2666655548625));
#23464=CARTESIAN_POINT('Ctrl Pts',(-94.15408246887,22.4488083606723,7.21400449977962));
#23465=CARTESIAN_POINT('Ctrl Pts',(-94.4041958192921,23.2394841686541,7.16134344469675));
#23466=CARTESIAN_POINT('Ctrl Pts',(-94.4813911490268,23.4835194414908,7.14509006396183));
#23467=CARTESIAN_POINT('Ctrl Pts',(-94.517798610341,23.7404570822428,7.12883668322691));
#23468=CARTESIAN_POINT('Ctrl Pts',(-94.5157924718976,23.9979483278017,7.11258330249199));
#23469=CARTESIAN_POINT('Ctrl Pts',(-94.5136288801011,24.0004946012931,7.38741669750802));
#23470=CARTESIAN_POINT('Ctrl Pts',(-94.5128326243634,23.5514363729595,7.41570091701263));
#23471=CARTESIAN_POINT('Ctrl Pts',(-94.3980254709817,23.1019981282164,7.44398513651724));
#23472=CARTESIAN_POINT('Ctrl Pts',(-94.1716472904104,22.7184034835405,7.47226935602185));
#23473=CARTESIAN_POINT('Ctrl Pts',(-93.7501644266289,22.0042066958411,7.52493041110473));
#23474=CARTESIAN_POINT('Ctrl Pts',(-92.9419210337657,21.5182564900734,7.57759146618761));
#23475=CARTESIAN_POINT('Ctrl Pts',(-92.1134692628649,21.4809394423544,7.63025252127049));
#23476=CARTESIAN_POINT('Ctrl Pts',(-91.285017491964,21.4436223946354,7.68291357635336));
#23477=CARTESIAN_POINT('Ctrl Pts',(-90.4363573430256,21.8549385049651,7.73557463143624));
#23478=CARTESIAN_POINT('Ctrl Pts',(-89.9523707200979,22.5283491743849,7.78823568651912));
#23479=CARTESIAN_POINT('Ctrl Pts',(-89.4683840971702,23.2017598438046,7.84089674160199));
#23480=CARTESIAN_POINT('Ctrl Pts',(-89.3490710002533,24.1372650723145,7.89355779668487));
#23481=CARTESIAN_POINT('Ctrl Pts',(-89.648541866765,24.9105967084797,7.94621885176775));
#23482=CARTESIAN_POINT('Ctrl Pts',(-89.9480127332768,25.6839283446448,7.99887990685063));
#23483=CARTESIAN_POINT('Ctrl Pts',(-90.6662675632173,26.2950863884653,8.05154096193351));
#23484=CARTESIAN_POINT('Ctrl Pts',(-91.4775657136168,26.4669013906121,8.10420201701639));
#23485=CARTESIAN_POINT('Ctrl Pts',(-92.2888638640162,26.6387163927589,8.15686307209926));
#23486=CARTESIAN_POINT('Ctrl Pts',(-93.1932053348746,26.3711883532321,8.20952412718214));
#23487=CARTESIAN_POINT('Ctrl Pts',(-93.7804554676164,25.785643447789,8.26218518226502));
#23488=CARTESIAN_POINT('Ctrl Pts',(-94.2459621805259,25.3214884497798,8.30392902067936));
#23489=CARTESIAN_POINT('Ctrl Pts',(-94.5122227023915,24.6575056999379,8.34567285909369));
#23490=CARTESIAN_POINT('Ctrl Pts',(-94.5182105203766,23.9978055611691,8.38741669750802));
#23491=CARTESIAN_POINT('Origin',(-92.,24.,5.));
#23492=CARTESIAN_POINT('',(-94.5201758362126,24.0015868137836,9.38741669750803));
#23493=CARTESIAN_POINT('',(-94.5149491154365,24.0017493991467,9.11258330249198));
#23494=CARTESIAN_POINT('',(-94.5175,24.,5.));
#23495=CARTESIAN_POINT('',(-90.0865340033349,25.6359872033749,10.));
#23496=CARTESIAN_POINT('Ctrl Pts',(-94.5201758362126,24.0015868137836,9.38741669750803));
#23497=CARTESIAN_POINT('Ctrl Pts',(-94.5146934294681,23.2729074143925,9.43362796642338));
#23498=CARTESIAN_POINT('Ctrl Pts',(-94.1807323142246,22.5399684977904,9.47983923533874));
#23499=CARTESIAN_POINT('Ctrl Pts',(-93.6239878020485,22.0711234457756,9.5260505042541));
#23500=CARTESIAN_POINT('Ctrl Pts',(-92.9895375021336,21.5368408846388,9.57871155933697));
#23501=CARTESIAN_POINT('Ctrl Pts',(-92.0657754031769,21.3455168748646,9.63137261441986));
#23502=CARTESIAN_POINT('Ctrl Pts',(-91.2718707713923,21.5853895680493,9.68403366950274));
#23503=CARTESIAN_POINT('Ctrl Pts',(-90.4779661396077,21.825262261234,9.73669472458561));
#23504=CARTESIAN_POINT('Ctrl Pts',(-89.8139189749953,22.4963316573775,9.78935577966849));
#23505=CARTESIAN_POINT('Ctrl Pts',(-89.5807324199303,23.2907313838813,9.84201683475137));
#23506=CARTESIAN_POINT('Ctrl Pts',(-89.3475458648653,24.0851311103851,9.89467788983425));
#23507=CARTESIAN_POINT('Ctrl Pts',(-89.5452199193478,25.0028611672492,9.94733894491713));
#23508=CARTESIAN_POINT('Ctrl Pts',(-90.0865340033349,25.635987203375,10.));
#23509=CARTESIAN_POINT('',(-93.9171032040961,25.6385343199284,10.));
#23510=CARTESIAN_POINT('Origin',(-92.,24.,10.));
#23511=CARTESIAN_POINT('Ctrl Pts',(-93.9171116625783,25.6385402433575,10.));
#23512=CARTESIAN_POINT('Ctrl Pts',(-93.3939569207211,26.2476959894343,9.94901908464118));
#23513=CARTESIAN_POINT('Ctrl Pts',(-92.5534186715195,26.5878275437024,9.89803816928235));
#23514=CARTESIAN_POINT('Ctrl Pts',(-91.7542642292644,26.5094851289584,9.84705725392353));
#23515=CARTESIAN_POINT('Ctrl Pts',(-90.9287726544835,26.4285608421126,9.79439619884065));
#23516=CARTESIAN_POINT('Ctrl Pts',(-90.1474375442602,25.9011254113112,9.74173514375777));
#23517=CARTESIAN_POINT('Ctrl Pts',(-89.7641120845165,25.1658537236911,9.68907408867489));
#23518=CARTESIAN_POINT('Ctrl Pts',(-89.3807866247728,24.4305820360709,9.63641303359201));
#23519=CARTESIAN_POINT('Ctrl Pts',(-89.3954708155088,23.487474091632,9.58375197850914));
#23520=CARTESIAN_POINT('Ctrl Pts',(-89.8017477031856,22.764502097224,9.53109092342626));
#23521=CARTESIAN_POINT('Ctrl Pts',(-90.2080245908623,22.041530102816,9.47842986834338));
#23522=CARTESIAN_POINT('Ctrl Pts',(-91.0058941754799,21.5386940584389,9.4257688132605));
#23523=CARTESIAN_POINT('Ctrl Pts',(-91.8333902143466,21.4839130383455,9.37310775817762));
#23524=CARTESIAN_POINT('Ctrl Pts',(-92.6608862532132,21.4291320182521,9.32044670309474));
#23525=CARTESIAN_POINT('Ctrl Pts',(-93.518008746329,21.8224060224424,9.26778564801187));
#23526=CARTESIAN_POINT('Ctrl Pts',(-94.016096172441,22.4854401035393,9.21512459292899));
#23527=CARTESIAN_POINT('Ctrl Pts',(-94.3393871214709,22.9157920981482,9.18094416278332));
#23528=CARTESIAN_POINT('Ctrl Pts',(-94.5114220034557,23.4597899508602,9.14676373263765));
#23529=CARTESIAN_POINT('Ctrl Pts',(-94.5149491154365,24.0017493991467,9.11258330249198));
#23530=CARTESIAN_POINT('Origin',(-92.,24.,12.2084234471775));
#23531=CARTESIAN_POINT('',(-95.0782766400089,24.0007881209763,1.79157655282254));
#23532=CARTESIAN_POINT('',(-95.0686108047355,24.0003349297086,1.70842344717745));
#23533=CARTESIAN_POINT('',(-95.0735,24.0000000000001,12.2084234471775));
#23534=CARTESIAN_POINT('',(-91.2062007174672,21.0307770462543,0.999999999999999));
#23535=CARTESIAN_POINT('Ctrl Pts',(-95.0686108047355,24.0003349297086,1.70842344717745));
#23536=CARTESIAN_POINT('Ctrl Pts',(-95.0689532420951,24.4946153833655,1.68292651844981));
#23537=CARTESIAN_POINT('Ctrl Pts',(-94.723556593627,26.0092287415617,1.6047685346393));
#23538=CARTESIAN_POINT('Ctrl Pts',(-92.3539160917337,27.6088396578189,1.4739494957459));
#23539=CARTESIAN_POINT('Ctrl Pts',(-89.1687762982368,26.2698556568796,1.31596633049727));
#23540=CARTESIAN_POINT('Ctrl Pts',(-88.5566852567634,22.8667001441213,1.15798316524863));
#23541=CARTESIAN_POINT('Ctrl Pts',(-90.2237466982397,21.2934286920664,1.05266105508288));
#23542=CARTESIAN_POINT('Ctrl Pts',(-91.2062007174672,21.0307770462543,0.999999999999999));
#23543=CARTESIAN_POINT('',(-92.7937992825328,21.0307770462543,1.));
#23544=CARTESIAN_POINT('Origin',(-92.,24.,0.999999999999999));
#23545=CARTESIAN_POINT('Ctrl Pts',(-95.078276640009,24.0007881209763,1.79157655282254));
#23546=CARTESIAN_POINT('Ctrl Pts',(-95.0784227334426,24.0437415110921,1.78934283757203));
#23547=CARTESIAN_POINT('Ctrl Pts',(-95.0582221315001,25.0992023691253,1.73444806723864));
#23548=CARTESIAN_POINT('Ctrl Pts',(-93.8523949517843,27.1179531681002,1.62689224182237));
#23549=CARTESIAN_POINT('Ctrl Pts',(-90.40096829048,27.2555127221398,1.46890907657374));
#23550=CARTESIAN_POINT('Ctrl Pts',(-88.4000492676845,24.4393710995325,1.3109259113251));
#23551=CARTESIAN_POINT('Ctrl Pts',(-89.6506968017519,21.2605902470593,1.15462288580053));
#23552=CARTESIAN_POINT('Ctrl Pts',(-91.8480943965222,20.7745943834541,1.05098091535883));
#23553=CARTESIAN_POINT('Ctrl Pts',(-92.7957016814436,21.0256872793281,1.));
#23554=CARTESIAN_POINT('Origin',(-92.,24.,12.2084234471775));
#23555=CARTESIAN_POINT('',(-95.069948942502,24.0019027882837,2.79157655282254));
#23556=CARTESIAN_POINT('',(-95.0750082483734,23.9974244677008,2.70842344717745));
#23557=CARTESIAN_POINT('',(-95.0735,24.0000000000001,12.2084234471775));
#23558=CARTESIAN_POINT('Ctrl Pts',(-95.0750082483734,23.9974244677008,2.70842344717745));
#23559=CARTESIAN_POINT('Ctrl Pts',(-95.0676141928259,24.8239896640293,2.66555951561375));
#23560=CARTESIAN_POINT('Ctrl Pts',(-94.2993639886886,26.6781669869539,2.57003452896717));
#23561=CARTESIAN_POINT('Ctrl Pts',(-91.1738622446318,27.5314376817822,2.42184848723771));
#23562=CARTESIAN_POINT('Ctrl Pts',(-88.5910236590807,25.2380222607046,2.26386532198907));
#23563=CARTESIAN_POINT('Ctrl Pts',(-89.1003115510402,21.8216058212252,2.10588215674044));
#23564=CARTESIAN_POINT('Ctrl Pts',(-92.2395757883417,20.3812154557911,1.94789899149181));
#23565=CARTESIAN_POINT('Ctrl Pts',(-94.6902007202701,21.9256564305863,1.81541275497081));
#23566=CARTESIAN_POINT('Ctrl Pts',(-95.068245976022,23.4737343794429,1.73558757353269));
#23567=CARTESIAN_POINT('Ctrl Pts',(-95.0686108047355,24.0003349297086,1.70842344717745));
#23568=CARTESIAN_POINT('Ctrl Pts',(-95.069948942502,24.0019027882837,2.79157655282254));
#23569=CARTESIAN_POINT('Ctrl Pts',(-95.0721210057469,24.3814602607307,2.77197583473597));
#23570=CARTESIAN_POINT('Ctrl Pts',(-94.831557865169,25.7781155062161,2.69971406156651));
#23571=CARTESIAN_POINT('Ctrl Pts',(-92.7514083303166,27.5481002919865,2.57479123331418));
#23572=CARTESIAN_POINT('Ctrl Pts',(-89.4392014827729,26.568262216555,2.41680806806554));
#23573=CARTESIAN_POINT('Ctrl Pts',(-88.4497281061605,23.25891107134,2.25882490281691));
#23574=CARTESIAN_POINT('Ctrl Pts',(-90.6804688187273,20.6217765261787,2.10084173756828));
#23575=CARTESIAN_POINT('Ctrl Pts',(-94.0596141395782,21.0427206231846,1.94509228757015));
#23576=CARTESIAN_POINT('Ctrl Pts',(-95.0749785010789,23.0310919164918,1.84200389265491));
#23577=CARTESIAN_POINT('Ctrl Pts',(-95.078276640009,24.0007881209763,1.79157655282254));
#23578=CARTESIAN_POINT('Origin',(-92.,24.,12.2084234471775));
#23579=CARTESIAN_POINT('',(-95.0716996757212,23.9974284306968,3.79157655282254));
#23580=CARTESIAN_POINT('',(-95.0762204956332,24.0022328813937,3.70842344717745));
#23581=CARTESIAN_POINT('',(-95.0735,24.0000000000001,12.2084234471775));
#23582=CARTESIAN_POINT('Ctrl Pts',(-95.0762204956332,24.0022328813937,3.70842344717745));
#23583=CARTESIAN_POINT('Ctrl Pts',(-95.0774152743553,24.1480569517706,3.70085356786056));
#23584=CARTESIAN_POINT('Ctrl Pts',(-95.0019699142738,25.3070874795556,3.6406226334608));
#23585=CARTESIAN_POINT('Ctrl Pts',(-93.5299145201094,27.2883129487163,3.52773064397815));
#23586=CARTESIAN_POINT('Ctrl Pts',(-90.0822081585387,27.0782646692958,3.36974747872952));
#23587=CARTESIAN_POINT('Ctrl Pts',(-88.3740039924776,24.0761257570407,3.21176431348088));
#23588=CARTESIAN_POINT('Ctrl Pts',(-89.9547029138477,21.0049371841951,3.05378114823225));
#23589=CARTESIAN_POINT('Ctrl Pts',(-93.3905541717124,20.6503748565914,2.89579798298361));
#23590=CARTESIAN_POINT('Ctrl Pts',(-94.9751243964845,22.605903680769,2.78067874929868));
#23591=CARTESIAN_POINT('Ctrl Pts',(-95.0766982584323,23.8085019627026,2.71822057069663));
#23592=CARTESIAN_POINT('Ctrl Pts',(-95.0750082483734,23.9974244677008,2.70842344717745));
#23593=CARTESIAN_POINT('Ctrl Pts',(-95.0716996757212,23.9974284306968,3.79157655282254));
#23594=CARTESIAN_POINT('Ctrl Pts',(-95.0659413561645,24.7122593975924,3.7546088318999));
#23595=CARTESIAN_POINT('Ctrl Pts',(-94.4623933413542,26.4541466296604,3.66498005589438));
#23596=CARTESIAN_POINT('Ctrl Pts',(-91.5706310470027,27.6012890799135,3.52269022480599));
#23597=CARTESIAN_POINT('Ctrl Pts',(-88.7493847378944,25.6084593551841,3.36470705955735));
#23598=CARTESIAN_POINT('Ctrl Pts',(-88.8765574469373,22.156701935519,3.20672389430872));
#23599=CARTESIAN_POINT('Ctrl Pts',(-91.836799110436,20.3768791020246,3.04874072906008));
#23600=CARTESIAN_POINT('Ctrl Pts',(-94.5594315108872,21.6964445021905,2.91035828189803));
#23601=CARTESIAN_POINT('Ctrl Pts',(-95.0662853449471,23.3617069600934,2.82463688981885));
#23602=CARTESIAN_POINT('Ctrl Pts',(-95.069948942502,24.0019027882837,2.79157655282254));
#23603=CARTESIAN_POINT('Origin',(-92.,24.,12.2084234471775));
#23604=CARTESIAN_POINT('',(-95.0783836922344,24.0005832748178,4.79157655282255));
#23605=CARTESIAN_POINT('',(-95.0687189181701,24.0004324466973,4.70842344717745));
#23606=CARTESIAN_POINT('',(-95.0735,24.0000000000001,12.2084234471775));
#23607=CARTESIAN_POINT('Ctrl Pts',(-95.0687189181701,24.0004324466973,4.70842344717745));
#23608=CARTESIAN_POINT('Ctrl Pts',(-95.0693320714153,24.4838070199057,4.6834865650245));
#23609=CARTESIAN_POINT('Ctrl Pts',(-94.7346949951819,25.9871566204806,4.60588862778867));
#23610=CARTESIAN_POINT('Ctrl Pts',(-92.3913282534434,27.6056209517321,4.47562963546996));
#23611=CARTESIAN_POINT('Ctrl Pts',(-89.1942539711864,26.2981360810345,4.31764647022133));
#23612=CARTESIAN_POINT('Ctrl Pts',(-88.5420870968054,22.9061633512837,4.15966330497268));
#23613=CARTESIAN_POINT('Ctrl Pts',(-91.0263652646397,20.5063377831117,4.00168013972405));
#23614=CARTESIAN_POINT('Ctrl Pts',(-94.2324119925839,21.238533748243,3.85126685379231));
#23615=CARTESIAN_POINT('Ctrl Pts',(-95.0691036084142,23.1336088897796,3.75351462294344));
#23616=CARTESIAN_POINT('Ctrl Pts',(-95.0762204956332,24.0022328813937,3.70842344717745));
#23617=CARTESIAN_POINT('Ctrl Pts',(-95.0783836922344,24.0005832748178,4.79157655282255));
#23618=CARTESIAN_POINT('Ctrl Pts',(-95.0784682719039,24.0327646232159,4.78990288414672));
#23619=CARTESIAN_POINT('Ctrl Pts',(-95.0634880644544,25.0774335875127,4.73556816038801));
#23620=CARTESIAN_POINT('Ctrl Pts',(-93.8851896583918,27.0983384007903,4.62857238154643));
#23621=CARTESIAN_POINT('Ctrl Pts',(-90.4354577715253,27.2719792949116,4.47058921629779));
#23622=CARTESIAN_POINT('Ctrl Pts',(-88.4048190868975,24.4778232899584,4.31260605104916));
#23623=CARTESIAN_POINT('Ctrl Pts',(-89.6351322020287,21.2502652496794,4.15462288580053));
#23624=CARTESIAN_POINT('Ctrl Pts',(-93.0104611272249,20.5168104867762,3.99663972055189));
#23625=CARTESIAN_POINT('Ctrl Pts',(-94.8939119603259,22.3750681296892,3.8756242762259));
#23626=CARTESIAN_POINT('Ctrl Pts',(-95.0741441659616,23.693972308664,3.80726988698278));
#23627=CARTESIAN_POINT('Ctrl Pts',(-95.0716996757212,23.9974284306968,3.79157655282254));
#23628=CARTESIAN_POINT('Origin',(-92.,24.,12.2084234471775));
#23629=CARTESIAN_POINT('',(-95.0701623993453,24.0020253450063,5.79157655282255));
#23630=CARTESIAN_POINT('',(-95.0746893422024,23.9973677267576,5.70842344717746));
#23631=CARTESIAN_POINT('',(-95.0735,24.0000000000001,12.2084234471775));
#23632=CARTESIAN_POINT('Ctrl Pts',(-95.0746893422024,23.9973677267576,5.70842344717746));
#23633=CARTESIAN_POINT('Ctrl Pts',(-95.0673208895816,24.8133508051794,5.66611956218844));
#23634=CARTESIAN_POINT('Ctrl Pts',(-94.3157336914086,26.657090117177,5.57115462211653));
#23635=CARTESIAN_POINT('Ctrl Pts',(-91.2111785026033,27.5399718768618,5.42352862696177));
#23636=CARTESIAN_POINT('Ctrl Pts',(-88.6043014164073,25.2739196885051,5.26554546171313));
#23637=CARTESIAN_POINT('Ctrl Pts',(-89.0774388479143,21.8523788611612,5.1075622964645));
#23638=CARTESIAN_POINT('Ctrl Pts',(-92.2014389978195,20.3788037094653,4.94957913121586));
#23639=CARTESIAN_POINT('Ctrl Pts',(-94.6784589321776,21.9039237459708,4.81653284812018));
#23640=CARTESIAN_POINT('Ctrl Pts',(-95.0680372304395,23.4630292470767,4.73614762010738));
#23641=CARTESIAN_POINT('Ctrl Pts',(-95.0687189181701,24.0004324466973,4.70842344717745));
#23642=CARTESIAN_POINT('Ctrl Pts',(-95.0701623993453,24.0020253450063,5.79157655282255));
#23643=CARTESIAN_POINT('Ctrl Pts',(-95.0724185577781,24.3706733312739,5.77253588131065));
#23644=CARTESIAN_POINT('Ctrl Pts',(-94.8409293691539,25.7561580997578,5.70083415471588));
#23645=CARTESIAN_POINT('Ctrl Pts',(-92.7888215168717,27.5399719642595,5.57647137303824));
#23646=CARTESIAN_POINT('Ctrl Pts',(-89.466456326301,26.5951488100944,5.4184882077896));
#23647=CARTESIAN_POINT('Ctrl Pts',(-88.4421017230707,23.2964371072189,5.26050504254096));
#23648=CARTESIAN_POINT('Ctrl Pts',(-90.6448822957048,20.6358809621643,5.10252187729233));
#23649=CARTESIAN_POINT('Ctrl Pts',(-94.0404432418415,21.0225553310303,4.94621238071953));
#23650=CARTESIAN_POINT('Ctrl Pts',(-95.075807019589,23.0201963741307,4.8425639392296));
#23651=CARTESIAN_POINT('Ctrl Pts',(-95.0783836922344,24.0005832748178,4.79157655282255));
#23652=CARTESIAN_POINT('Origin',(-92.,24.,12.2084234471775));
#23653=CARTESIAN_POINT('',(-95.0714153574487,23.9974952077453,6.79157655282255));
#23654=CARTESIAN_POINT('',(-95.0765039205242,24.0021186989273,6.70842344717745));
#23655=CARTESIAN_POINT('',(-95.0735,24.0000000000001,12.2084234471775));
#23656=CARTESIAN_POINT('Ctrl Pts',(-95.0765039205242,24.0021186989273,6.70842344717745));
#23657=CARTESIAN_POINT('Ctrl Pts',(-95.0775698549681,24.1371216997451,6.70141361443525));
#23658=CARTESIAN_POINT('Ctrl Pts',(-95.00840225429,25.2852297742064,6.64174272661017));
#23659=CARTESIAN_POINT('Ctrl Pts',(-93.5645421898479,27.2719792141301,6.5294107837022));
#23660=CARTESIAN_POINT('Ctrl Pts',(-90.1148103881513,27.0983383242962,6.37142761845358));
#23661=CARTESIAN_POINT('Ctrl Pts',(-88.3750099098822,24.1143988208681,6.21344445320493));
#23662=CARTESIAN_POINT('Ctrl Pts',(-89.9231991720716,21.0266956824956,6.05546128795631));
#23663=CARTESIAN_POINT('Ctrl Pts',(-93.355117670839,20.6358810452204,5.89747812270766));
#23664=CARTESIAN_POINT('Ctrl Pts',(-94.9680494317644,22.584007681798,5.78179884244806));
#23665=CARTESIAN_POINT('Ctrl Pts',(-95.0764933447696,23.7975923269541,5.71878061727132));
#23666=CARTESIAN_POINT('Ctrl Pts',(-95.0746893422024,23.9973677267576,5.70842344717746));
#23667=CARTESIAN_POINT('Ctrl Pts',(-95.0714153574487,23.9974952077453,6.79157655282255));
#23668=CARTESIAN_POINT('Ctrl Pts',(-95.0659291292545,24.7016618298241,6.75516887847459));
#23669=CARTESIAN_POINT('Ctrl Pts',(-94.4768296167088,26.4326507862167,6.66610014904375));
#23670=CARTESIAN_POINT('Ctrl Pts',(-91.6086717368946,27.6056210407497,6.52437036453005));
#23671=CARTESIAN_POINT('Ctrl Pts',(-88.7665454640887,25.6426845888844,6.3663871992814));
#23672=CARTESIAN_POINT('Ctrl Pts',(-88.8572728216189,22.1897771481732,6.20840403403277));
#23673=CARTESIAN_POINT('Ctrl Pts',(-91.7985609972073,20.3788036200624,6.05042086878414));
#23674=CARTESIAN_POINT('Ctrl Pts',(-94.5460460301537,21.6747784855977,5.9114783750474));
#23675=CARTESIAN_POINT('Ctrl Pts',(-95.0661786684217,23.351098370438,5.82519693639353));
#23676=CARTESIAN_POINT('Ctrl Pts',(-95.0701623993453,24.0020253450063,5.79157655282255));
#23677=CARTESIAN_POINT('Origin',(-92.,24.,12.2084234471775));
#23678=CARTESIAN_POINT('',(-95.0784606140442,24.000390174329,7.79157655282255));
#23679=CARTESIAN_POINT('',(-95.0687739277024,24.0006038359779,7.70842344717745));
#23680=CARTESIAN_POINT('',(-95.0735,24.0000000000001,12.2084234471775));
#23681=CARTESIAN_POINT('Ctrl Pts',(-95.0687739277024,24.0006038359779,7.70842344717745));
#23682=CARTESIAN_POINT('Ctrl Pts',(-95.0696117452305,24.4731013478073,7.68404661159918));
#23683=CARTESIAN_POINT('Ctrl Pts',(-94.745518655979,25.9652418365262,7.60700872093803));
#23684=CARTESIAN_POINT('Ctrl Pts',(-92.4293689423973,27.6012889909868,7.47730977519402));
#23685=CARTESIAN_POINT('Ctrl Pts',(-89.2186704291244,26.3276267101463,7.31932660994537));
#23686=CARTESIAN_POINT('Ctrl Pts',(-88.5307327633938,22.9427275180138,7.16134344469675));
#23687=CARTESIAN_POINT('Ctrl Pts',(-90.9895388977222,20.516810572774,7.00336027944811));
#23688=CARTESIAN_POINT('Ctrl Pts',(-94.2151018414648,21.2177213748182,6.85238694694168));
#23689=CARTESIAN_POINT('Ctrl Pts',(-95.0695620701134,23.1229176917646,6.75407466951813));
#23690=CARTESIAN_POINT('Ctrl Pts',(-95.0765039205242,24.0021186989273,6.70842344717745));
#23691=CARTESIAN_POINT('Ctrl Pts',(-95.0784606140442,24.000390174329,7.79157655282255));
#23692=CARTESIAN_POINT('Ctrl Pts',(-95.0784992224434,24.0218014961978,7.79046293072141));
#23693=CARTESIAN_POINT('Ctrl Pts',(-95.0686358124042,25.0556766999574,7.73668825353738));
#23694=CARTESIAN_POINT('Ctrl Pts',(-93.9177918888646,27.0782647453892,7.63025252127048));
#23695=CARTESIAN_POINT('Ctrl Pts',(-90.4700854420894,27.288313029852,7.47226935602185));
#23696=CARTESIAN_POINT('Ctrl Pts',(-88.4100634919605,24.5157489192992,7.31428619077322));
#23697=CARTESIAN_POINT('Ctrl Pts',(-89.6062365978313,21.275383052732,7.15630302552458));
#23698=CARTESIAN_POINT('Ctrl Pts',(-92.9736347594024,20.5063376968639,6.99831986027594));
#23699=CARTESIAN_POINT('Ctrl Pts',(-94.8854039328386,22.3531166132715,6.87674436937527));
#23700=CARTESIAN_POINT('Ctrl Pts',(-95.0738645596358,23.6831359850142,6.80782993355747));
#23701=CARTESIAN_POINT('Ctrl Pts',(-95.0714153574487,23.9974952077453,6.79157655282255));
#23702=CARTESIAN_POINT('Origin',(-92.,24.,12.2084234471775));
#23703=CARTESIAN_POINT('',(-95.0703857423214,24.0021357609841,8.79157655282255));
#23704=CARTESIAN_POINT('',(-95.0743674416594,23.9973209105276,8.70842344717745));
#23705=CARTESIAN_POINT('',(-95.0735,24.0000000000001,12.2084234471775));
#23706=CARTESIAN_POINT('Ctrl Pts',(-95.0743674416594,23.9973209105276,8.70842344717745));
#23707=CARTESIAN_POINT('Ctrl Pts',(-95.0670571899902,24.8027184781565,8.66667960876312));
#23708=CARTESIAN_POINT('Ctrl Pts',(-94.3319128073199,26.6359725607219,8.57227471526591));
#23709=CARTESIAN_POINT('Ctrl Pts',(-91.2485916883301,27.5481002036266,8.42520876668582));
#23710=CARTESIAN_POINT('Ctrl Pts',(-88.617938794798,25.3096959362796,8.26722560143718));
#23711=CARTESIAN_POINT('Ctrl Pts',(-89.0549304174884,21.8833499742238,8.10924243618856));
#23712=CARTESIAN_POINT('Ctrl Pts',(-92.1632008855268,20.3768791915845,7.95125927093991));
#23713=CARTESIAN_POINT('Ctrl Pts',(-94.6666765768248,21.8820749507615,7.81765294126956));
#23714=CARTESIAN_POINT('Ctrl Pts',(-95.0678018156825,23.4523692918733,7.73670766668206));
#23715=CARTESIAN_POINT('Ctrl Pts',(-95.0687739277024,24.0006038359779,7.70842344717745));
#23716=CARTESIAN_POINT('Ctrl Pts',(-95.0703857423214,24.0021357609841,8.79157655282255));
#23717=CARTESIAN_POINT('Ctrl Pts',(-95.0727139521361,24.3598775376807,8.77309592788534));
#23718=CARTESIAN_POINT('Ctrl Pts',(-94.8501666541559,25.7342139358697,8.70195424786526));
#23719=CARTESIAN_POINT('Ctrl Pts',(-92.8261377777637,27.5314377737091,8.57815151276228));
#23720=CARTESIAN_POINT('Ctrl Pts',(-89.493997547754,26.6217541894133,8.42016834751367));
#23721=CARTESIAN_POINT('Ctrl Pts',(-88.4348706359932,23.3340326759415,8.26218518226501));
#23722=CARTESIAN_POINT('Ctrl Pts',(-90.6094457936036,20.6503747732117,8.10420201701639));
#23723=CARTESIAN_POINT('Ctrl Pts',(-94.0210778474872,21.0024378034505,7.94733247386889));
#23724=CARTESIAN_POINT('Ctrl Pts',(-95.0766735052339,23.0093011164261,7.84312398580429));
#23725=CARTESIAN_POINT('Ctrl Pts',(-95.0784606140442,24.000390174329,7.79157655282255));
#23726=CARTESIAN_POINT('Origin',(-92.,24.,12.2084234471775));
#23727=CARTESIAN_POINT('',(-95.0702888275776,23.9968971804147,9.79157655282255));
#23728=CARTESIAN_POINT('',(-95.076766805402,24.0019372679897,9.70842344717746));
#23729=CARTESIAN_POINT('',(-95.0735,24.0000000000001,12.2084234471775));
#23730=CARTESIAN_POINT('',(-92.7937992825329,21.0307770462543,10.));
#23731=CARTESIAN_POINT('Ctrl Pts',(-92.7937992825329,21.0307770462543,10.));
#23732=CARTESIAN_POINT('Ctrl Pts',(-93.7762533017603,21.2934286920664,9.94733894491712));
#23733=CARTESIAN_POINT('Ctrl Pts',(-94.8759105460538,22.3312191677288,9.87786446252464));
#23734=CARTESIAN_POINT('Ctrl Pts',(-95.0726356002046,23.6716361186704,9.80838998013215));
#23735=CARTESIAN_POINT('Ctrl Pts',(-95.0702888275776,23.9968971804147,9.79157655282255));
#23736=CARTESIAN_POINT('',(-91.2043027735401,21.0256991239339,10.));
#23737=CARTESIAN_POINT('Origin',(-92.,24.,10.));
#23738=CARTESIAN_POINT('Ctrl Pts',(-91.2042983602307,21.0256873161864,10.));
#23739=CARTESIAN_POINT('Ctrl Pts',(-92.1519057059922,20.7745943606123,9.94901908464117));
#23740=CARTESIAN_POINT('Ctrl Pts',(-94.2125558943073,21.2303462451956,9.85182690036699));
#23741=CARTESIAN_POINT('Ctrl Pts',(-95.0700735870785,23.1123260926059,9.75463471609281));
#23742=CARTESIAN_POINT('Ctrl Pts',(-95.076766805402,24.0019372679897,9.70842344717746));
#23743=CARTESIAN_POINT('Origin',(46.,-46.,36.));
#23744=CARTESIAN_POINT('',(39.,-46.,40.));
#23745=CARTESIAN_POINT('Origin',(46.,-46.,40.));
#23746=CARTESIAN_POINT('',(39.,-46.,32.));
#23747=CARTESIAN_POINT('',(39.,-46.,36.));
#23748=CARTESIAN_POINT('Origin',(46.,-46.,32.));
#23749=CARTESIAN_POINT('Origin',(46.,-46.,32.));
#23750=CARTESIAN_POINT('',(41.5,-46.,32.));
#23751=CARTESIAN_POINT('Origin',(46.,-46.,32.));
#23752=CARTESIAN_POINT('Origin',(-46.,-46.,36.));
#23753=CARTESIAN_POINT('',(-53.,-46.,40.));
#23754=CARTESIAN_POINT('Origin',(-46.,-46.,40.));
#23755=CARTESIAN_POINT('',(-53.,-46.,32.));
#23756=CARTESIAN_POINT('',(-53.,-46.,36.));
#23757=CARTESIAN_POINT('Origin',(-46.,-46.,32.));
#23758=CARTESIAN_POINT('Origin',(-46.,-46.,32.));
#23759=CARTESIAN_POINT('',(-50.5,-46.,32.));
#23760=CARTESIAN_POINT('Origin',(-46.,-46.,32.));
#23761=CARTESIAN_POINT('Origin',(-46.,46.,36.));
#23762=CARTESIAN_POINT('',(-53.,46.,40.));
#23763=CARTESIAN_POINT('Origin',(-46.,46.,40.));
#23764=CARTESIAN_POINT('',(-53.,46.,32.));
#23765=CARTESIAN_POINT('',(-53.,46.,36.));
#23766=CARTESIAN_POINT('Origin',(-46.,46.,32.));
#23767=CARTESIAN_POINT('Origin',(-46.,46.,32.));
#23768=CARTESIAN_POINT('',(-50.5,46.,32.));
#23769=CARTESIAN_POINT('Origin',(-46.,46.,32.));
#23770=CARTESIAN_POINT('Origin',(46.,46.,36.));
#23771=CARTESIAN_POINT('',(39.,46.,40.));
#23772=CARTESIAN_POINT('Origin',(46.,46.,40.));
#23773=CARTESIAN_POINT('',(39.,46.,32.));
#23774=CARTESIAN_POINT('',(39.,46.,36.));
#23775=CARTESIAN_POINT('Origin',(46.,46.,32.));
#23776=CARTESIAN_POINT('Origin',(46.,46.,32.));
#23777=CARTESIAN_POINT('',(41.5,46.,32.));
#23778=CARTESIAN_POINT('Origin',(46.,46.,32.));
#23779=CARTESIAN_POINT('Origin',(46.,-46.,20.));
#23780=CARTESIAN_POINT('',(41.5,-46.,0.));
#23781=CARTESIAN_POINT('',(41.5,-46.,20.));
#23782=CARTESIAN_POINT('Origin',(46.,-46.,0.));
#23783=CARTESIAN_POINT('Origin',(-46.,-46.,20.));
#23784=CARTESIAN_POINT('',(-50.5,-46.,0.));
#23785=CARTESIAN_POINT('',(-50.5,-46.,20.));
#23786=CARTESIAN_POINT('Origin',(-46.,-46.,0.));
#23787=CARTESIAN_POINT('Origin',(-46.,46.,20.));
#23788=CARTESIAN_POINT('',(-50.5,46.,0.));
#23789=CARTESIAN_POINT('',(-50.5,46.,20.));
#23790=CARTESIAN_POINT('Origin',(-46.,46.,0.));
#23791=CARTESIAN_POINT('Origin',(46.,46.,20.));
#23792=CARTESIAN_POINT('',(41.5,46.,0.));
#23793=CARTESIAN_POINT('',(41.5,46.,20.));
#23794=CARTESIAN_POINT('Origin',(46.,46.,0.));
#23795=CARTESIAN_POINT('Origin',(-92.,24.,1.));
#23796=CARTESIAN_POINT('Ctrl Pts',(-93.913465996665,25.635987203375,0.999999999999999));
#23797=CARTESIAN_POINT('Ctrl Pts',(-93.9756063047087,25.5775905725136,0.999999999999998));
#23798=CARTESIAN_POINT('Ctrl Pts',(-94.0343713138295,25.5159402489924,0.999999999999998));
#23799=CARTESIAN_POINT('Ctrl Pts',(-94.0897489850203,25.4514126613156,0.999999999999998));
#23800=CARTESIAN_POINT('Ctrl Pts',(-94.1464813764675,25.3853065162843,0.999999999999998));
#23801=CARTESIAN_POINT('Ctrl Pts',(-94.1996591403008,25.3161801193169,1.));
#23802=CARTESIAN_POINT('Ctrl Pts',(-94.2492404445121,25.2443919311763,1.));
#23803=CARTESIAN_POINT('Ctrl Pts',(-94.2621841917327,25.2256508315724,1.));
#23804=CARTESIAN_POINT('Ctrl Pts',(-94.2748826589411,25.2067281064344,0.999999999999997));
#23805=CARTESIAN_POINT('Ctrl Pts',(-94.2873347259112,25.1876296997861,0.999999999999997));
#23806=CARTESIAN_POINT('Ctrl Pts',(-94.2974956811874,25.1720452947016,0.999999999999996));
#23807=CARTESIAN_POINT('Ctrl Pts',(-94.3074930002328,25.1563430139423,1.));
#23808=CARTESIAN_POINT('Ctrl Pts',(-94.3173172477238,25.1405406475386,1.));
#23809=CARTESIAN_POINT('Ctrl Pts',(-94.3647645434793,25.0642213617018,1.));
#23810=CARTESIAN_POINT('Ctrl Pts',(-94.4082282646501,24.9854948529656,0.999999999999998));
#23811=CARTESIAN_POINT('Ctrl Pts',(-94.447673659524,24.9047536078528,0.999999999999998));
#23812=CARTESIAN_POINT('Ctrl Pts',(-94.4795145183608,24.8395781774593,0.999999999999999));
#23813=CARTESIAN_POINT('Ctrl Pts',(-94.5087365608418,24.773088868802,1.));
#23814=CARTESIAN_POINT('Ctrl Pts',(-94.5353043306397,24.7054742948633,1.));
#23815=CARTESIAN_POINT('Ctrl Pts',(-94.5460290352188,24.6781800832584,1.));
#23816=CARTESIAN_POINT('Ctrl Pts',(-94.5563210329607,24.6507023520544,0.999999999999999));
#23817=CARTESIAN_POINT('Ctrl Pts',(-94.5661772012358,24.623052941431,0.999999999999999));
#23818=CARTESIAN_POINT('Ctrl Pts',(-94.5713953813417,24.6084144327908,0.999999999999999));
#23819=CARTESIAN_POINT('Ctrl Pts',(-94.5764908417308,24.5937291306026,0.999999999999998));
#23820=CARTESIAN_POINT('Ctrl Pts',(-94.5814593622078,24.5790106095272,0.999999999999998));
#23821=CARTESIAN_POINT('Ctrl Pts',(-94.610973429931,24.4915794658263,0.999999999999998));
#23822=CARTESIAN_POINT('Ctrl Pts',(-94.6360512221953,24.4028684394346,1.));
#23823=CARTESIAN_POINT('Ctrl Pts',(-94.6566599719052,24.3132752235806,1.));
#23824=CARTESIAN_POINT('Ctrl Pts',(-94.6775876507752,24.2222955146362,1.));
#23825=CARTESIAN_POINT('Ctrl Pts',(-94.6939073964014,24.130405294356,0.999999999999997));
#23826=CARTESIAN_POINT('Ctrl Pts',(-94.7055430522835,24.037987869175,0.999999999999997));
#23827=CARTESIAN_POINT('Ctrl Pts',(-94.7170875472974,23.9462944988128,0.999999999999997));
#23828=CARTESIAN_POINT('Ctrl Pts',(-94.724021404917,23.8540812223222,0.999999999999998));
#23829=CARTESIAN_POINT('Ctrl Pts',(-94.7262232902698,23.7617032481877,0.999999999999999));
#23830=CARTESIAN_POINT('Ctrl Pts',(-94.7273184961164,23.7157549442746,0.999999999999999));
#23831=CARTESIAN_POINT('Ctrl Pts',(-94.7272422422959,23.6697656818021,1.));
#23832=CARTESIAN_POINT('Ctrl Pts',(-94.7259748077026,23.6237784781036,1.));
#23833=CARTESIAN_POINT('Ctrl Pts',(-94.7255580392477,23.6086565807406,1.));
#23834=CARTESIAN_POINT('Ctrl Pts',(-94.7250123596335,23.5935330552964,0.999999999999996));
#23835=CARTESIAN_POINT('Ctrl Pts',(-94.7243372521877,23.5784152548529,0.999999999999996));
#23836=CARTESIAN_POINT('Ctrl Pts',(-94.7200633700785,23.4827094568323,0.999999999999996));
#23837=CARTESIAN_POINT('Ctrl Pts',(-94.7106224525511,23.3875708315057,0.999999999999995));
#23838=CARTESIAN_POINT('Ctrl Pts',(-94.6959503273247,23.2933977070033,0.999999999999996));
#23839=CARTESIAN_POINT('Ctrl Pts',(-94.6917956792088,23.2667310729442,0.999999999999996));
#23840=CARTESIAN_POINT('Ctrl Pts',(-94.6872212839362,23.2401417258322,0.999999999999998));
#23841=CARTESIAN_POINT('Ctrl Pts',(-94.6822249702578,23.2136384506288,0.999999999999998));
#23842=CARTESIAN_POINT('Ctrl Pts',(-94.6652600471295,23.1236468977724,0.999999999999998));
#23843=CARTESIAN_POINT('Ctrl Pts',(-94.6434348327879,23.0346478147206,0.999999999999998));
#23844=CARTESIAN_POINT('Ctrl Pts',(-94.6170519644753,22.9468734390333,0.999999999999998));
#23845=CARTESIAN_POINT('Ctrl Pts',(-94.5900726212507,22.8571146235805,0.999999999999999));
#23846=CARTESIAN_POINT('Ctrl Pts',(-94.5583270022639,22.7686358185468,1.));
#23847=CARTESIAN_POINT('Ctrl Pts',(-94.5220844975755,22.6816890800785,0.999999999999999));
#23848=CARTESIAN_POINT('Ctrl Pts',(-94.5094176334808,22.6513009341951,0.999999999999999));
#23849=CARTESIAN_POINT('Ctrl Pts',(-94.4962010035889,22.6211000168438,0.999999999999998));
#23850=CARTESIAN_POINT('Ctrl Pts',(-94.4824446757977,22.591097444797,0.999999999999998));
#23851=CARTESIAN_POINT('Ctrl Pts',(-94.4754977537663,22.5759461971739,0.999999999999997));
#23852=CARTESIAN_POINT('Ctrl Pts',(-94.4684131849647,22.5608455360005,0.999999999999999));
#23853=CARTESIAN_POINT('Ctrl Pts',(-94.4611921986787,22.5457969186967,1.));
#23854=CARTESIAN_POINT('Ctrl Pts',(-94.4551822280867,22.5332720718318,1.));
#23855=CARTESIAN_POINT('Ctrl Pts',(-94.4490796032345,22.5207872106202,1.));
#23856=CARTESIAN_POINT('Ctrl Pts',(-94.4428889228564,22.5083503604479,1.));
#23857=CARTESIAN_POINT('Ctrl Pts',(-94.3999256375741,22.4220386936643,1.));
#23858=CARTESIAN_POINT('Ctrl Pts',(-94.3526753109166,22.3379337018791,1.));
#23859=CARTESIAN_POINT('Ctrl Pts',(-94.3014800103383,22.2562854637047,1.));
#23860=CARTESIAN_POINT('Ctrl Pts',(-94.2492799079211,22.1730347288376,1.));
#23861=CARTESIAN_POINT('Ctrl Pts',(-94.1929781399576,22.0923373565558,1.));
#23862=CARTESIAN_POINT('Ctrl Pts',(-94.1328823961135,22.0144657633818,1.));
#23863=CARTESIAN_POINT('Ctrl Pts',(-94.0723186325409,21.9359877139172,1.));
#23864=CARTESIAN_POINT('Ctrl Pts',(-94.0079011060885,21.8603787916184,0.999999999999999));
#23865=CARTESIAN_POINT('Ctrl Pts',(-93.9398956019456,21.7879374141084,0.999999999999999));
#23866=CARTESIAN_POINT('Ctrl Pts',(-93.9029689977178,21.7486021557239,0.999999999999999));
#23867=CARTESIAN_POINT('Ctrl Pts',(-93.8649836956945,21.7102012375533,1.));
#23868=CARTESIAN_POINT('Ctrl Pts',(-93.8259770071998,21.6727861926027,1.));
#23869=CARTESIAN_POINT('Ctrl Pts',(-93.8138450048983,21.6611492290723,1.));
#23870=CARTESIAN_POINT('Ctrl Pts',(-93.8016141734242,21.6496076574392,0.999999999999998));
#23871=CARTESIAN_POINT('Ctrl Pts',(-93.7892855705602,21.6381630928521,0.999999999999998));
#23872=CARTESIAN_POINT('Ctrl Pts',(-93.7779997461575,21.6276865329596,0.999999999999997));
#23873=CARTESIAN_POINT('Ctrl Pts',(-93.7666377236851,21.6172966268635,1.));
#23874=CARTESIAN_POINT('Ctrl Pts',(-93.7552049282741,21.6069982199581,1.));
#23875=CARTESIAN_POINT('Ctrl Pts',(-93.6793958597524,21.5387111032299,1.));
#23876=CARTESIAN_POINT('Ctrl Pts',(-93.6004205023376,21.4743910085569,0.999999999999999));
#23877=CARTESIAN_POINT('Ctrl Pts',(-93.5186050201243,21.4143205611548,0.999999999999999));
#23878=CARTESIAN_POINT('Ctrl Pts',(-93.436718607489,21.3541980353187,0.999999999999999));
#23879=CARTESIAN_POINT('Ctrl Pts',(-93.3519865665313,21.2983316912964,0.999999999999998));
#23880=CARTESIAN_POINT('Ctrl Pts',(-93.264690947132,21.2470310933275,0.999999999999998));
#23881=CARTESIAN_POINT('Ctrl Pts',(-93.1791590995957,21.1967670027101,0.999999999999999));
#23882=CARTESIAN_POINT('Ctrl Pts',(-93.0911655548093,21.1508853499643,0.999999999999997));
#23883=CARTESIAN_POINT('Ctrl Pts',(-93.0009418597692,21.1097134459682,0.999999999999997));
#23884=CARTESIAN_POINT('Ctrl Pts',(-92.9631524544841,21.0924689541994,0.999999999999997));
#23885=CARTESIAN_POINT('Ctrl Pts',(-92.9249714624208,21.07605118337,0.999999999999999));
#23886=CARTESIAN_POINT('Ctrl Pts',(-92.8864145036881,21.0604865582877,0.999999999999999));
#23887=CARTESIAN_POINT('Ctrl Pts',(-92.8564008056109,21.0483706660271,0.999999999999999));
#23888=CARTESIAN_POINT('Ctrl Pts',(-92.8261592741354,21.0367717663531,0.999999999999999));
#23889=CARTESIAN_POINT('Ctrl Pts',(-92.7957016814436,21.0256872793281,0.999999999999999));
#23890=CARTESIAN_POINT('Ctrl Pts',(-91.2062007174672,21.0307770462543,0.999999999999999));
#23891=CARTESIAN_POINT('Ctrl Pts',(-91.1113643609119,21.0654686091134,0.999999999999998));
#23892=CARTESIAN_POINT('Ctrl Pts',(-91.0185712349542,21.1051505773263,0.999999999999999));
#23893=CARTESIAN_POINT('Ctrl Pts',(-90.928062273623,21.1495027068259,0.999999999999997));
#23894=CARTESIAN_POINT('Ctrl Pts',(-90.8362818390432,21.1944778966871,0.999999999999996));
#23895=CARTESIAN_POINT('Ctrl Pts',(-90.7468495275144,21.244256084386,0.999999999999996));
#23896=CARTESIAN_POINT('Ctrl Pts',(-90.6600505960964,21.2985440193193,0.999999999999996));
#23897=CARTESIAN_POINT('Ctrl Pts',(-90.6355418278817,21.3138728994379,0.999999999999996));
#23898=CARTESIAN_POINT('Ctrl Pts',(-90.6112432552945,21.3295615450785,0.999999999999992));
#23899=CARTESIAN_POINT('Ctrl Pts',(-90.5871618961064,21.3456038099433,0.999999999999992));
#23900=CARTESIAN_POINT('Ctrl Pts',(-90.5678312417006,21.3584813006018,0.999999999999992));
#23901=CARTESIAN_POINT('Ctrl Pts',(-90.5486384466368,21.3715882772414,0.999999999999994));
#23902=CARTESIAN_POINT('Ctrl Pts',(-90.52960642948,21.3849077947694,0.999999999999994));
#23903=CARTESIAN_POINT('Ctrl Pts',(-90.446898789443,21.4427905642147,0.999999999999994));
#23904=CARTESIAN_POINT('Ctrl Pts',(-90.367145983118,21.5047351112166,0.999999999999995));
#23905=CARTESIAN_POINT('Ctrl Pts',(-90.2906143666657,21.570444201942,0.999999999999996));
#23906=CARTESIAN_POINT('Ctrl Pts',(-90.2316015138477,21.6211119008557,0.999999999999996));
#23907=CARTESIAN_POINT('Ctrl Pts',(-90.1745045557113,21.6740188392933,0.999999999999995));
#23908=CARTESIAN_POINT('Ctrl Pts',(-90.1194631968057,21.7290405248296,0.999999999999995));
#23909=CARTESIAN_POINT('Ctrl Pts',(-90.0901430626928,21.758350179081,0.999999999999995));
#23910=CARTESIAN_POINT('Ctrl Pts',(-90.0614065056815,21.7882600664935,0.999999999999998));
#23911=CARTESIAN_POINT('Ctrl Pts',(-90.0332766727044,21.8187522035138,0.999999999999998));
#23912=CARTESIAN_POINT('Ctrl Pts',(-90.0236426846049,21.8291952404639,0.999999999999998));
#23913=CARTESIAN_POINT('Ctrl Pts',(-90.0140806611891,21.8397057918699,0.999999999999991));
#23914=CARTESIAN_POINT('Ctrl Pts',(-90.004598089186,21.850275607196,0.999999999999991));
#23915=CARTESIAN_POINT('Ctrl Pts',(-89.9388055962019,21.9236116704984,0.999999999999992));
#23916=CARTESIAN_POINT('Ctrl Pts',(-89.8767453527984,21.9998940815955,0.999999999999998));
#23917=CARTESIAN_POINT('Ctrl Pts',(-89.8186611506175,22.0788444252834,0.999999999999997));
#23918=CARTESIAN_POINT('Ctrl Pts',(-89.7610833542944,22.1571064421111,0.999999999999997));
#23919=CARTESIAN_POINT('Ctrl Pts',(-89.7074121343123,22.2379908576831,0.999999999999994));
#23920=CARTESIAN_POINT('Ctrl Pts',(-89.6579307656577,22.32124888072,0.999999999999994));
#23921=CARTESIAN_POINT('Ctrl Pts',(-89.6098823876189,22.4020957342815,0.999999999999994));
#23922=CARTESIAN_POINT('Ctrl Pts',(-89.5657844916839,22.4851814054866,0.999999999999992));
#23923=CARTESIAN_POINT('Ctrl Pts',(-89.5259442419403,22.5702884173418,0.999999999999991));
#23924=CARTESIAN_POINT('Ctrl Pts',(-89.5051329729808,22.6147455913167,0.999999999999991));
#23925=CARTESIAN_POINT('Ctrl Pts',(-89.4854842991392,22.6597544344945,0.999999999999997));
#23926=CARTESIAN_POINT('Ctrl Pts',(-89.467047707511,22.7052841839688,0.999999999999998));
#23927=CARTESIAN_POINT('Ctrl Pts',(-89.459907033166,22.7229183064012,0.999999999999998));
#23928=CARTESIAN_POINT('Ctrl Pts',(-89.4529482256316,22.7406305682224,0.999999999999992));
#23929=CARTESIAN_POINT('Ctrl Pts',(-89.4461743286839,22.7584191729874,0.999999999999992));
#23930=CARTESIAN_POINT('Ctrl Pts',(-89.4410204433374,22.7719535432535,0.999999999999992));
#23931=CARTESIAN_POINT('Ctrl Pts',(-89.4359736405729,22.7855322273038,0.999999999999996));
#23932=CARTESIAN_POINT('Ctrl Pts',(-89.4310400913489,22.7991405298987,0.999999999999996));
#23933=CARTESIAN_POINT('Ctrl Pts',(-89.3993682456114,22.886501583972,0.999999999999995));
#23934=CARTESIAN_POINT('Ctrl Pts',(-89.3723051104949,22.9752235793332,0.999999999999994));
#23935=CARTESIAN_POINT('Ctrl Pts',(-89.3501019718364,23.0650831124335,0.999999999999994));
#23936=CARTESIAN_POINT('Ctrl Pts',(-89.3450993726547,23.0853294043503,0.999999999999994));
#23937=CARTESIAN_POINT('Ctrl Pts',(-89.3403436950579,23.1056334830589,0.999999999999995));
#23938=CARTESIAN_POINT('Ctrl Pts',(-89.3358381789014,23.1259928495363,0.999999999999995));
#23939=CARTESIAN_POINT('Ctrl Pts',(-89.3154926547755,23.2179294817595,0.999999999999994));
#23940=CARTESIAN_POINT('Ctrl Pts',(-89.3002441342108,23.3109938333353,0.999999999999996));
#23941=CARTESIAN_POINT('Ctrl Pts',(-89.2899827069896,23.4047941591632,0.999999999999996));
#23942=CARTESIAN_POINT('Ctrl Pts',(-89.2792695744502,23.5027235505786,0.999999999999997));
#23943=CARTESIAN_POINT('Ctrl Pts',(-89.2739922714095,23.6014563765805,0.999999999999995));
#23944=CARTESIAN_POINT('Ctrl Pts',(-89.2740832157028,23.7005321536448,0.999999999999995));
#23945=CARTESIAN_POINT('Ctrl Pts',(-89.2741183389869,23.7387958702845,0.999999999999995));
#23946=CARTESIAN_POINT('Ctrl Pts',(-89.2749547528147,23.7771104872619,0.999999999999996));
#23947=CARTESIAN_POINT('Ctrl Pts',(-89.2765906985078,23.8154482999531,0.999999999999996));
#23948=CARTESIAN_POINT('Ctrl Pts',(-89.2771783035686,23.8292186181587,0.999999999999996));
#23949=CARTESIAN_POINT('Ctrl Pts',(-89.2778690508017,23.8429901308395,0.999999999999995));
#23950=CARTESIAN_POINT('Ctrl Pts',(-89.2786619686985,23.8567498857267,0.999999999999995));
#23951=CARTESIAN_POINT('Ctrl Pts',(-89.2840135874435,23.9496182173429,0.999999999999995));
#23952=CARTESIAN_POINT('Ctrl Pts',(-89.2940209180062,24.0420994637446,0.999999999999996));
#23953=CARTESIAN_POINT('Ctrl Pts',(-89.3085609026807,24.1338217237738,0.999999999999996));
#23954=CARTESIAN_POINT('Ctrl Pts',(-89.3230638385443,24.2253102696181,0.999999999999996));
#23955=CARTESIAN_POINT('Ctrl Pts',(-89.3420767704053,24.3160446363436,0.999999999999993));
#23956=CARTESIAN_POINT('Ctrl Pts',(-89.365526168021,24.4056386468464,0.999999999999993));
#23957=CARTESIAN_POINT('Ctrl Pts',(-89.3885742626434,24.4936993836513,0.999999999999993));
#23958=CARTESIAN_POINT('Ctrl Pts',(-89.4159087427651,24.5806592446879,0.999999999999998));
#23959=CARTESIAN_POINT('Ctrl Pts',(-89.447500123989,24.6661223199297,0.999999999999999));
#23960=CARTESIAN_POINT('Ctrl Pts',(-89.463362608983,24.7090345540909,0.999999999999999));
#23961=CARTESIAN_POINT('Ctrl Pts',(-89.4802989345948,24.7515688848954,0.999999999999997));
#23962=CARTESIAN_POINT('Ctrl Pts',(-89.4983087570542,24.7936714134035,0.999999999999997));
#23963=CARTESIAN_POINT('Ctrl Pts',(-89.5036080710629,24.8060599041634,0.999999999999997));
#23964=CARTESIAN_POINT('Ctrl Pts',(-89.5090003430761,24.8184109903508,0.999999999999998));
#23965=CARTESIAN_POINT('Ctrl Pts',(-89.5144855988184,24.8307232500462,0.999999999999998));
#23966=CARTESIAN_POINT('Ctrl Pts',(-89.520079028009,24.8432783169417,0.999999999999998));
#23967=CARTESIAN_POINT('Ctrl Pts',(-89.5257654644254,24.8557847223552,0.999999999999995));
#23968=CARTESIAN_POINT('Ctrl Pts',(-89.5315436189995,24.868239131147,0.999999999999995));
#23969=CARTESIAN_POINT('Ctrl Pts',(-89.5690290042182,24.9490362620044,0.999999999999995));
#23970=CARTESIAN_POINT('Ctrl Pts',(-89.6103840908339,25.0276765323043,0.999999999999998));
#23971=CARTESIAN_POINT('Ctrl Pts',(-89.655539055121,25.1038122347855,0.999999999999997));
#23972=CARTESIAN_POINT('Ctrl Pts',(-89.6999358276934,25.1786695516068,0.999999999999997));
#23973=CARTESIAN_POINT('Ctrl Pts',(-89.7480063970585,25.2511063717929,0.999999999999996));
#23974=CARTESIAN_POINT('Ctrl Pts',(-89.7997205985195,25.3207580282558,0.999999999999995));
#23975=CARTESIAN_POINT('Ctrl Pts',(-89.8498548445873,25.3882817100587,0.999999999999994));
#23976=CARTESIAN_POINT('Ctrl Pts',(-89.9034139287439,25.4531882520902,0.999999999999991));
#23977=CARTESIAN_POINT('Ctrl Pts',(-89.9603980590403,25.5151051167182,0.999999999999991));
#23978=CARTESIAN_POINT('Ctrl Pts',(-89.9815871896822,25.5381284484197,0.999999999999991));
#23979=CARTESIAN_POINT('Ctrl Pts',(-90.0032501397509,25.560737964521,0.999999999999995));
#23980=CARTESIAN_POINT('Ctrl Pts',(-90.025387758703,25.5829128445691,0.999999999999995));
#23981=CARTESIAN_POINT('Ctrl Pts',(-90.0442145502047,25.6017713245233,0.999999999999995));
#23982=CARTESIAN_POINT('Ctrl Pts',(-90.0633846686702,25.6203154277105,0.999999999999994));
#23983=CARTESIAN_POINT('Ctrl Pts',(-90.0828883826537,25.638540237813,0.999999999999994));
#23984=CARTESIAN_POINT('Origin',(-92.,24.,12.2084234471775));
#23985=CARTESIAN_POINT('Ctrl Pts',(-95.076766805402,24.0019372679897,9.70842344717746));
#23986=CARTESIAN_POINT('Ctrl Pts',(-95.0777009893786,24.1261018275903,9.70197366100994));
#23987=CARTESIAN_POINT('Ctrl Pts',(-95.0146667615987,25.2631137100916,9.64286281975954));
#23988=CARTESIAN_POINT('Ctrl Pts',(-93.5990316467515,27.2555126958586,9.53109092342626));
#23989=CARTESIAN_POINT('Ctrl Pts',(-90.1476051047097,27.1179530605299,9.37310775817762));
#23990=CARTESIAN_POINT('Ctrl Pts',(-88.3764282219687,24.1527149914234,9.215124592929));
#23991=CARTESIAN_POINT('Ctrl Pts',(-89.8919231533181,21.0487577497888,9.05714142768035));
#23992=CARTESIAN_POINT('Ctrl Pts',(-93.3195311476575,20.6217766146216,8.89915826243173));
#23993=CARTESIAN_POINT('Ctrl Pts',(-94.9608439554881,22.5621019356809,8.78291893559742));
#23994=CARTESIAN_POINT('Ctrl Pts',(-95.0762792831289,23.7866862376245,8.719340663846));
#23995=CARTESIAN_POINT('Ctrl Pts',(-95.0743674416594,23.9973209105276,8.70842344717745));
#23996=CARTESIAN_POINT('Ctrl Pts',(-95.0702888275776,23.9968971804147,9.79157655282255));
#23997=CARTESIAN_POINT('Ctrl Pts',(-95.0652853128242,24.6903808619892,9.75572892504928));
#23998=CARTESIAN_POINT('Ctrl Pts',(-94.4922439119073,26.4123573994234,9.66722024219312));
#23999=CARTESIAN_POINT('Ctrl Pts',(-91.6460838986403,27.6088399383518,9.5260505042541));
#24000=CARTESIAN_POINT('Ctrl Pts',(-88.7843955634606,25.6770749374766,9.36806733900546));
#24001=CARTESIAN_POINT('Ctrl Pts',(-88.8381773234134,22.2228835564639,9.21008417375683));
#24002=CARTESIAN_POINT('Ctrl Pts',(-91.7604241972829,20.3812153351416,9.05210100850819));
#24003=CARTESIAN_POINT('Ctrl Pts',(-94.5324622678489,21.6531111499586,8.91259846819676));
#24004=CARTESIAN_POINT('Ctrl Pts',(-95.0660796534741,23.3404823888654,8.82575698296822));
#24005=CARTESIAN_POINT('Ctrl Pts',(-95.0703857423214,24.0021357609841,8.79157655282255));
#24006=CARTESIAN_POINT('Ctrl Pts',(-90.0865340033349,25.635987203375,10.));
#24007=CARTESIAN_POINT('Ctrl Pts',(-89.5452199193478,25.0028611672492,9.94733894491712));
#24008=CARTESIAN_POINT('Ctrl Pts',(-89.1498718103828,23.1674010535211,9.84201683475136));
#24009=CARTESIAN_POINT('Ctrl Pts',(-91.1420133042202,21.1541928650905,9.68403366950274));
#24010=CARTESIAN_POINT('Ctrl Pts',(-93.9132996010903,21.7281648944129,9.52605050425409));
#24011=CARTESIAN_POINT('Ctrl Pts',(-94.9487151037096,24.3598882319117,9.36806733900547));
#24012=CARTESIAN_POINT('Ctrl Pts',(-93.3097648188374,26.6665863711808,9.21008417375682));
#24013=CARTESIAN_POINT('Ctrl Pts',(-90.4827056616583,26.5539114461962,9.0521010085082));
#24014=CARTESIAN_POINT('Ctrl Pts',(-89.0319368956585,24.1250886581775,8.89411784325956));
#24015=CARTESIAN_POINT('Ctrl Pts',(-90.2732768955517,21.5826411697067,8.73613467801092));
#24016=CARTESIAN_POINT('Ctrl Pts',(-93.0808263101442,21.2329014567463,8.57815151276229));
#24017=CARTESIAN_POINT('Ctrl Pts',(-94.9080231896089,23.3929749996272,8.42016834751365));
#24018=CARTESIAN_POINT('Ctrl Pts',(-94.097546805733,26.1036603137053,8.26218518226502));
#24019=CARTESIAN_POINT('Ctrl Pts',(-91.3845223931578,26.9062444322857,8.10420201701639));
#24020=CARTESIAN_POINT('Ctrl Pts',(-89.2297579033363,25.0727703008244,7.94621885176775));
#24021=CARTESIAN_POINT('Ctrl Pts',(-89.5876971940872,22.2662546152947,7.78823568651911));
#24022=CARTESIAN_POINT('Ctrl Pts',(-92.1336776409025,21.0323062843058,7.63025252127049));
#24023=CARTESIAN_POINT('Ctrl Pts',(-94.5584078194921,22.4901569016088,7.47226935602184));
#24024=CARTESIAN_POINT('Ctrl Pts',(-94.6625748235914,25.317487010502,7.31428619077322));
#24025=CARTESIAN_POINT('Ctrl Pts',(-92.3516955628713,26.9498113013858,7.15630302552458));
#24026=CARTESIAN_POINT('Ctrl Pts',(-89.7218164325105,25.9065561225943,6.99831986027595));
#24027=CARTESIAN_POINT('Ctrl Pts',(-89.1583275522511,23.1339894343907,6.84033669502731));
#24028=CARTESIAN_POINT('Ctrl Pts',(-91.1723325768719,21.146923903354,6.68235352977868));
#24029=CARTESIAN_POINT('Ctrl Pts',(-93.9370602031581,21.7476957660557,6.52437036453004));
#24030=CARTESIAN_POINT('Ctrl Pts',(-94.9448081097382,24.3913844486004,6.36638719928141));
#24031=CARTESIAN_POINT('Ctrl Pts',(-93.2815145478907,26.6800740756702,6.20840403403277));
#24032=CARTESIAN_POINT('Ctrl Pts',(-90.4558435504055,26.5378450403175,6.05042086878414));
#24033=CARTESIAN_POINT('Ctrl Pts',(-89.0307751580049,24.0937039308721,5.8924377035355));
#24034=CARTESIAN_POINT('Ctrl Pts',(-90.2988950433351,21.5645701580227,5.73445453828688));
#24035=CARTESIAN_POINT('Ctrl Pts',(-93.1099751867047,21.244454378182,5.57647137303824));
#24036=CARTESIAN_POINT('Ctrl Pts',(-94.9142699499044,23.4237125300644,5.4184882077896));
#24037=CARTESIAN_POINT('Ctrl Pts',(-94.0752223982648,26.1256830870713,5.26050504254097));
#24038=CARTESIAN_POINT('Ctrl Pts',(-91.3538772995945,26.8995865300145,5.10252187729233));
#24039=CARTESIAN_POINT('Ctrl Pts',(-89.2185875437792,25.0434660210873,4.9445387120437));
#24040=CARTESIAN_POINT('Ctrl Pts',(-89.606133821254,22.2408862153809,4.78655554679506));
#24041=CARTESIAN_POINT('Ctrl Pts',(-92.1649984307826,21.0338826544913,4.62857238154643));
#24042=CARTESIAN_POINT('Ctrl Pts',(-94.5742038315407,22.5172487662402,4.47058921629779));
#24043=CARTESIAN_POINT('Ctrl Pts',(-94.6485184946103,25.3455208558373,4.31260605104916));
#24044=CARTESIAN_POINT('Ctrl Pts',(-92.3205364822007,26.9533596050059,4.15462288580053));
#24045=CARTESIAN_POINT('Ctrl Pts',(-89.7018169423985,25.88240038523,3.99663972055189));
#24046=CARTESIAN_POINT('Ctrl Pts',(-89.1676278725255,23.1040397712239,3.83865655530326));
#24047=CARTESIAN_POINT('Ctrl Pts',(-91.2024970078837,21.1383456544603,3.68067339005462));
#24048=CARTESIAN_POINT('Ctrl Pts',(-93.9607285557694,21.768269726576,3.52269022480599));
#24049=CARTESIAN_POINT('Ctrl Pts',(-94.9405124242392,24.4224492832982,3.36470705955735));
#24050=CARTESIAN_POINT('Ctrl Pts',(-93.253151066984,26.6934530172094,3.20672389430872));
#24051=CARTESIAN_POINT('Ctrl Pts',(-90.4291391049686,26.5214027346518,3.04874072906008));
#24052=CARTESIAN_POINT('Ctrl Pts',(-89.029951212319,24.0623545122336,2.89075756381145));
#24053=CARTESIAN_POINT('Ctrl Pts',(-90.3246997187609,21.5467477993204,2.73277439856281));
#24054=CARTESIAN_POINT('Ctrl Pts',(-93.139001180181,21.2563262409204,2.57479123331418));
#24055=CARTESIAN_POINT('Ctrl Pts',(-94.9201929246499,23.4545070114807,2.41680806806555));
#24056=CARTESIAN_POINT('Ctrl Pts',(-94.0526634178927,26.1474755214497,2.25882490281691));
#24057=CARTESIAN_POINT('Ctrl Pts',(-91.3233115994341,26.8925961815151,2.10084173756828));
#24058=CARTESIAN_POINT('Ctrl Pts',(-89.2077117493852,25.0140624829424,1.94285857231964));
#24059=CARTESIAN_POINT('Ctrl Pts',(-89.6248688237332,22.215680056917,1.78487540707101));
#24060=CARTESIAN_POINT('Ctrl Pts',(-92.1962362281275,21.0358581128856,1.62689224182237));
#24061=CARTESIAN_POINT('Ctrl Pts',(-94.5898449391916,22.5443661358106,1.46890907657374));
#24062=CARTESIAN_POINT('Ctrl Pts',(-94.6338974915196,25.3736900328969,1.3109259113251));
#24063=CARTESIAN_POINT('Ctrl Pts',(-92.2898922274085,26.9559960431297,1.15294274607647));
#24064=CARTESIAN_POINT('Ctrl Pts',(-89.6809482123999,25.85923592523,0.994959580827835));
#24065=CARTESIAN_POINT('Ctrl Pts',(-89.1795852070609,23.0717155076705,0.836976415579201));
#24066=CARTESIAN_POINT('Ctrl Pts',(-90.5450731455404,21.7830508320407,0.731654305413444));
#24067=CARTESIAN_POINT('Ctrl Pts',(-91.3498000020249,21.5679131979649,0.678993250330566));
#24068=CARTESIAN_POINT('Ctrl Pts',(-89.9456684496579,25.7564253212269,10.1070022498898));
#24069=CARTESIAN_POINT('Ctrl Pts',(-89.3645039014938,25.0766898079629,10.0543411948069));
#24070=CARTESIAN_POINT('Ctrl Pts',(-88.9400510525638,23.1061067782159,9.94901908464118));
#24071=CARTESIAN_POINT('Ctrl Pts',(-91.0788500334022,20.9446902147086,9.79103591939254));
#24072=CARTESIAN_POINT('Ctrl Pts',(-94.0541529050566,21.5609169210655,9.63305275414391));
#24073=CARTESIAN_POINT('Ctrl Pts',(-95.1657936336881,24.3863824863894,9.47506958889527));
#24074=CARTESIAN_POINT('Ctrl Pts',(-93.4061870948087,26.8628951460734,9.31708642364664));
#24075=CARTESIAN_POINT('Ctrl Pts',(-90.3710054760088,26.7419253176407,9.159103258398));
#24076=CARTESIAN_POINT('Ctrl Pts',(-88.8134340044285,24.1342974359261,9.00112009314937));
#24077=CARTESIAN_POINT('Ctrl Pts',(-90.1461589814738,21.4046800297341,8.84313692790073));
#24078=CARTESIAN_POINT('Ctrl Pts',(-93.1603945893153,21.0291931760381,8.68515376265211));
#24079=CARTESIAN_POINT('Ctrl Pts',(-95.1221060619588,23.3482870287292,8.52717059740345));
#24080=CARTESIAN_POINT('Ctrl Pts',(-94.2519640217524,26.2585275939992,8.36918743215484));
#24081=CARTESIAN_POINT('Ctrl Pts',(-91.3392121582154,27.120196356066,8.21120426690619));
#24082=CARTESIAN_POINT('Ctrl Pts',(-89.0258182004901,25.1517455126428,8.05322110165757));
#24083=CARTESIAN_POINT('Ctrl Pts',(-89.4101082685543,22.1386197349377,7.89523793640893));
#24084=CARTESIAN_POINT('Ctrl Pts',(-92.1435187224439,20.813830586732,7.73725477116029));
#24085=CARTESIAN_POINT('Ctrl Pts',(-94.7467527049787,22.3790052613962,7.57927160591167));
#24086=CARTESIAN_POINT('Ctrl Pts',(-94.8585882763444,25.4144777788355,7.42128844066302));
#24087=CARTESIAN_POINT('Ctrl Pts',(-92.37758668938,27.1669705312528,7.2633052754144));
#24088=CARTESIAN_POINT('Ctrl Pts',(-89.5541010980484,26.0469129851116,7.10532211016575));
#24089=CARTESIAN_POINT('Ctrl Pts',(-88.9491292892987,23.0702354622651,6.94733894491712));
#24090=CARTESIAN_POINT('Ctrl Pts',(-91.1114013504886,20.936886126494,6.78935577966849));
#24091=CARTESIAN_POINT('Ctrl Pts',(-94.0796627153006,21.5818856165592,6.63137261441985));
#24092=CARTESIAN_POINT('Ctrl Pts',(-95.1615990146061,24.4201973917876,6.47338944917122));
#24093=CARTESIAN_POINT('Ctrl Pts',(-93.3758570952098,26.8773757884902,6.31540628392258));
#24094=CARTESIAN_POINT('Ctrl Pts',(-90.342165829654,26.724676134977,6.15742311867395));
#24095=CARTESIAN_POINT('Ctrl Pts',(-88.8121867419641,24.1006022275375,5.99943995342532));
#24096=CARTESIAN_POINT('Ctrl Pts',(-90.1736630862473,21.3852786661803,5.84145678817668));
#24097=CARTESIAN_POINT('Ctrl Pts',(-93.1916893480828,21.0415966005281,5.68347362292805));
#24098=CARTESIAN_POINT('Ctrl Pts',(-95.1288126962993,23.3812873949059,5.52549045767941));
#24099=CARTESIAN_POINT('Ctrl Pts',(-94.2279961358928,26.2821716400553,5.36750729243078));
#24100=CARTESIAN_POINT('Ctrl Pts',(-91.3063110339307,27.1130483122969,5.20952412718214));
#24101=CARTESIAN_POINT('Ctrl Pts',(-89.013825501322,25.1202839102265,5.05154096193351));
#24102=CARTESIAN_POINT('Ctrl Pts',(-89.429902163474,22.1113837639744,4.89355779668487));
#24103=CARTESIAN_POINT('Ctrl Pts',(-92.1771452864616,20.8155230061493,4.73557463143624));
#24104=CARTESIAN_POINT('Ctrl Pts',(-94.7637115879574,22.4080915751154,4.5775914661876));
#24105=CARTESIAN_POINT('Ctrl Pts',(-94.8434971484341,25.4445754200009,4.41960830093897));
#24106=CARTESIAN_POINT('Ctrl Pts',(-92.3441337392816,27.1707800539146,4.26162513569034));
#24107=CARTESIAN_POINT('Ctrl Pts',(-89.5326292853278,26.0209789504981,4.1036419704417));
#24108=CARTESIAN_POINT('Ctrl Pts',(-88.9591142806189,23.0380809645772,3.94565880519306));
#24109=CARTESIAN_POINT('Ctrl Pts',(-91.1437864268022,20.9276763640107,3.78767563994443));
#24110=CARTESIAN_POINT('Ctrl Pts',(-94.1050734848669,21.6039741910548,3.6296924746958));
#24111=CARTESIAN_POINT('Ctrl Pts',(-95.1569870893007,24.4535491577124,3.47170930944716));
#24112=CARTESIAN_POINT('Ctrl Pts',(-93.3454055513592,26.891739661045,3.31372614419853));
#24113=CARTESIAN_POINT('Ctrl Pts',(-90.3134954561586,26.7070233795331,3.15574297894989));
#24114=CARTESIAN_POINT('Ctrl Pts',(-88.8113021390385,24.0669449271692,2.99775981370126));
#24115=CARTESIAN_POINT('Ctrl Pts',(-90.2013674504565,21.3661442609453,2.83977664845262));
#24116=CARTESIAN_POINT('Ctrl Pts',(-93.2228521773582,21.0543424461441,2.68179348320399));
#24117=CARTESIAN_POINT('Ctrl Pts',(-95.1351717086425,23.4143489046794,2.52381031795536));
#24118=CARTESIAN_POINT('Ctrl Pts',(-94.2037764083394,26.3055683900265,2.36582715270672));
#24119=CARTESIAN_POINT('Ctrl Pts',(-91.2734951478333,27.1055433482708,2.20784398745809));
#24120=CARTESIAN_POINT('Ctrl Pts',(-89.0021490526171,25.0887157421965,2.04986082220945));
#24121=CARTESIAN_POINT('Ctrl Pts',(-89.4500163995022,22.084321978353,1.89187765696082));
#24122=CARTESIAN_POINT('Ctrl Pts',(-92.2106827481989,20.8176438938541,1.73389449171218));
#24123=CARTESIAN_POINT('Ctrl Pts',(-94.7805041627852,22.4372052713963,1.57591132646355));
#24124=CARTESIAN_POINT('Ctrl Pts',(-94.8277997762312,25.4748183557424,1.41792816121491));
#24125=CARTESIAN_POINT('Ctrl Pts',(-92.3112335155169,27.1736105813594,1.25994499596628));
#24126=CARTESIAN_POINT('Ctrl Pts',(-89.5102242410121,25.9961091691131,1.10196183071765));
#24127=CARTESIAN_POINT('Ctrl Pts',(-88.9719518902951,23.0033770531541,0.943978665469011));
#24128=CARTESIAN_POINT('Ctrl Pts',(-90.4379643297735,21.6198434520492,0.838656555303255));
#24129=CARTESIAN_POINT('Ctrl Pts',(-91.301933573839,21.3888678140614,0.785995500220377));
#24130=CARTESIAN_POINT('Ctrl Pts',(-89.8048028959809,25.8768634390788,10.2140044997796));
#24131=CARTESIAN_POINT('Ctrl Pts',(-89.1837878836397,25.1505184486767,10.1613434446967));
#24132=CARTESIAN_POINT('Ctrl Pts',(-88.730230294745,23.0448125029107,10.056021334531));
#24133=CARTESIAN_POINT('Ctrl Pts',(-91.0156867625841,20.7351875643266,9.89803816928236));
#24134=CARTESIAN_POINT('Ctrl Pts',(-94.1950062090231,21.3936689477181,9.74005500403371));
#24135=CARTESIAN_POINT('Ctrl Pts',(-95.3828721636666,24.4128767408671,9.58207183878509));
#24136=CARTESIAN_POINT('Ctrl Pts',(-93.5026093707802,27.059203920966,9.42408867353644));
#24137=CARTESIAN_POINT('Ctrl Pts',(-90.2593052903592,26.9299391890853,9.26610550828783));
#24138=CARTESIAN_POINT('Ctrl Pts',(-88.5949311131987,24.1435062136747,9.10812234303918));
#24139=CARTESIAN_POINT('Ctrl Pts',(-90.0190410673959,21.2267188897615,8.95013917779055));
#24140=CARTESIAN_POINT('Ctrl Pts',(-93.2399628684865,20.8254848953298,8.79215601254191));
#24141=CARTESIAN_POINT('Ctrl Pts',(-95.3361889343087,23.3035990578312,8.63417284729328));
#24142=CARTESIAN_POINT('Ctrl Pts',(-94.406381237772,26.4133948742932,8.47618968204464));
#24143=CARTESIAN_POINT('Ctrl Pts',(-91.2939019232727,27.3341482798463,8.31820651679601));
#24144=CARTESIAN_POINT('Ctrl Pts',(-88.821878497644,25.2307207244612,8.16022335154738));
#24145=CARTESIAN_POINT('Ctrl Pts',(-89.2325193430214,22.0109848545807,8.00224018629873));
#24146=CARTESIAN_POINT('Ctrl Pts',(-92.1533598039853,20.5953548891583,7.84425702105011));
#24147=CARTESIAN_POINT('Ctrl Pts',(-94.9350975904653,22.2678536211836,7.68627385580147));
#24148=CARTESIAN_POINT('Ctrl Pts',(-95.0546017290973,25.5114685471691,7.52829069055284));
#24149=CARTESIAN_POINT('Ctrl Pts',(-92.4034778158887,27.3841297611198,7.3703075253042));
#24150=CARTESIAN_POINT('Ctrl Pts',(-89.3863857635864,26.187269847629,7.21232436005557));
#24151=CARTESIAN_POINT('Ctrl Pts',(-88.7399310263462,23.0064814901395,7.05434119480693));
#24152=CARTESIAN_POINT('Ctrl Pts',(-91.0504701241054,20.726848349634,6.8963580295583));
#24153=CARTESIAN_POINT('Ctrl Pts',(-94.222265227443,21.4160754670626,6.73837486430966));
#24154=CARTESIAN_POINT('Ctrl Pts',(-95.378389919474,24.4490103349749,6.58039169906103));
#24155=CARTESIAN_POINT('Ctrl Pts',(-93.4701996425288,27.0746775013101,6.42240853381239));
#24156=CARTESIAN_POINT('Ctrl Pts',(-90.2284881089026,26.9115072296366,6.26442536856376));
#24157=CARTESIAN_POINT('Ctrl Pts',(-88.5935983259232,24.1075005242028,6.10644220331512));
#24158=CARTESIAN_POINT('Ctrl Pts',(-90.0484311291595,21.2059871743379,5.9484590380665));
#24159=CARTESIAN_POINT('Ctrl Pts',(-93.2734035094609,20.8387388228742,5.79047587281786));
#24160=CARTESIAN_POINT('Ctrl Pts',(-95.3433554426941,23.3388622597475,5.63249270756922));
#24161=CARTESIAN_POINT('Ctrl Pts',(-94.3807698735207,26.4386601930393,5.47450954232059));
#24162=CARTESIAN_POINT('Ctrl Pts',(-91.2587447682671,27.3265100945794,5.31652637707196));
#24163=CARTESIAN_POINT('Ctrl Pts',(-88.8090634588646,25.1971017993658,5.15854321182332));
#24164=CARTESIAN_POINT('Ctrl Pts',(-89.2536705056942,21.9818813125678,5.00056004657468));
#24165=CARTESIAN_POINT('Ctrl Pts',(-92.1892921421405,20.5971633578073,4.84257688132605));
#24166=CARTESIAN_POINT('Ctrl Pts',(-94.953219344374,22.2989343839906,4.68459371607741));
#24167=CARTESIAN_POINT('Ctrl Pts',(-95.0384758022577,25.5436299841645,4.52661055082878));
#24168=CARTESIAN_POINT('Ctrl Pts',(-92.3677309963625,27.3882005028234,4.36862738558015));
#24169=CARTESIAN_POINT('Ctrl Pts',(-89.3634416282571,26.1595575157663,4.21064422033151));
#24170=CARTESIAN_POINT('Ctrl Pts',(-88.7506006887122,22.9721221579304,4.05266105508288));
#24171=CARTESIAN_POINT('Ctrl Pts',(-91.085075845721,20.7170070735612,3.89467788983424));
#24172=CARTESIAN_POINT('Ctrl Pts',(-94.2494184139642,21.4396786555336,3.73669472458561));
#24173=CARTESIAN_POINT('Ctrl Pts',(-95.3734617543622,24.4846490321267,3.57871155933697));
#24174=CARTESIAN_POINT('Ctrl Pts',(-93.4376600357343,27.0900263048807,3.42072839408834));
#24175=CARTESIAN_POINT('Ctrl Pts',(-90.1978518073486,26.8926440244145,3.26274522883971));
#24176=CARTESIAN_POINT('Ctrl Pts',(-88.5926530657581,24.071535342105,3.10476206359107));
#24177=CARTESIAN_POINT('Ctrl Pts',(-90.0780351821522,21.1855407225702,2.94677889834244));
#24178=CARTESIAN_POINT('Ctrl Pts',(-93.3067031745353,20.8523586513677,2.7887957330938));
#24179=CARTESIAN_POINT('Ctrl Pts',(-95.3501504926354,23.3741907978781,2.63081256784517));
#24180=CARTESIAN_POINT('Ctrl Pts',(-94.354889398786,26.4636612586033,2.47282940259653));
#24181=CARTESIAN_POINT('Ctrl Pts',(-91.2236786962326,27.3184905150265,2.3148462373479));
#24182=CARTESIAN_POINT('Ctrl Pts',(-88.7965863558489,25.1633690014505,2.15686307209926));
#24183=CARTESIAN_POINT('Ctrl Pts',(-89.2751639752712,21.9529638997891,1.99887990685063));
#24184=CARTESIAN_POINT('Ctrl Pts',(-92.2251292682703,20.5994296748226,1.84089674160199));
#24185=CARTESIAN_POINT('Ctrl Pts',(-94.9711633863787,22.3300444069819,1.68291357635336));
#24186=CARTESIAN_POINT('Ctrl Pts',(-95.021702060943,25.5759466785879,1.52493041110472));
#24187=CARTESIAN_POINT('Ctrl Pts',(-92.3325748036253,27.3912251195891,1.36694724585609));
#24188=CARTESIAN_POINT('Ctrl Pts',(-89.3395002696244,26.1329824129964,1.20896408060746));
#24189=CARTESIAN_POINT('Ctrl Pts',(-88.7643185735293,22.9350385986377,1.05098091535882));
#24190=CARTESIAN_POINT('Ctrl Pts',(-90.3308555140066,21.4566360720578,0.945658805193066));
#24191=CARTESIAN_POINT('Ctrl Pts',(-91.2540671456531,21.2098224301578,0.892997750110188));
#24192=CARTESIAN_POINT('Ctrl Pts',(-89.6639373423039,25.9973015569307,10.3210067496694));
#24193=CARTESIAN_POINT('Ctrl Pts',(-89.0030718657857,25.2243470893904,10.2683456945866));
#24194=CARTESIAN_POINT('Ctrl Pts',(-88.520409536926,22.9835182276056,10.1630235844208));
#24195=CARTESIAN_POINT('Ctrl Pts',(-90.9525234917661,20.5256849139446,10.0050404191722));
#24196=CARTESIAN_POINT('Ctrl Pts',(-94.3358595129894,21.2264209743707,9.84705725392353));
#24197=CARTESIAN_POINT('Ctrl Pts',(-95.5999506936451,24.4393709953448,9.6890740886749));
#24198=CARTESIAN_POINT('Ctrl Pts',(-93.5990316467515,27.2555126958586,9.53109092342626));
#24199=CARTESIAN_POINT('Ctrl Pts',(-90.1476051047097,27.1179530605299,9.37310775817762));
#24200=CARTESIAN_POINT('Ctrl Pts',(-88.3764282219687,24.1527149914234,9.215124592929));
#24201=CARTESIAN_POINT('Ctrl Pts',(-89.8919231533181,21.0487577497888,9.05714142768035));
#24202=CARTESIAN_POINT('Ctrl Pts',(-93.3195311476575,20.6217766146216,8.89915826243173));
#24203=CARTESIAN_POINT('Ctrl Pts',(-95.5502718066587,23.2589110869331,8.74117509718308));
#24204=CARTESIAN_POINT('Ctrl Pts',(-94.5607984537914,26.5682621545871,8.58319193193445));
#24205=CARTESIAN_POINT('Ctrl Pts',(-91.2485916883301,27.5481002036266,8.42520876668582));
#24206=CARTESIAN_POINT('Ctrl Pts',(-88.617938794798,25.3096959362796,8.26722560143718));
#24207=CARTESIAN_POINT('Ctrl Pts',(-89.0549304174884,21.8833499742238,8.10924243618856));
#24208=CARTESIAN_POINT('Ctrl Pts',(-92.1632008855268,20.3768791915845,7.95125927093991));
#24209=CARTESIAN_POINT('Ctrl Pts',(-95.1234424759519,22.156701980971,7.79327610569129));
#24210=CARTESIAN_POINT('Ctrl Pts',(-95.2506151818503,25.6084593155026,7.63529294044264));
#24211=CARTESIAN_POINT('Ctrl Pts',(-92.4293689423973,27.6012889909868,7.47730977519402));
#24212=CARTESIAN_POINT('Ctrl Pts',(-89.2186704291244,26.3276267101463,7.31932660994537));
#24213=CARTESIAN_POINT('Ctrl Pts',(-88.5307327633938,22.9427275180138,7.16134344469675));
#24214=CARTESIAN_POINT('Ctrl Pts',(-90.9895388977222,20.516810572774,7.00336027944811));
#24215=CARTESIAN_POINT('Ctrl Pts',(-94.3648677395855,21.250265317566,6.84537711419948));
#24216=CARTESIAN_POINT('Ctrl Pts',(-95.5951808243418,24.4778232781622,6.68739394895084));
#24217=CARTESIAN_POINT('Ctrl Pts',(-93.5645421898479,27.2719792141301,6.5294107837022));
#24218=CARTESIAN_POINT('Ctrl Pts',(-90.1148103881513,27.0983383242962,6.37142761845358));
#24219=CARTESIAN_POINT('Ctrl Pts',(-88.3750099098822,24.1143988208681,6.21344445320493));
#24220=CARTESIAN_POINT('Ctrl Pts',(-89.9231991720716,21.0266956824956,6.05546128795631));
#24221=CARTESIAN_POINT('Ctrl Pts',(-93.355117670839,20.6358810452204,5.89747812270766));
#24222=CARTESIAN_POINT('Ctrl Pts',(-95.5578981890889,23.2964371245891,5.73949495745904));
#24223=CARTESIAN_POINT('Ctrl Pts',(-94.5335436111488,26.5951487460233,5.58151179221039));
#24224=CARTESIAN_POINT('Ctrl Pts',(-91.2111785026033,27.5399718768618,5.42352862696177));
#24225=CARTESIAN_POINT('Ctrl Pts',(-88.6043014164073,25.2739196885051,5.26554546171313));
#24226=CARTESIAN_POINT('Ctrl Pts',(-89.0774388479143,21.8523788611612,5.1075622964645));
#24227=CARTESIAN_POINT('Ctrl Pts',(-92.2014389978195,20.3788037094653,4.94957913121586));
#24228=CARTESIAN_POINT('Ctrl Pts',(-95.1427271007907,22.1897771928657,4.79159596596723));
#24229=CARTESIAN_POINT('Ctrl Pts',(-95.2334544560814,25.6426845483281,4.63361280071859));
#24230=CARTESIAN_POINT('Ctrl Pts',(-92.3913282534434,27.6056209517321,4.47562963546996));
#24231=CARTESIAN_POINT('Ctrl Pts',(-89.1942539711864,26.2981360810345,4.31764647022133));
#24232=CARTESIAN_POINT('Ctrl Pts',(-88.5420870968054,22.9061633512837,4.15966330497268));
#24233=CARTESIAN_POINT('Ctrl Pts',(-91.0263652646397,20.5063377831117,4.00168013972405));
#24234=CARTESIAN_POINT('Ctrl Pts',(-94.3937633430615,21.2753831200124,3.84369697447542));
#24235=CARTESIAN_POINT('Ctrl Pts',(-95.5899364194238,24.515748906541,3.68571380922679));
#24236=CARTESIAN_POINT('Ctrl Pts',(-93.5299145201094,27.2883129487163,3.52773064397815));
#24237=CARTESIAN_POINT('Ctrl Pts',(-90.0822081585387,27.0782646692958,3.36974747872952));
#24238=CARTESIAN_POINT('Ctrl Pts',(-88.3740039924776,24.0761257570407,3.21176431348088));
#24239=CARTESIAN_POINT('Ctrl Pts',(-89.9547029138477,21.0049371841951,3.05378114823225));
#24240=CARTESIAN_POINT('Ctrl Pts',(-93.3905541717124,20.6503748565914,2.89579798298361));
#24241=CARTESIAN_POINT('Ctrl Pts',(-95.5651292766281,23.3340326910768,2.73781481773498));
#24242=CARTESIAN_POINT('Ctrl Pts',(-94.5060023892326,26.6217541271801,2.57983165248634));
#24243=CARTESIAN_POINT('Ctrl Pts',(-91.1738622446318,27.5314376817822,2.42184848723771));
#24244=CARTESIAN_POINT('Ctrl Pts',(-88.5910236590807,25.2380222607046,2.26386532198907));
#24245=CARTESIAN_POINT('Ctrl Pts',(-89.1003115510402,21.8216058212252,2.10588215674044));
#24246=CARTESIAN_POINT('Ctrl Pts',(-92.2395757883417,20.3812154557911,1.94789899149181));
#24247=CARTESIAN_POINT('Ctrl Pts',(-95.1618226099723,22.2228835425676,1.78991582624317));
#24248=CARTESIAN_POINT('Ctrl Pts',(-95.2156043456547,25.6770750014334,1.63193266099454));
#24249=CARTESIAN_POINT('Ctrl Pts',(-92.3539160917337,27.6088396578189,1.4739494957459));
#24250=CARTESIAN_POINT('Ctrl Pts',(-89.1687762982368,26.2698556568796,1.31596633049727));
#24251=CARTESIAN_POINT('Ctrl Pts',(-88.5566852567634,22.8667001441213,1.15798316524863));
#24252=CARTESIAN_POINT('Ctrl Pts',(-90.2237466982397,21.2934286920664,1.05266105508288));
#24253=CARTESIAN_POINT('Ctrl Pts',(-91.2062007174672,21.0307770462543,0.999999999999999));
#24254=CARTESIAN_POINT('Ctrl Pts',(-90.0865340033349,25.635987203375,10.));
#24255=CARTESIAN_POINT('Ctrl Pts',(-90.0249228618548,25.5780878591452,10.));
#24256=CARTESIAN_POINT('Ctrl Pts',(-89.9666808203251,25.517037957366,10.));
#24257=CARTESIAN_POINT('Ctrl Pts',(-89.9118055510373,25.4532222734424,10.));
#24258=CARTESIAN_POINT('Ctrl Pts',(-89.8554775805255,25.3877172106174,10.));
#24259=CARTESIAN_POINT('Ctrl Pts',(-89.8026965604115,25.3192975596955,10.));
#24260=CARTESIAN_POINT('Ctrl Pts',(-89.7534854803736,25.2483309191671,10.));
#24261=CARTESIAN_POINT('Ctrl Pts',(-89.7029129709014,25.1754009794549,10.));
#24262=CARTESIAN_POINT('Ctrl Pts',(-89.6561101247971,25.0997806200714,10.));
#24263=CARTESIAN_POINT('Ctrl Pts',(-89.6131359910394,25.0218257865711,10.));
#24264=CARTESIAN_POINT('Ctrl Pts',(-89.5942445812189,24.9875568769186,10.));
#24265=CARTESIAN_POINT('Ctrl Pts',(-89.576093545669,24.9528363378472,10.));
#24266=CARTESIAN_POINT('Ctrl Pts',(-89.5586903184073,24.9176923367854,10.));
#24267=CARTESIAN_POINT('Ctrl Pts',(-89.5487652975608,24.8976497930708,10.));
#24268=CARTESIAN_POINT('Ctrl Pts',(-89.5390835217552,24.8774695021065,10.));
#24269=CARTESIAN_POINT('Ctrl Pts',(-89.5296466035421,24.8571565405449,10.));
#24270=CARTESIAN_POINT('Ctrl Pts',(-89.5211295714255,24.8388236333292,10.));
#24271=CARTESIAN_POINT('Ctrl Pts',(-89.5128096038927,24.8203769113042,10.));
#24272=CARTESIAN_POINT('Ctrl Pts',(-89.5047015810792,24.8018519373589,10.));
#24273=CARTESIAN_POINT('Ctrl Pts',(-89.4681367628098,24.7183097074791,10.));
#24274=CARTESIAN_POINT('Ctrl Pts',(-89.4358322656984,24.6330839820791,10.));
#24275=CARTESIAN_POINT('Ctrl Pts',(-89.4078131930617,24.5465734751462,10.));
#24276=CARTESIAN_POINT('Ctrl Pts',(-89.3793314409182,24.4586344184821,10.));
#24277=CARTESIAN_POINT('Ctrl Pts',(-89.3552773189935,24.3693670436557,10.));
#24278=CARTESIAN_POINT('Ctrl Pts',(-89.3357162704087,24.2791530221529,10.));
#24279=CARTESIAN_POINT('Ctrl Pts',(-89.3167358111661,24.1916166331482,10.));
#24280=CARTESIAN_POINT('Ctrl Pts',(-89.3019855060178,24.1031880412207,10.));
#24281=CARTESIAN_POINT('Ctrl Pts',(-89.2915659618403,24.0141940291817,10.));
#24282=CARTESIAN_POINT('Ctrl Pts',(-89.2872066009748,23.9769604413456,10.));
#24283=CARTESIAN_POINT('Ctrl Pts',(-89.2836058304791,23.9396276882538,10.));
#24284=CARTESIAN_POINT('Ctrl Pts',(-89.2807733396434,23.9022190875751,10.));
#24285=CARTESIAN_POINT('Ctrl Pts',(-89.2790027503762,23.8788349812521,10.));
#24286=CARTESIAN_POINT('Ctrl Pts',(-89.2775323941369,23.855421232113,10.));
#24287=CARTESIAN_POINT('Ctrl Pts',(-89.2763649279049,23.831983503391,10.));
#24288=CARTESIAN_POINT('Ctrl Pts',(-89.2756806561512,23.8182462531842,10.));
#24289=CARTESIAN_POINT('Ctrl Pts',(-89.2751007108949,23.8045053337837,10.));
#24290=CARTESIAN_POINT('Ctrl Pts',(-89.2746256143469,23.7907701196614,10.));
#24291=CARTESIAN_POINT('Ctrl Pts',(-89.2712677542697,23.6936931626774,10.));
#24292=CARTESIAN_POINT('Ctrl Pts',(-89.2731370867512,23.5967807432359,10.));
#24293=CARTESIAN_POINT('Ctrl Pts',(-89.2802984098264,23.5004551183685,10.));
#24294=CARTESIAN_POINT('Ctrl Pts',(-89.2874597329016,23.4041294935012,10.));
#24295=CARTESIAN_POINT('Ctrl Pts',(-89.2999126116991,23.3083896086995,10.));
#24296=CARTESIAN_POINT('Ctrl Pts',(-89.3177747368199,23.2136387821642,10.));
#24297=CARTESIAN_POINT('Ctrl Pts',(-89.3348522432755,23.1230500173402,10.));
#24298=CARTESIAN_POINT('Ctrl Pts',(-89.3568741021772,23.0333643557258,10.));
#24299=CARTESIAN_POINT('Ctrl Pts',(-89.3835656166833,22.944821137573,10.));
#24300=CARTESIAN_POINT('Ctrl Pts',(-89.3925004778798,22.9151817042656,10.));
#24301=CARTESIAN_POINT('Ctrl Pts',(-89.4019590305019,22.8856703233237,10.));
#24302=CARTESIAN_POINT('Ctrl Pts',(-89.4119322462713,22.8562961512496,10.));
#24303=CARTESIAN_POINT('Ctrl Pts',(-89.4184134249044,22.8372070970455,10.));
#24304=CARTESIAN_POINT('Ctrl Pts',(-89.4251119666747,22.8181759907911,10.));
#24305=CARTESIAN_POINT('Ctrl Pts',(-89.4320255302053,22.7992053804625,10.));
#24306=CARTESIAN_POINT('Ctrl Pts',(-89.4386151870788,22.7811235602558,10.));
#24307=CARTESIAN_POINT('Ctrl Pts',(-89.4454019414807,22.7630924900219,10.));
#24308=CARTESIAN_POINT('Ctrl Pts',(-89.4523729733375,22.7451415275117,10.));
#24309=CARTESIAN_POINT('Ctrl Pts',(-89.4862164573599,22.657991859374,10.));
#24310=CARTESIAN_POINT('Ctrl Pts',(-89.5244382857894,22.5726164812725,10.));
#24311=CARTESIAN_POINT('Ctrl Pts',(-89.5667072739698,22.4892490087878,10.));
#24312=CARTESIAN_POINT('Ctrl Pts',(-89.6105455323263,22.4027864518486,10.));
#24313=CARTESIAN_POINT('Ctrl Pts',(-89.6587371595254,22.3184829337952,10.));
#24314=CARTESIAN_POINT('Ctrl Pts',(-89.7109686726718,22.2366020740164,10.));
#24315=CARTESIAN_POINT('Ctrl Pts',(-89.7637886184407,22.1537987563926,10.));
#24316=CARTESIAN_POINT('Ctrl Pts',(-89.8207403974939,22.0734721714026,10.));
#24317=CARTESIAN_POINT('Ctrl Pts',(-89.8815515974396,21.9959097943086,10.));
#24318=CARTESIAN_POINT('Ctrl Pts',(-89.9232140421765,21.9427709275831,10.));
#24319=CARTESIAN_POINT('Ctrl Pts',(-89.9666890946139,21.8909298240417,10.));
#24320=CARTESIAN_POINT('Ctrl Pts',(-90.0119013664328,21.8404859713398,10.));
#24321=CARTESIAN_POINT('Ctrl Pts',(-90.0240086331394,21.8269777543492,10.));
#24322=CARTESIAN_POINT('Ctrl Pts',(-90.0362418078457,21.8135685183995,10.));
#24323=CARTESIAN_POINT('Ctrl Pts',(-90.0485858239554,21.8002746718516,10.));
#24324=CARTESIAN_POINT('Ctrl Pts',(-90.1172467100136,21.7263305620101,10.));
#24325=CARTESIAN_POINT('Ctrl Pts',(-90.1894214870782,21.6558543370425,10.));
#24326=CARTESIAN_POINT('Ctrl Pts',(-90.2647996929718,21.5891358088469,10.));
#24327=CARTESIAN_POINT('Ctrl Pts',(-90.3277046150347,21.5334575956746,10.));
#24328=CARTESIAN_POINT('Ctrl Pts',(-90.3928415834859,21.4803963685471,10.));
#24329=CARTESIAN_POINT('Ctrl Pts',(-90.4600538268301,21.4301343333567,10.));
#24330=CARTESIAN_POINT('Ctrl Pts',(-90.4819361316924,21.4137705114946,10.));
#24331=CARTESIAN_POINT('Ctrl Pts',(-90.5040385613939,21.3977035152968,10.));
#24332=CARTESIAN_POINT('Ctrl Pts',(-90.5263561317875,21.3819400181443,10.));
#24333=CARTESIAN_POINT('Ctrl Pts',(-90.5491248911564,21.3658578341455,10.));
#24334=CARTESIAN_POINT('Ctrl Pts',(-90.5721229921494,21.3500881169477,10.));
#24335=CARTESIAN_POINT('Ctrl Pts',(-90.5953160059198,21.3346571799234,10.));
#24336=CARTESIAN_POINT('Ctrl Pts',(-90.6802613708273,21.2781407396983,10.));
#24337=CARTESIAN_POINT('Ctrl Pts',(-90.7678730040975,21.2261247337397,10.));
#24338=CARTESIAN_POINT('Ctrl Pts',(-90.8578606394009,21.1789172289357,10.));
#24339=CARTESIAN_POINT('Ctrl Pts',(-90.9411343062963,21.1352318713112,10.));
#24340=CARTESIAN_POINT('Ctrl Pts',(-91.026443472184,21.0956640032536,10.));
#24341=CARTESIAN_POINT('Ctrl Pts',(-91.1135855312338,21.060486601523,10.));
#24342=CARTESIAN_POINT('Ctrl Pts',(-91.14360948864,21.0483665664592,10.));
#24343=CARTESIAN_POINT('Ctrl Pts',(-91.1738512261799,21.0367679981665,10.));
#24344=CARTESIAN_POINT('Ctrl Pts',(-91.2042983602307,21.0256873161864,10.));
#24345=CARTESIAN_POINT('Ctrl Pts',(-94.5182105203766,23.9978055611691,8.38741669750802));
#24346=CARTESIAN_POINT('Ctrl Pts',(-94.5197765073294,23.8252749644444,8.39833391417657));
#24347=CARTESIAN_POINT('Ctrl Pts',(-94.5035405383448,23.6530372868482,8.40925113084511));
#24348=CARTESIAN_POINT('Ctrl Pts',(-94.4684109790521,23.4847436281601,8.42016834751366));
#24349=CARTESIAN_POINT('Ctrl Pts',(-94.2989575631206,22.6729504853336,8.47282940259653));
#24350=CARTESIAN_POINT('Ctrl Pts',(-93.6898919366324,21.95292597104,8.52549045767941));
#24351=CARTESIAN_POINT('Ctrl Pts',(-92.9174342209562,21.6512036660532,8.57815151276229));
#24352=CARTESIAN_POINT('Ctrl Pts',(-92.14497650528,21.3494813610665,8.63081256784517));
#24353=CARTESIAN_POINT('Ctrl Pts',(-91.2091267004159,21.4660612653866,8.68347362292805));
#24354=CARTESIAN_POINT('Ctrl Pts',(-90.5343117980016,21.9480924656251,8.73613467801092));
#24355=CARTESIAN_POINT('Ctrl Pts',(-89.8594968955873,22.4301236658636,8.7887957330938));
#24356=CARTESIAN_POINT('Ctrl Pts',(-89.4457168956229,23.2776061620205,8.84145678817668));
#24357=CARTESIAN_POINT('Ctrl Pts',(-89.480621689974,24.1061512081021,8.89411784325956));
#24358=CARTESIAN_POINT('Ctrl Pts',(-89.5155264843251,24.9346962541837,8.94677889834244));
#24359=CARTESIAN_POINT('Ctrl Pts',(-89.9991160729917,25.7443038501899,8.99943995342532));
#24360=CARTESIAN_POINT('Ctrl Pts',(-90.7120873935215,26.1678868023572,9.0521010085082));
#24361=CARTESIAN_POINT('Ctrl Pts',(-91.4250587140513,26.5914697545244,9.10476206359107));
#24362=CARTESIAN_POINT('Ctrl Pts',(-92.3674117664443,26.6290280628526,9.15742311867395));
#24363=CARTESIAN_POINT('Ctrl Pts',(-93.1117466734529,26.2633575271385,9.21008417375683));
#24364=CARTESIAN_POINT('Ctrl Pts',(-93.8560815804615,25.8976869914244,9.2627452288397));
#24365=CARTESIAN_POINT('Ctrl Pts',(-94.4023983420855,25.128787611668,9.31540628392259));
#24366=CARTESIAN_POINT('Ctrl Pts',(-94.502987472461,24.3057173655401,9.36806733900547));
#24367=CARTESIAN_POINT('Ctrl Pts',(-94.5153073620014,24.2049099077324,9.37451712517299));
#24368=CARTESIAN_POINT('Ctrl Pts',(-94.5209410251377,24.1032898490186,9.38096691134051));
#24369=CARTESIAN_POINT('Ctrl Pts',(-94.5201758362126,24.0015868137836,9.38741669750803));
#24370=CARTESIAN_POINT('Ctrl Pts',(-92.7937992825329,21.0307770462543,10.));
#24371=CARTESIAN_POINT('Ctrl Pts',(-93.7762533017603,21.2934286920664,9.94733894491712));
#24372=CARTESIAN_POINT('Ctrl Pts',(-95.443314608871,22.8667010511062,9.84201683475137));
#24373=CARTESIAN_POINT('Ctrl Pts',(-94.8312238178928,26.2698553838415,9.68403366950273));
#24374=CARTESIAN_POINT('Ctrl Pts',(-91.6460838986403,27.6088399383518,9.5260505042541));
#24375=CARTESIAN_POINT('Ctrl Pts',(-88.7843955634606,25.6770749374766,9.36806733900546));
#24376=CARTESIAN_POINT('Ctrl Pts',(-88.8381773234134,22.2228835564639,9.21008417375683));
#24377=CARTESIAN_POINT('Ctrl Pts',(-91.7604241972829,20.3812153351416,9.05210100850819));
#24378=CARTESIAN_POINT('Ctrl Pts',(-94.8996885260907,21.8216057842524,8.89411784325956));
#24379=CARTESIAN_POINT('Ctrl Pts',(-95.4089764216849,25.2380222823144,8.73613467801093));
#24380=CARTESIAN_POINT('Ctrl Pts',(-92.8261377777637,27.5314377737091,8.57815151276228));
#24381=CARTESIAN_POINT('Ctrl Pts',(-89.493997547754,26.6217541894133,8.42016834751367));
#24382=CARTESIAN_POINT('Ctrl Pts',(-88.4348706359932,23.3340326759415,8.26218518226501));
#24383=CARTESIAN_POINT('Ctrl Pts',(-90.6094457936036,20.6503747732117,8.10420201701639));
#24384=CARTESIAN_POINT('Ctrl Pts',(-94.0452971368402,21.0049371106047,7.94621885176775));
#24385=CARTESIAN_POINT('Ctrl Pts',(-95.6259960969404,24.0761257587368,7.78823568651912));
#24386=CARTESIAN_POINT('Ctrl Pts',(-93.9177918888646,27.0782647453892,7.63025252127048));
#24387=CARTESIAN_POINT('Ctrl Pts',(-90.4700854420894,27.288313029852,7.47226935602185));
#24388=CARTESIAN_POINT('Ctrl Pts',(-88.4100634919605,24.5157489192992,7.31428619077322));
#24389=CARTESIAN_POINT('Ctrl Pts',(-89.6062365978313,21.275383052732,7.15630302552458));
#24390=CARTESIAN_POINT('Ctrl Pts',(-92.9736347594024,20.5063376968639,6.99831986027594));
#24391=CARTESIAN_POINT('Ctrl Pts',(-95.4579129885642,22.9061633242749,6.84033669502732));
#24392=CARTESIAN_POINT('Ctrl Pts',(-94.8057460980851,26.2981361377744,6.68235352977867));
#24393=CARTESIAN_POINT('Ctrl Pts',(-91.6086717368946,27.6056210407497,6.52437036453005));
#24394=CARTESIAN_POINT('Ctrl Pts',(-88.7665454640887,25.6426845888844,6.3663871992814));
#24395=CARTESIAN_POINT('Ctrl Pts',(-88.8572728216189,22.1897771481732,6.20840403403277));
#24396=CARTESIAN_POINT('Ctrl Pts',(-91.7985609972073,20.3788036200624,6.05042086878414));
#24397=CARTESIAN_POINT('Ctrl Pts',(-94.9225612242403,21.852378808139,5.8924377035355));
#24398=CARTESIAN_POINT('Ctrl Pts',(-95.3956986674282,25.2739197199567,5.73445453828687));
#24399=CARTESIAN_POINT('Ctrl Pts',(-92.7888215168717,27.5399719642595,5.57647137303824));
#24400=CARTESIAN_POINT('Ctrl Pts',(-89.466456326301,26.5951488100944,5.4184882077896));
#24401=CARTESIAN_POINT('Ctrl Pts',(-88.4421017230707,23.2964371072189,5.26050504254096));
#24402=CARTESIAN_POINT('Ctrl Pts',(-90.6448822957048,20.6358809621643,5.10252187729233));
#24403=CARTESIAN_POINT('Ctrl Pts',(-94.0768008792021,21.0266956090883,4.9445387120437));
#24404=CARTESIAN_POINT('Ctrl Pts',(-95.6249901796143,24.1143988236926,4.78655554679506));
#24405=CARTESIAN_POINT('Ctrl Pts',(-93.8851896583918,27.0983384007903,4.62857238154643));
#24406=CARTESIAN_POINT('Ctrl Pts',(-90.4354577715253,27.2719792949116,4.47058921629779));
#24407=CARTESIAN_POINT('Ctrl Pts',(-88.4048190868975,24.4778232899584,4.31260605104916));
#24408=CARTESIAN_POINT('Ctrl Pts',(-89.6351322020287,21.2502652496794,4.15462288580053));
#24409=CARTESIAN_POINT('Ctrl Pts',(-93.0104611272249,20.5168104867762,3.99663972055189));
#24410=CARTESIAN_POINT('Ctrl Pts',(-95.4692673222584,22.9427274919151,3.83865655530326));
#24411=CARTESIAN_POINT('Ctrl Pts',(-94.7813296395429,26.3276267676048,3.68067339005461));
#24412=CARTESIAN_POINT('Ctrl Pts',(-91.5706310470027,27.6012890799135,3.52269022480599));
#24413=CARTESIAN_POINT('Ctrl Pts',(-88.7493847378944,25.6084593551841,3.36470705955735));
#24414=CARTESIAN_POINT('Ctrl Pts',(-88.8765574469373,22.156701935519,3.20672389430872));
#24415=CARTESIAN_POINT('Ctrl Pts',(-91.836799110436,20.3768791020246,3.04874072906008));
#24416=CARTESIAN_POINT('Ctrl Pts',(-94.9450696552403,21.883349922176,2.89075756381145));
#24417=CARTESIAN_POINT('Ctrl Pts',(-95.3820612886587,25.3096959682138,2.73277439856281));
#24418=CARTESIAN_POINT('Ctrl Pts',(-92.7514083303166,27.5481002919865,2.57479123331418));
#24419=CARTESIAN_POINT('Ctrl Pts',(-89.4392014827729,26.568262216555,2.41680806806554));
#24420=CARTESIAN_POINT('Ctrl Pts',(-88.4497281061605,23.25891107134,2.25882490281691));
#24421=CARTESIAN_POINT('Ctrl Pts',(-90.6804688187273,20.6217765261787,2.10084173756828));
#24422=CARTESIAN_POINT('Ctrl Pts',(-94.1080769010003,21.0487576862311,1.94285857231964));
#24423=CARTESIAN_POINT('Ctrl Pts',(-95.6235718625379,24.1527149782027,1.78487540707101));
#24424=CARTESIAN_POINT('Ctrl Pts',(-93.8523949517843,27.1179531681002,1.62689224182237));
#24425=CARTESIAN_POINT('Ctrl Pts',(-90.40096829048,27.2555127221398,1.46890907657374));
#24426=CARTESIAN_POINT('Ctrl Pts',(-88.4000492676845,24.4393710995325,1.3109259113251));
#24427=CARTESIAN_POINT('Ctrl Pts',(-89.6641403201721,21.2264207486355,1.15294274607647));
#24428=CARTESIAN_POINT('Ctrl Pts',(-93.0474767585969,20.5256850731752,0.994959580827836));
#24429=CARTESIAN_POINT('Ctrl Pts',(-95.479589838589,22.9835175562679,0.8369764155792));
#24430=CARTESIAN_POINT('Ctrl Pts',(-94.9969281342143,25.2243470893905,0.731654305413444));
#24431=CARTESIAN_POINT('Ctrl Pts',(-94.3360626576961,25.9973015569307,0.678993250330566));
#24432=CARTESIAN_POINT('Ctrl Pts',(-92.7459328543469,21.2098224301578,10.1070022498898));
#24433=CARTESIAN_POINT('Ctrl Pts',(-93.6691444859934,21.4566360720578,10.0543411948069));
#24434=CARTESIAN_POINT('Ctrl Pts',(-95.2356813002075,22.9350394509311,9.94901908464118));
#24435=CARTESIAN_POINT('Ctrl Pts',(-94.6604998395023,26.1329821564226,9.79103591939254));
#24436=CARTESIAN_POINT('Ctrl Pts',(-91.6674251873291,27.3912253832059,9.63305275414391));
#24437=CARTESIAN_POINT('Ctrl Pts',(-88.9782978536527,25.5759466184877,9.47506958889527));
#24438=CARTESIAN_POINT('Ctrl Pts',(-89.0288365510238,22.3300444200403,9.31708642364664));
#24439=CARTESIAN_POINT('Ctrl Pts',(-91.7748707182212,20.5994295614483,9.159103258398));
#24440=CARTESIAN_POINT('Ctrl Pts',(-94.7248360972086,21.9529638650458,9.00112009314937));
#24441=CARTESIAN_POINT('Ctrl Pts',(-95.2034137200466,25.1633690217573,8.84313692790074));
#24442=CARTESIAN_POINT('Ctrl Pts',(-92.7763213248125,27.3184906014102,8.6851537626521));
#24443=CARTESIAN_POINT('Ctrl Pts',(-89.6451105420003,26.4636613170838,8.52717059740347));
#24444=CARTESIAN_POINT('Ctrl Pts',(-88.6498494252551,23.3741907836555,8.36918743215483));
#24445=CARTESIAN_POINT('Ctrl Pts',(-90.6932967928722,20.8523585730158,8.2112042669062));
#24446=CARTESIAN_POINT('Ctrl Pts',(-93.9219648654793,21.1855406534173,8.05322110165756));
#24447=CARTESIAN_POINT('Ctrl Pts',(-95.407347018268,24.0715353436988,7.89523793640893));
#24448=CARTESIAN_POINT('Ctrl Pts',(-93.8021482371961,26.8926440959194,7.73725477116029));
#24449=CARTESIAN_POINT('Ctrl Pts',(-90.562339928744,27.0900263811239,7.57927160591166));
#24450=CARTESIAN_POINT('Ctrl Pts',(-88.6265381623655,24.4846490441156,7.42128844066302));
#24451=CARTESIAN_POINT('Ctrl Pts',(-89.7505815304929,21.4396785923102,7.26330527541439));
#24452=CARTESIAN_POINT('Ctrl Pts',(-92.9149241768713,20.7170069925142,7.10532211016575));
#24453=CARTESIAN_POINT('Ctrl Pts',(-95.2493993915097,22.9721221325502,6.94733894491712));
#24454=CARTESIAN_POINT('Ctrl Pts',(-94.6365584368373,26.1595575690848,6.78935577966849));
#24455=CARTESIAN_POINT('Ctrl Pts',(-91.6322689945581,27.3882005864732,6.63137261441985));
#24456=CARTESIAN_POINT('Ctrl Pts',(-88.9615241227262,25.5436300222753,6.47338944917122));
#24457=CARTESIAN_POINT('Ctrl Pts',(-89.0467805827143,22.298934341993,6.31540628392258));
#24458=CARTESIAN_POINT('Ctrl Pts',(-91.8107078531862,20.5971632737955,6.15742311867395));
#24459=CARTESIAN_POINT('Ctrl Pts',(-94.7463295621093,21.9818812627428,5.99943995342531));
#24460=CARTESIAN_POINT('Ctrl Pts',(-95.1909366199157,25.1971018289209,5.84145678817668));
#24461=CARTESIAN_POINT('Ctrl Pts',(-92.7412552500335,27.3265101767069,5.68347362292804));
#24462=CARTESIAN_POINT('Ctrl Pts',(-89.6192300677009,26.4386602532469,5.52549045767941));
#24463=CARTESIAN_POINT('Ctrl Pts',(-88.6566444747624,23.3388622434248,5.36750729243077));
#24464=CARTESIAN_POINT('Ctrl Pts',(-90.7265964591003,20.8387387448265,5.20952412718215));
#24465=CARTESIAN_POINT('Ctrl Pts',(-93.9515689190225,21.2059871053571,5.05154096193351));
#24466=CARTESIAN_POINT('Ctrl Pts',(-95.4064017581767,24.107500526857,4.89355779668487));
#24467=CARTESIAN_POINT('Ctrl Pts',(-93.7715119348338,26.9115073015181,4.73557463143624));
#24468=CARTESIAN_POINT('Ctrl Pts',(-90.5298003211737,27.0746775772205,4.5775914661876));
#24469=CARTESIAN_POINT('Ctrl Pts',(-88.6216099971176,24.4490103460599,4.41960830093897));
#24470=CARTESIAN_POINT('Ctrl Pts',(-89.777734717692,21.4160754032696,4.26162513569033));
#24471=CARTESIAN_POINT('Ctrl Pts',(-92.9495298993373,20.7268482688219,4.1036419704417));
#24472=CARTESIAN_POINT('Ctrl Pts',(-95.2600690541411,23.0064814656145,3.94565880519306));
#24473=CARTESIAN_POINT('Ctrl Pts',(-94.6136143009402,26.1872699016227,3.78767563994443));
#24474=CARTESIAN_POINT('Ctrl Pts',(-91.5965221741506,27.3841298446842,3.6296924746958));
#24475=CARTESIAN_POINT('Ctrl Pts',(-88.9453981954867,25.5114685844578,3.47170930944717));
#24476=CARTESIAN_POINT('Ctrl Pts',(-89.0649023370739,22.2678535784724,3.31372614419853));
#24477=CARTESIAN_POINT('Ctrl Pts',(-91.8466401922208,20.5953548049989,3.1557429789499));
#24478=CARTESIAN_POINT('Ctrl Pts',(-94.7674807253219,22.0109848056715,2.99775981370126));
#24479=CARTESIAN_POINT('Ctrl Pts',(-95.1781215807801,25.2307207544698,2.83977664845263));
#24480=CARTESIAN_POINT('Ctrl Pts',(-92.7060980942495,27.334148362878,2.68179348320399));
#24481=CARTESIAN_POINT('Ctrl Pts',(-89.5936187026175,26.4133949325244,2.52381031795536));
#24482=CARTESIAN_POINT('Ctrl Pts',(-88.6638109837675,23.3035990431782,2.36582715270672));
#24483=CARTESIAN_POINT('Ctrl Pts',(-90.7600370999255,20.8254848122201,2.20784398745809));
#24484=CARTESIAN_POINT('Ctrl Pts',(-93.9809589836469,21.2267188300363,2.04986082220945));
#24485=CARTESIAN_POINT('Ctrl Pts',(-95.4050689662123,24.1435062012512,1.89187765696082));
#24486=CARTESIAN_POINT('Ctrl Pts',(-93.7406947627281,26.9299392901691,1.73389449171218));
#24487=CARTESIAN_POINT('Ctrl Pts',(-90.4973905702364,27.0592039456624,1.57591132646355));
#24488=CARTESIAN_POINT('Ctrl Pts',(-88.6171277999948,24.4128768387722,1.41792816121492));
#24489=CARTESIAN_POINT('Ctrl Pts',(-89.8049936341991,21.3936687355948,1.25994499596628));
#24490=CARTESIAN_POINT('Ctrl Pts',(-92.9843134726817,20.7351877139554,1.10196183071765));
#24491=CARTESIAN_POINT('Ctrl Pts',(-95.2697691184269,23.044811872055,0.943978665469011));
#24492=CARTESIAN_POINT('Ctrl Pts',(-94.8162121163602,25.1505184486767,0.838656555303255));
#24493=CARTESIAN_POINT('Ctrl Pts',(-94.1951971040191,25.8768634390788,0.785995500220377));
#24494=CARTESIAN_POINT('Ctrl Pts',(-92.698066426161,21.3888678140614,10.2140044997796));
#24495=CARTESIAN_POINT('Ctrl Pts',(-93.5620356702265,21.6198434520493,10.1613434446967));
#24496=CARTESIAN_POINT('Ctrl Pts',(-95.0280479915439,23.0033778507559,10.056021334531));
#24497=CARTESIAN_POINT('Ctrl Pts',(-94.489775861112,25.9961089290038,9.89803816928235));
#24498=CARTESIAN_POINT('Ctrl Pts',(-91.6887664760181,27.1736108280598,9.74005500403372));
#24499=CARTESIAN_POINT('Ctrl Pts',(-89.1722001438447,25.4748182994988,9.58207183878508));
#24500=CARTESIAN_POINT('Ctrl Pts',(-89.2194957786344,22.4372052836166,9.42408867353645));
#24501=CARTESIAN_POINT('Ctrl Pts',(-91.7893172391592,20.8176437877551,9.26610550828781));
#24502=CARTESIAN_POINT('Ctrl Pts',(-94.5499836683268,22.0843219458392,9.10812234303918));
#24503=CARTESIAN_POINT('Ctrl Pts',(-94.9978510184081,25.0887157612002,8.95013917779056));
#24504=CARTESIAN_POINT('Ctrl Pts',(-92.7265048718613,27.1055434291113,8.7921560125419));
#24505=CARTESIAN_POINT('Ctrl Pts',(-89.7962235362468,26.3055684447544,8.63417284729328));
#24506=CARTESIAN_POINT('Ctrl Pts',(-88.8648282145167,23.4143488913694,8.47618968204464));
#24507=CARTESIAN_POINT('Ctrl Pts',(-90.7771477921409,21.05434237282,8.31820651679601));
#24508=CARTESIAN_POINT('Ctrl Pts',(-93.7986325941184,21.36614419623,8.16022335154737));
#24509=CARTESIAN_POINT('Ctrl Pts',(-95.1886979395956,24.0669449286608,8.00224018629874));
#24510=CARTESIAN_POINT('Ctrl Pts',(-93.6865045855277,26.7070234464496,7.84425702105011));
#24511=CARTESIAN_POINT('Ctrl Pts',(-90.6545944153985,26.8917397323958,7.68627385580146));
#24512=CARTESIAN_POINT('Ctrl Pts',(-88.8430128327707,24.453549168932,7.52829069055284));
#24513=CARTESIAN_POINT('Ctrl Pts',(-89.8949264631544,21.6039741318885,7.3703075253042));
#24514=CARTESIAN_POINT('Ctrl Pts',(-92.8562135943403,20.9276762881645,7.21232436005557));
#24515=CARTESIAN_POINT('Ctrl Pts',(-95.0408857944551,23.0380809408256,7.05434119480694));
#24516=CARTESIAN_POINT('Ctrl Pts',(-94.4673707755895,26.0209790003952,6.89635802955829));
#24517=CARTESIAN_POINT('Ctrl Pts',(-91.6558662522217,27.1707801321966,6.73837486430967));
#24518=CARTESIAN_POINT('Ctrl Pts',(-89.1565027813635,25.4445754556661,6.58039169906103));
#24519=CARTESIAN_POINT('Ctrl Pts',(-89.2362883438098,22.4080915358129,6.4224085338124));
#24520=CARTESIAN_POINT('Ctrl Pts',(-91.822854709165,20.8155229275285,6.26442536856376));
#24521=CARTESIAN_POINT('Ctrl Pts',(-94.5700978999785,22.1113837173467,6.10644220331513));
#24522=CARTESIAN_POINT('Ctrl Pts',(-94.9861745724032,25.120283937885,5.94845903806649));
#24523=CARTESIAN_POINT('Ctrl Pts',(-92.6936889831954,27.1130483891544,5.79047587281786));
#24524=CARTESIAN_POINT('Ctrl Pts',(-89.7720038091006,26.2821716963994,5.63249270756922));
#24525=CARTESIAN_POINT('Ctrl Pts',(-88.8711872264539,23.3812873796306,5.47450954232058));
#24526=CARTESIAN_POINT('Ctrl Pts',(-90.8083106224959,21.0415965274887,5.31652637707196));
#24527=CARTESIAN_POINT('Ctrl Pts',(-93.8263369588428,21.385278601626,5.15854321182332));
#24528=CARTESIAN_POINT('Ctrl Pts',(-95.1878133367391,24.1006022300213,5.00056004657468));
#24529=CARTESIAN_POINT('Ctrl Pts',(-93.6578342112759,26.7246762022459,4.84257688132605));
#24530=CARTESIAN_POINT('Ctrl Pts',(-90.6241428708219,26.8773758595294,4.68459371607742));
#24531=CARTESIAN_POINT('Ctrl Pts',(-88.8384009073378,24.4201974021613,4.52661055082877));
#24532=CARTESIAN_POINT('Ctrl Pts',(-89.9203372333551,21.5818855568597,4.36862738558015));
#24533=CARTESIAN_POINT('Ctrl Pts',(-92.8885986714498,20.9368860508676,4.21064422033151));
#24534=CARTESIAN_POINT('Ctrl Pts',(-95.0508707860237,23.0702354393139,4.05266105508288));
#24535=CARTESIAN_POINT('Ctrl Pts',(-94.4458989623375,26.0469130356406,3.89467788983424));
#24536=CARTESIAN_POINT('Ctrl Pts',(-91.6224133012984,27.1669706094549,3.73669472458561));
#24537=CARTESIAN_POINT('Ctrl Pts',(-89.1414116530791,25.4144778137314,3.57871155933698));
#24538=CARTESIAN_POINT('Ctrl Pts',(-89.2532472272103,22.3790052214257,3.42072839408834));
#24539=CARTESIAN_POINT('Ctrl Pts',(-91.8564812740057,20.8138305079731,3.26274522883971));
#24540=CARTESIAN_POINT('Ctrl Pts',(-94.5898917954033,22.1386196891669,3.10476206359107));
#24541=CARTESIAN_POINT('Ctrl Pts',(-94.9741818729016,25.1517455407257,2.94677889834244));
#24542=CARTESIAN_POINT('Ctrl Pts',(-92.6607878581825,27.1201964337696,2.7887957330938));
#24543=CARTESIAN_POINT('Ctrl Pts',(-89.7480359224623,26.2585276484937,2.63081256784517));
#24544=CARTESIAN_POINT('Ctrl Pts',(-88.8778938613744,23.3482870150165,2.47282940259653));
#24545=CARTESIAN_POINT('Ctrl Pts',(-90.8396053811237,21.0291930982615,2.3148462373479));
#24546=CARTESIAN_POINT('Ctrl Pts',(-93.8538410662936,21.4046799738415,2.15686307209927));
#24547=CARTESIAN_POINT('Ctrl Pts',(-95.1865660698866,24.1342974242998,1.99887990685063));
#24548=CARTESIAN_POINT('Ctrl Pts',(-93.628994573672,26.741925412238,1.840896741602));
#24549=CARTESIAN_POINT('Ctrl Pts',(-90.5938128499926,26.862895169185,1.68291357635336));
#24550=CARTESIAN_POINT('Ctrl Pts',(-88.8342063323052,24.386382578012,1.52493041110473));
#24551=CARTESIAN_POINT('Ctrl Pts',(-89.9458469482258,21.5609167225542,1.36694724585609));
#24552=CARTESIAN_POINT('Ctrl Pts',(-92.9211501867667,20.9446903547357,1.20896408060746));
#24553=CARTESIAN_POINT('Ctrl Pts',(-95.0599483982647,23.1061061878421,1.05098091535882));
#24554=CARTESIAN_POINT('Ctrl Pts',(-94.6354960985062,25.076689807963,0.945658805193066));
#24555=CARTESIAN_POINT('Ctrl Pts',(-94.054331550342,25.7564253212269,0.892997750110188));
#24556=CARTESIAN_POINT('Ctrl Pts',(-92.6501999979751,21.5679131979649,10.3210067496694));
#24557=CARTESIAN_POINT('Ctrl Pts',(-93.4549268544596,21.7830508320407,10.2683456945866));
#24558=CARTESIAN_POINT('Ctrl Pts',(-94.8204146828803,23.0717162505807,10.1630235844208));
#24559=CARTESIAN_POINT('Ctrl Pts',(-94.3190518827217,25.8592357015848,10.0050404191722));
#24560=CARTESIAN_POINT('Ctrl Pts',(-91.7101077647069,26.9559962729139,9.84705725392354));
#24561=CARTESIAN_POINT('Ctrl Pts',(-89.3661024340368,25.3736899805099,9.68907408867489));
#24562=CARTESIAN_POINT('Ctrl Pts',(-89.4101550062447,22.544366147193,9.53109092342627));
#24563=CARTESIAN_POINT('Ctrl Pts',(-91.8037637600975,21.0358580140618,9.37310775817762));
#24564=CARTESIAN_POINT('Ctrl Pts',(-94.3751312394447,22.2156800266327,9.215124592929));
#24565=CARTESIAN_POINT('Ctrl Pts',(-94.7922883167697,25.0140625006431,9.05714142768035));
#24566=CARTESIAN_POINT('Ctrl Pts',(-92.6766884189101,26.8925962568123,8.89915826243172));
#24567=CARTESIAN_POINT('Ctrl Pts',(-89.9473365304931,26.1474755724249,8.74117509718309));
#24568=CARTESIAN_POINT('Ctrl Pts',(-89.0798070037785,23.4545069990834,8.58319193193445));
#24569=CARTESIAN_POINT('Ctrl Pts',(-90.8609987914095,21.2563261726241,8.42520876668581));
#24570=CARTESIAN_POINT('Ctrl Pts',(-93.6753003227575,21.5467477390426,8.26722560143719));
#24571=CARTESIAN_POINT('Ctrl Pts',(-94.9700488609232,24.0623545136228,8.10924243618855));
#24572=CARTESIAN_POINT('Ctrl Pts',(-93.5708609338593,26.5214027969798,7.95125927093992));
#24573=CARTESIAN_POINT('Ctrl Pts',(-90.7468489020531,26.6934530836676,7.79327610569128));
#24574=CARTESIAN_POINT('Ctrl Pts',(-89.0594875031757,24.4224492937485,7.63529294044265));
#24575=CARTESIAN_POINT('Ctrl Pts',(-90.0392713958159,21.7682696714666,7.47730977519401));
#24576=CARTESIAN_POINT('Ctrl Pts',(-92.7975030118092,21.1383455838149,7.31932660994537));
#24577=CARTESIAN_POINT('Ctrl Pts',(-94.8323721974005,23.104039749101,7.16134344469675));
#24578=CARTESIAN_POINT('Ctrl Pts',(-94.2981831143417,25.8824004317056,7.0033602794481));
#24579=CARTESIAN_POINT('Ctrl Pts',(-91.6794635098852,26.9533596779201,6.84537711419948));
#24580=CARTESIAN_POINT('Ctrl Pts',(-89.3514814400011,25.3455208890569,6.68739394895083));
#24581=CARTESIAN_POINT('Ctrl Pts',(-89.425796104905,22.5172487296327,6.52941078370221));
#24582=CARTESIAN_POINT('Ctrl Pts',(-91.8350015651438,21.0338825812615,6.37142761845357));
#24583=CARTESIAN_POINT('Ctrl Pts',(-94.3938662378476,22.2408861719505,6.21344445320494));
#24584=CARTESIAN_POINT('Ctrl Pts',(-94.7814125248905,25.0434660468492,6.0554612879563));
#24585=CARTESIAN_POINT('Ctrl Pts',(-92.6461227163573,26.8995866016018,5.89747812270767));
#24586=CARTESIAN_POINT('Ctrl Pts',(-89.9247775505004,26.1256831395519,5.73949495745903));
#24587=CARTESIAN_POINT('Ctrl Pts',(-89.0857299781456,23.4237125158365,5.5815117922104));
#24588=CARTESIAN_POINT('Ctrl Pts',(-90.8900247858914,21.2444543101509,5.42352862696177));
#24589=CARTESIAN_POINT('Ctrl Pts',(-93.7011049986631,21.5645700978948,5.26554546171313));
#24590=CARTESIAN_POINT('Ctrl Pts',(-94.9692249153015,24.0937039331857,5.1075622964645));
#24591=CARTESIAN_POINT('Ctrl Pts',(-93.544156487718,26.5378451029737,4.94957913121586));
#24592=CARTESIAN_POINT('Ctrl Pts',(-90.7184854204702,26.6800741418383,4.79159596596723));
#24593=CARTESIAN_POINT('Ctrl Pts',(-89.0551918175579,24.3913844582627,4.63361280071859));
#24594=CARTESIAN_POINT('Ctrl Pts',(-90.0629397490182,21.7476957104499,4.47562963546996));
#24595=CARTESIAN_POINT('Ctrl Pts',(-92.8276674435623,21.1469238329133,4.31764647022132));
#24596=CARTESIAN_POINT('Ctrl Pts',(-94.8416725179064,23.1339894130133,4.15966330497269));
#24597=CARTESIAN_POINT('Ctrl Pts',(-94.2781836237349,25.9065561696584,4.00168013972405));
#24598=CARTESIAN_POINT('Ctrl Pts',(-91.6483044284461,26.9498113742256,3.84369697447542));
#24599=CARTESIAN_POINT('Ctrl Pts',(-89.3374251106716,25.317487043005,3.68571380922678));
#24600=CARTESIAN_POINT('Ctrl Pts',(-89.4415921173466,22.4901568643791,3.52773064397815));
#24601=CARTESIAN_POINT('Ctrl Pts',(-91.8663223557907,21.0323062109474,3.36974747872952));
#24602=CARTESIAN_POINT('Ctrl Pts',(-94.4123028654849,22.2662545726624,3.21176431348088));
#24603=CARTESIAN_POINT('Ctrl Pts',(-94.770242165023,25.0727703269817,3.05378114823225));
#24604=CARTESIAN_POINT('Ctrl Pts',(-92.6154776221156,26.9062445046611,2.89579798298362));
#24605=CARTESIAN_POINT('Ctrl Pts',(-89.9024531423069,26.103660364463,2.73781481773498));
#24606=CARTESIAN_POINT('Ctrl Pts',(-89.0919767389814,23.3929749868548,2.57983165248635));
#24607=CARTESIAN_POINT('Ctrl Pts',(-90.9191736623217,21.2329013843029,2.42184848723771));
#24608=CARTESIAN_POINT('Ctrl Pts',(-93.7267231489404,21.5826411176466,2.26386532198907));
#24609=CARTESIAN_POINT('Ctrl Pts',(-94.9680631735608,24.1250886473484,2.10588215674044));
#24610=CARTESIAN_POINT('Ctrl Pts',(-93.5172943846158,26.5539115343069,1.94789899149181));
#24611=CARTESIAN_POINT('Ctrl Pts',(-90.690235129749,26.6665863927076,1.78991582624317));
#24612=CARTESIAN_POINT('Ctrl Pts',(-89.0512848646154,24.3598883172517,1.63193266099454));
#24613=CARTESIAN_POINT('Ctrl Pts',(-90.0867002622527,21.7281647095135,1.4739494957459));
#24614=CARTESIAN_POINT('Ctrl Pts',(-92.8579869008516,21.154192995516,1.31596633049727));
#24615=CARTESIAN_POINT('Ctrl Pts',(-94.8501276781025,23.1674005036292,1.15798316524863));
#24616=CARTESIAN_POINT('Ctrl Pts',(-94.4547800806521,25.0028611672492,1.05266105508288));
#24617=CARTESIAN_POINT('Ctrl Pts',(-93.913465996665,25.635987203375,0.999999999999999));
#24618=CARTESIAN_POINT('Ctrl Pts',(-94.5149491154365,24.0017493991467,9.11258330249198));
#24619=CARTESIAN_POINT('Ctrl Pts',(-94.5168561491793,24.2947752403159,9.09410267755477));
#24620=CARTESIAN_POINT('Ctrl Pts',(-94.4695027538977,24.5872051880346,9.07562205261757));
#24621=CARTESIAN_POINT('Ctrl Pts',(-94.3701621542389,24.8607543810029,9.05714142768036));
#24622=CARTESIAN_POINT('Ctrl Pts',(-94.0870883508165,25.6402404193662,9.00448037259748));
#24623=CARTESIAN_POINT('Ctrl Pts',(-93.3818883848633,26.2664183380893,8.9518193175146));
#24624=CARTESIAN_POINT('Ctrl Pts',(-92.5743964204839,26.4553205167196,8.89915826243172));
#24625=CARTESIAN_POINT('Ctrl Pts',(-91.7669044561044,26.6442226953499,8.84649720734884));
#24626=CARTESIAN_POINT('Ctrl Pts',(-90.8571204932987,26.3958491338874,8.79383615226597));
#24627=CARTESIAN_POINT('Ctrl Pts',(-90.2576402574435,25.8228342575992,8.74117509718309));
#24628=CARTESIAN_POINT('Ctrl Pts',(-89.6581600215882,25.2498193813111,8.68851404210021));
#24629=CARTESIAN_POINT('Ctrl Pts',(-89.3689835126833,24.3521631901972,8.63585298701733));
#24630=CARTESIAN_POINT('Ctrl Pts',(-89.5212605561694,23.5369716235638,8.58319193193445));
#24631=CARTESIAN_POINT('Ctrl Pts',(-89.6735375996555,22.7217800569303,8.53053087685158));
#24632=CARTESIAN_POINT('Ctrl Pts',(-90.2672681955325,21.9890531147772,8.47786982176869));
#24633=CARTESIAN_POINT('Ctrl Pts',(-91.0331837486956,21.6710932381038,8.42520876668582));
#24634=CARTESIAN_POINT('Ctrl Pts',(-91.7990993018588,21.3531333614303,8.37254771160294));
#24635=CARTESIAN_POINT('Ctrl Pts',(-92.7371998123082,21.4499405502365,8.31988665652007));
#24636=CARTESIAN_POINT('Ctrl Pts',(-93.4220414905605,21.9176119404029,8.26722560143719));
#24637=CARTESIAN_POINT('Ctrl Pts',(-94.0924008378475,22.375393494611,8.21567816845545));
#24638=CARTESIAN_POINT('Ctrl Pts',(-94.5200994141618,23.1885197854572,8.16413073547371));
#24639=CARTESIAN_POINT('Ctrl Pts',(-94.5215632327497,24.0003195913041,8.11258330249198));
#24640=CARTESIAN_POINT('Ctrl Pts',(-92.7937992825329,21.0307770462543,10.));
#24641=CARTESIAN_POINT('Ctrl Pts',(-92.886852429315,21.0648163030129,10.));
#24642=CARTESIAN_POINT('Ctrl Pts',(-92.9778402996159,21.1036238816581,10.));
#24643=CARTESIAN_POINT('Ctrl Pts',(-93.0665543950992,21.146871551721,10.));
#24644=CARTESIAN_POINT('Ctrl Pts',(-93.1572341761917,21.1910774835146,10.));
#24645=CARTESIAN_POINT('Ctrl Pts',(-93.2455389715861,21.2399230660589,10.));
#24646=CARTESIAN_POINT('Ctrl Pts',(-93.331217194957,21.2931033029543,10.));
#24647=CARTESIAN_POINT('Ctrl Pts',(-93.4136696869558,21.3442813372855,10.));
#24648=CARTESIAN_POINT('Ctrl Pts',(-93.4936899468829,21.399474651453,10.));
#24649=CARTESIAN_POINT('Ctrl Pts',(-93.5710207513935,21.4584414877618,10.));
#24650=CARTESIAN_POINT('Ctrl Pts',(-93.6386852053402,21.510037469532,10.));
#24651=CARTESIAN_POINT('Ctrl Pts',(-93.704290254497,21.5645232522164,10.));
#24652=CARTESIAN_POINT('Ctrl Pts',(-93.7676389322689,21.6217495880709,10.));
#24653=CARTESIAN_POINT('Ctrl Pts',(-93.7817377391777,21.6344858137932,10.));
#24654=CARTESIAN_POINT('Ctrl Pts',(-93.7957273872076,21.6473604850923,10.));
#24655=CARTESIAN_POINT('Ctrl Pts',(-93.8095862319439,21.6603535286729,10.));
#24656=CARTESIAN_POINT('Ctrl Pts',(-93.8820169438681,21.7282592895434,10.));
#24657=CARTESIAN_POINT('Ctrl Pts',(-93.950981982273,21.7994868057952,10.));
#24658=CARTESIAN_POINT('Ctrl Pts',(-94.0162414008102,21.873745473286,10.));
#24659=CARTESIAN_POINT('Ctrl Pts',(-94.0811411486556,21.9475948716335,10.));
#24660=CARTESIAN_POINT('Ctrl Pts',(-94.1423764967312,22.0244428982871,10.));
#24661=CARTESIAN_POINT('Ctrl Pts',(-94.1996678356441,22.1040304952042,10.));
#24662=CARTESIAN_POINT('Ctrl Pts',(-94.2548606489396,22.1807028764161,10.));
#24663=CARTESIAN_POINT('Ctrl Pts',(-94.306393259299,22.2599185451354,10.));
#24664=CARTESIAN_POINT('Ctrl Pts',(-94.3539707411089,22.3414594921653,10.));
#24665=CARTESIAN_POINT('Ctrl Pts',(-94.3739595056304,22.3757173538057,10.));
#24666=CARTESIAN_POINT('Ctrl Pts',(-94.393249578858,22.4103857572211,10.));
#24667=CARTESIAN_POINT('Ctrl Pts',(-94.4118164862111,22.4454488349773,10.));
#24668=CARTESIAN_POINT('Ctrl Pts',(-94.4248530613841,22.4700680373179,10.));
#24669=CARTESIAN_POINT('Ctrl Pts',(-94.4375330822862,22.4948818173567,10.));
#24670=CARTESIAN_POINT('Ctrl Pts',(-94.4498475904497,22.5198846883706,10.));
#24671=CARTESIAN_POINT('Ctrl Pts',(-94.4576000654923,22.5356249949224,10.));
#24672=CARTESIAN_POINT('Ctrl Pts',(-94.4652085569624,22.5514423657842,10.));
#24673=CARTESIAN_POINT('Ctrl Pts',(-94.4726611640941,22.5673143052863,10.));
#24674=CARTESIAN_POINT('Ctrl Pts',(-94.5147817191001,22.6570191413296,10.));
#24675=CARTESIAN_POINT('Ctrl Pts',(-94.5520000635204,22.7486086650705,10.));
#24676=CARTESIAN_POINT('Ctrl Pts',(-94.5840245510179,22.841810410067,10.));
#24677=CARTESIAN_POINT('Ctrl Pts',(-94.6138870174053,22.928719965682,10.));
#24678=CARTESIAN_POINT('Ctrl Pts',(-94.6392330675716,23.0170321958857,10.));
#24679=CARTESIAN_POINT('Ctrl Pts',(-94.6597756784635,23.1065348612349,10.));
#24680=CARTESIAN_POINT('Ctrl Pts',(-94.6612629487322,23.1130147898981,10.));
#24681=CARTESIAN_POINT('Ctrl Pts',(-94.6627250182631,23.1195009595791,10.));
#24682=CARTESIAN_POINT('Ctrl Pts',(-94.6641617673287,23.1259932900522,10.));
#24683=CARTESIAN_POINT('Ctrl Pts',(-94.6847473682253,23.2190147697364,10.));
#24684=CARTESIAN_POINT('Ctrl Pts',(-94.7001391868307,23.3133019772443,10.));
#24685=CARTESIAN_POINT('Ctrl Pts',(-94.710414230246,23.4084468885598,10.));
#24686=CARTESIAN_POINT('Ctrl Pts',(-94.7162318667376,23.4623170753494,10.));
#24687=CARTESIAN_POINT('Ctrl Pts',(-94.7204082723905,23.5164620291754,10.));
#24688=CARTESIAN_POINT('Ctrl Pts',(-94.7229505321312,23.5708049958492,10.));
#24689=CARTESIAN_POINT('Ctrl Pts',(-94.7235978728717,23.5846424553858,10.));
#24690=CARTESIAN_POINT('Ctrl Pts',(-94.7241391083574,23.5984913476866,10.));
#24691=CARTESIAN_POINT('Ctrl Pts',(-94.7245741747776,23.6123381701615,10.));
#24692=CARTESIAN_POINT('Ctrl Pts',(-94.7275029882991,23.7055532725254,10.));
#24693=CARTESIAN_POINT('Ctrl Pts',(-94.7256324130786,23.7988256455609,10.));
#24694=CARTESIAN_POINT('Ctrl Pts',(-94.7190973170423,23.8917800191491,10.));
#24695=CARTESIAN_POINT('Ctrl Pts',(-94.7125517832747,23.9848828576991,10.));
#24696=CARTESIAN_POINT('Ctrl Pts',(-94.7013264378212,24.0776676598214,10.));
#24697=CARTESIAN_POINT('Ctrl Pts',(-94.6855058890551,24.1697452002995,10.));
#24698=CARTESIAN_POINT('Ctrl Pts',(-94.6699125051955,24.2605006130693,10.));
#24699=CARTESIAN_POINT('Ctrl Pts',(-94.6498544727692,24.3505697728504,10.));
#24700=CARTESIAN_POINT('Ctrl Pts',(-94.6253698218263,24.4395547318434,10.));
#24701=CARTESIAN_POINT('Ctrl Pts',(-94.6161277488969,24.4731433454831,10.));
#24702=CARTESIAN_POINT('Ctrl Pts',(-94.6062545684086,24.5065771588648,10.));
#24703=CARTESIAN_POINT('Ctrl Pts',(-94.5957509020197,24.5398334420004,10.));
#24704=CARTESIAN_POINT('Ctrl Pts',(-94.5880549567994,24.564200032081,10.));
#24705=CARTESIAN_POINT('Ctrl Pts',(-94.580020527761,24.5884713017397,10.));
#24706=CARTESIAN_POINT('Ctrl Pts',(-94.5716476124507,24.6126380141342,10.));
#24707=CARTESIAN_POINT('Ctrl Pts',(-94.5664801186889,24.6275529309722,10.));
#24708=CARTESIAN_POINT('Ctrl Pts',(-94.5611866874841,24.6424193347924,10.));
#24709=CARTESIAN_POINT('Ctrl Pts',(-94.5557685057797,24.6572331360837,10.));
#24710=CARTESIAN_POINT('Ctrl Pts',(-94.5240624702071,24.7439203194109,10.));
#24711=CARTESIAN_POINT('Ctrl Pts',(-94.4880796645989,24.8288333308261,10.));
#24712=CARTESIAN_POINT('Ctrl Pts',(-94.4478803904321,24.9115713472888,10.));
#24713=CARTESIAN_POINT('Ctrl Pts',(-94.417730934807,24.9736248596359,10.));
#24714=CARTESIAN_POINT('Ctrl Pts',(-94.385208726487,25.0344544524595,10.));
#24715=CARTESIAN_POINT('Ctrl Pts',(-94.3503241152314,25.0938760326955,10.));
#24716=CARTESIAN_POINT('Ctrl Pts',(-94.3345452312936,25.1207533916281,10.));
#24717=CARTESIAN_POINT('Ctrl Pts',(-94.3182828581177,25.1473424861813,10.));
#24718=CARTESIAN_POINT('Ctrl Pts',(-94.30153717312,25.1736252114009,10.));
#24719=CARTESIAN_POINT('Ctrl Pts',(-94.2924151850668,25.1879423746278,10.));
#24720=CARTESIAN_POINT('Ctrl Pts',(-94.2831549587815,25.2021604667475,10.));
#24721=CARTESIAN_POINT('Ctrl Pts',(-94.2737571738008,25.2162764754097,10.));
#24722=CARTESIAN_POINT('Ctrl Pts',(-94.2261821049897,25.2877369402766,10.));
#24723=CARTESIAN_POINT('Ctrl Pts',(-94.1750818284041,25.3565881459122,10.));
#24724=CARTESIAN_POINT('Ctrl Pts',(-94.1204874011733,25.4224766046402,10.));
#24725=CARTESIAN_POINT('Ctrl Pts',(-94.0743569379003,25.4781501464216,10.));
#24726=CARTESIAN_POINT('Ctrl Pts',(-94.0257310847012,25.5317080232705,10.));
#24727=CARTESIAN_POINT('Ctrl Pts',(-93.974612285206,25.5829128576333,10.));
#24728=CARTESIAN_POINT('Ctrl Pts',(-93.9557804971257,25.6017763403231,10.));
#24729=CARTESIAN_POINT('Ctrl Pts',(-93.9366102390046,25.6203202358367,10.));
#24730=CARTESIAN_POINT('Ctrl Pts',(-93.9171116625783,25.6385402433575,10.));
#24731=CARTESIAN_POINT('Origin',(-92.,24.,5.));
#24732=CARTESIAN_POINT('Origin',(24.,-92.,1.));
#24733=CARTESIAN_POINT('Ctrl Pts',(22.086534003335,-90.364012796625,0.999999999999996));
#24734=CARTESIAN_POINT('Ctrl Pts',(22.0243936079803,-90.4224095095372,0.999999999999996));
#24735=CARTESIAN_POINT('Ctrl Pts',(21.9656285061808,-90.4840599082819,1.));
#24736=CARTESIAN_POINT('Ctrl Pts',(21.9102507399932,-90.5485875659184,1.));
#24737=CARTESIAN_POINT('Ctrl Pts',(21.8535182656837,-90.6146937657734,1.));
#24738=CARTESIAN_POINT('Ctrl Pts',(21.8003404147377,-90.6838202105017,1.));
#24739=CARTESIAN_POINT('Ctrl Pts',(21.7507590223762,-90.7556084413231,1.));
#24740=CARTESIAN_POINT('Ctrl Pts',(21.7378150803192,-90.7743498008507,1.));
#24741=CARTESIAN_POINT('Ctrl Pts',(21.7251164247153,-90.7932727903877,1.));
#24742=CARTESIAN_POINT('Ctrl Pts',(21.712664175894,-90.8123714657101,1.));
#24743=CARTESIAN_POINT('Ctrl Pts',(21.7025035054025,-90.8279554256486,1.));
#24744=CARTESIAN_POINT('Ctrl Pts',(21.6925064617469,-90.8436572537483,1.00000000000001));
#24745=CARTESIAN_POINT('Ctrl Pts',(21.6826824795535,-90.859459161395,1.00000000000001));
#24746=CARTESIAN_POINT('Ctrl Pts',(21.6352350823632,-90.9357784557211,1.00000000000001));
#24747=CARTESIAN_POINT('Ctrl Pts',(21.5917712588655,-91.0145049681213,1.));
#24748=CARTESIAN_POINT('Ctrl Pts',(21.5523257641043,-91.0952462143552,1.));
#24749=CARTESIAN_POINT('Ctrl Pts',(21.5204848603752,-91.1604215725011,1.));
#24750=CARTESIAN_POINT('Ctrl Pts',(21.4912627687126,-91.2269108043057,1.));
#24751=CARTESIAN_POINT('Ctrl Pts',(21.4646949470728,-91.2945252986071,1.));
#24752=CARTESIAN_POINT('Ctrl Pts',(21.453969916315,-91.3218202549228,1.));
#24753=CARTESIAN_POINT('Ctrl Pts',(21.4436776165902,-91.3492987408287,1.));
#24754=CARTESIAN_POINT('Ctrl Pts',(21.4338211709067,-91.3769489152558,1.));
#24755=CARTESIAN_POINT('Ctrl Pts',(21.4286030046016,-91.3915873775532,1.));
#24756=CARTESIAN_POINT('Ctrl Pts',(21.4235075578582,-91.4062726316137,1.));
#24757=CARTESIAN_POINT('Ctrl Pts',(21.4185390502848,-91.4209911044601,1.));
#24758=CARTESIAN_POINT('Ctrl Pts',(21.3890249542532,-91.5084222725943,1.));
#24759=CARTESIAN_POINT('Ctrl Pts',(21.3639471422075,-91.5971333206905,1.00000000000001));
#24760=CARTESIAN_POINT('Ctrl Pts',(21.3433383849555,-91.6867265580416,1.));
#24761=CARTESIAN_POINT('Ctrl Pts',(21.3224107209673,-91.7777061908243,1.));
#24762=CARTESIAN_POINT('Ctrl Pts',(21.3060909929174,-91.8695963327704,1.));
#24763=CARTESIAN_POINT('Ctrl Pts',(21.2944553610685,-91.9620136812046,1.));
#24764=CARTESIAN_POINT('Ctrl Pts',(21.2829108960697,-92.0537069264133,1.));
#24765=CARTESIAN_POINT('Ctrl Pts',(21.2759770698909,-92.1459200787513,1.));
#24766=CARTESIAN_POINT('Ctrl Pts',(21.2737752209329,-92.2382979338272,1.));
#24767=CARTESIAN_POINT('Ctrl Pts',(21.2726800380433,-92.2842459748521,1.));
#24768=CARTESIAN_POINT('Ctrl Pts',(21.2727563056639,-92.3302349753314,1.));
#24769=CARTESIAN_POINT('Ctrl Pts',(21.2740237450673,-92.376221919001,0.999999999999999));
#24770=CARTESIAN_POINT('Ctrl Pts',(21.274440529148,-92.3913442404225,0.999999999999999));
#24771=CARTESIAN_POINT('Ctrl Pts',(21.2749862321654,-92.4064681915453,1.00000000000001));
#24772=CARTESIAN_POINT('Ctrl Pts',(21.2756613706513,-92.4215864144296,1.00000000000001));
#24773=CARTESIAN_POINT('Ctrl Pts',(21.2799353266163,-92.5172921403349,1.00000000000001));
#24774=CARTESIAN_POINT('Ctrl Pts',(21.2893763305713,-92.6124307008699,1.));
#24775=CARTESIAN_POINT('Ctrl Pts',(21.3040485587001,-92.7066037716583,1.));
#24776=CARTESIAN_POINT('Ctrl Pts',(21.3082030637169,-92.7332692850082,1.));
#24777=CARTESIAN_POINT('Ctrl Pts',(21.3127772824124,-92.7598575187067,1.));
#24778=CARTESIAN_POINT('Ctrl Pts',(21.3177733858486,-92.7863596889658,1.));
#24779=CARTESIAN_POINT('Ctrl Pts',(21.3347382842712,-92.8763511457416,1.));
#24780=CARTESIAN_POINT('Ctrl Pts',(21.3565634809548,-92.9653501497144,1.00000000000001));
#24781=CARTESIAN_POINT('Ctrl Pts',(21.3829463368398,-93.053124461382,1.00000000000001));
#24782=CARTESIAN_POINT('Ctrl Pts',(21.4099256760044,-93.1428832401415,1.00000000000001));
#24783=CARTESIAN_POINT('Ctrl Pts',(21.4416712994561,-93.2313620234102,1.));
#24784=CARTESIAN_POINT('Ctrl Pts',(21.4779138149312,-93.3183087529105,1.));
#24785=CARTESIAN_POINT('Ctrl Pts',(21.4905805865845,-93.3486966648463,1.));
#24786=CARTESIAN_POINT('Ctrl Pts',(21.5037971164571,-93.3788973526586,1.));
#24787=CARTESIAN_POINT('Ctrl Pts',(21.5175533367842,-93.4088996997427,1.));
#24788=CARTESIAN_POINT('Ctrl Pts',(21.5245000449418,-93.4240504856619,1.));
#24789=CARTESIAN_POINT('Ctrl Pts',(21.5315843916462,-93.439150688623,1.));
#24790=CARTESIAN_POINT('Ctrl Pts',(21.5388051477107,-93.4541988513293,1.));
#24791=CARTESIAN_POINT('Ctrl Pts',(21.5448146544791,-93.4667227525421,1.));
#24792=CARTESIAN_POINT('Ctrl Pts',(21.5509168026395,-93.4792066765993,1.));
#24793=CARTESIAN_POINT('Ctrl Pts',(21.557106992875,-93.4916425965208,1.));
#24794=CARTESIAN_POINT('Ctrl Pts',(21.6000701102765,-93.5779543037962,1.));
#24795=CARTESIAN_POINT('Ctrl Pts',(21.6473202761047,-93.6620593554308,1.00000000000001));
#24796=CARTESIAN_POINT('Ctrl Pts',(21.6985154201144,-93.7437076709316,1.));
#24797=CARTESIAN_POINT('Ctrl Pts',(21.7507153892901,-93.8269585267468,1.));
#24798=CARTESIAN_POINT('Ctrl Pts',(21.807017032588,-93.9076560355637,1.));
#24799=CARTESIAN_POINT('Ctrl Pts',(21.8671126570016,-93.9855277788831,1.));
#24800=CARTESIAN_POINT('Ctrl Pts',(21.9276763341489,-94.0640060236358,1.));
#24801=CARTESIAN_POINT('Ctrl Pts',(21.9920937838106,-94.1396151518342,1.));
#24802=CARTESIAN_POINT('Ctrl Pts',(22.0600992170831,-94.2120567437253,1.));
#24803=CARTESIAN_POINT('Ctrl Pts',(22.0970259685969,-94.2513923164038,1.));
#24804=CARTESIAN_POINT('Ctrl Pts',(22.1350114303049,-94.2897935419768,1.));
#24805=CARTESIAN_POINT('Ctrl Pts',(22.1740182897571,-94.3272088863493,1.));
#24806=CARTESIAN_POINT('Ctrl Pts',(22.1861457892181,-94.338841572884,1.));
#24807=CARTESIAN_POINT('Ctrl Pts',(22.19837204473,-94.3503789383802,1.));
#24808=CARTESIAN_POINT('Ctrl Pts',(22.2106959996637,-94.3618193694808,1.));
#24809=CARTESIAN_POINT('Ctrl Pts',(22.2219869757007,-94.3723008775767,1.));
#24810=CARTESIAN_POINT('Ctrl Pts',(22.233354235474,-94.3826956656343,1.));
#24811=CARTESIAN_POINT('Ctrl Pts',(22.2447923276406,-94.3929988640766,1.));
#24812=CARTESIAN_POINT('Ctrl Pts',(22.3206014106346,-94.4612861286342,1.));
#24813=CARTESIAN_POINT('Ctrl Pts',(22.3995767828725,-94.525606373815,1.));
#24814=CARTESIAN_POINT('Ctrl Pts',(22.481392277051,-94.5856769718859,1.));
#24815=CARTESIAN_POINT('Ctrl Pts',(22.5632787219117,-94.6457996633891,1.));
#24816=CARTESIAN_POINT('Ctrl Pts',(22.6480107936424,-94.7016661711405,1.));
#24817=CARTESIAN_POINT('Ctrl Pts',(22.7353064390419,-94.7529669283351,1.));
#24818=CARTESIAN_POINT('Ctrl Pts',(22.8208383089763,-94.8032311731532,1.));
#24819=CARTESIAN_POINT('Ctrl Pts',(22.9088318714074,-94.8491129760966,1.));
#24820=CARTESIAN_POINT('Ctrl Pts',(22.999055576298,-94.8902850239913,1.));
#24821=CARTESIAN_POINT('Ctrl Pts',(23.036845885043,-94.9075299864265,1.));
#24822=CARTESIAN_POINT('Ctrl Pts',(23.0750277978348,-94.9239481874739,1.00000000000001));
#24823=CARTESIAN_POINT('Ctrl Pts',(23.1135856932339,-94.9395132002532,1.00000000000001));
#24824=CARTESIAN_POINT('Ctrl Pts',(23.1435994051255,-94.9516291055513,1.00000000000001));
#24825=CARTESIAN_POINT('Ctrl Pts',(23.1738409492154,-94.963228017135,1.));
#24826=CARTESIAN_POINT('Ctrl Pts',(23.2042985533737,-94.9743125149969,1.));
#24827=CARTESIAN_POINT('Ctrl Pts',(24.7937992825328,-94.9692229537457,0.999999999999999));
#24828=CARTESIAN_POINT('Ctrl Pts',(24.8886355742656,-94.9345314145989,0.999999999999998));
#24829=CARTESIAN_POINT('Ctrl Pts',(24.9814286349627,-94.8948494551214,0.999999999999999));
#24830=CARTESIAN_POINT('Ctrl Pts',(25.0719375317936,-94.8504973230204,1.));
#24831=CARTESIAN_POINT('Ctrl Pts',(25.1637179471699,-94.8055221078804,1.));
#24832=CARTESIAN_POINT('Ctrl Pts',(25.2531502379127,-94.7557438784068,1.));
#24833=CARTESIAN_POINT('Ctrl Pts',(25.3399491478545,-94.7014558894208,1.));
#24834=CARTESIAN_POINT('Ctrl Pts',(25.364457897529,-94.6861270018428,1.));
#24835=CARTESIAN_POINT('Ctrl Pts',(25.3887564517354,-94.67043834813,1.));
#24836=CARTESIAN_POINT('Ctrl Pts',(25.412837792733,-94.6543960746657,1.));
#24837=CARTESIAN_POINT('Ctrl Pts',(25.4321685186508,-94.6415185197377,1.));
#24838=CARTESIAN_POINT('Ctrl Pts',(25.4513613841745,-94.6284114764054,1.));
#24839=CARTESIAN_POINT('Ctrl Pts',(25.4703934705292,-94.6150918899927,1.));
#24840=CARTESIAN_POINT('Ctrl Pts',(25.5531011015752,-94.5572090379411,1.));
#24841=CARTESIAN_POINT('Ctrl Pts',(25.632853897381,-94.4952643972528,1.));
#24842=CARTESIAN_POINT('Ctrl Pts',(25.7093855024759,-94.4295552060846,1.));
#24843=CARTESIAN_POINT('Ctrl Pts',(25.7683983469888,-94.378887429332,1.));
#24844=CARTESIAN_POINT('Ctrl Pts',(25.8254952962918,-94.3259804090005,1.));
#24845=CARTESIAN_POINT('Ctrl Pts',(25.8805366461498,-94.2709586395016,1.));
#24846=CARTESIAN_POINT('Ctrl Pts',(25.9098567594312,-94.2416489565302,1.));
#24847=CARTESIAN_POINT('Ctrl Pts',(25.9385932961873,-94.2117390404666,1.));
#24848=CARTESIAN_POINT('Ctrl Pts',(25.9667231095721,-94.1812468751386,1.));
#24849=CARTESIAN_POINT('Ctrl Pts',(25.9763570926068,-94.1708038267102,1.));
#24850=CARTESIAN_POINT('Ctrl Pts',(25.9859191110483,-94.1602932638038,1.));
#24851=CARTESIAN_POINT('Ctrl Pts',(25.9954016781335,-94.1497234370175,1.));
#24852=CARTESIAN_POINT('Ctrl Pts',(26.0611941651552,-94.0763872628137,1.));
#24853=CARTESIAN_POINT('Ctrl Pts',(26.1232544023175,-94.0001047398696,0.999999999999999));
#24854=CARTESIAN_POINT('Ctrl Pts',(26.1813385985981,-93.9211542875407,1.));
#24855=CARTESIAN_POINT('Ctrl Pts',(26.2389163893977,-93.842892162577,1.));
#24856=CARTESIAN_POINT('Ctrl Pts',(26.2925876041462,-93.762007641982,1.));
#24857=CARTESIAN_POINT('Ctrl Pts',(26.3420689684564,-93.6787495211355,1.));
#24858=CARTESIAN_POINT('Ctrl Pts',(26.3901173500934,-93.5979025594445,1.));
#24859=CARTESIAN_POINT('Ctrl Pts',(26.4342152491803,-93.5148167861772,1.));
#24860=CARTESIAN_POINT('Ctrl Pts',(26.4740555020368,-93.429709682334,1.));
#24861=CARTESIAN_POINT('Ctrl Pts',(26.4948667676164,-93.3852524710013,1.));
#24862=CARTESIAN_POINT('Ctrl Pts',(26.5145154386263,-93.3402435934832,1.));
#24863=CARTESIAN_POINT('Ctrl Pts',(26.532952028064,-93.2947138132593,1.));
#24864=CARTESIAN_POINT('Ctrl Pts',(26.5400926949078,-93.2770796953468,1.));
#24865=CARTESIAN_POINT('Ctrl Pts',(26.547051495376,-93.2593674387298,1.));
#24866=CARTESIAN_POINT('Ctrl Pts',(26.5538253857067,-93.2415788398828,1.));
#24867=CARTESIAN_POINT('Ctrl Pts',(26.5589792735639,-93.2280444543052,1.));
#24868=CARTESIAN_POINT('Ctrl Pts',(26.5640260787941,-93.2144657552044,1.));
#24869=CARTESIAN_POINT('Ctrl Pts',(26.5689596304255,-93.2008574378807,1.));
#24870=CARTESIAN_POINT('Ctrl Pts',(26.6006314839344,-93.113496310445,1.));
#24871=CARTESIAN_POINT('Ctrl Pts',(26.6276946267098,-93.0247742554061,0.999999999999999));
#24872=CARTESIAN_POINT('Ctrl Pts',(26.6498977732891,-92.9349146801924,0.999999999999999));
#24873=CARTESIAN_POINT('Ctrl Pts',(26.6549003687673,-92.9146684009979,0.999999999999999));
#24874=CARTESIAN_POINT('Ctrl Pts',(26.6596560432156,-92.8943643360308,0.999999999999998));
#24875=CARTESIAN_POINT('Ctrl Pts',(26.6641615567933,-92.8740049843512,0.999999999999998));
#24876=CARTESIAN_POINT('Ctrl Pts',(26.6845070859586,-92.7820683435573,0.999999999999998));
#24877=CARTESIAN_POINT('Ctrl Pts',(26.6997556148125,-92.6890040030942,0.999999999999999));
#24878=CARTESIAN_POINT('Ctrl Pts',(26.7100170529272,-92.595203704688,1.));
#24879=CARTESIAN_POINT('Ctrl Pts',(26.7207301965764,-92.4972743443061,1.));
#24880=CARTESIAN_POINT('Ctrl Pts',(26.7260075138338,-92.3985415671608,0.999999999999998));
#24881=CARTESIAN_POINT('Ctrl Pts',(26.7259165861328,-92.2994658529915,0.999999999999999));
#24882=CARTESIAN_POINT('Ctrl Pts',(26.7258814692617,-92.2612021661132,0.999999999999999));
#24883=CARTESIAN_POINT('Ctrl Pts',(26.7250450624305,-92.222887581006,0.999999999999999));
#24884=CARTESIAN_POINT('Ctrl Pts',(26.7234091242744,-92.1845498020633,0.999999999999999));
#24885=CARTESIAN_POINT('Ctrl Pts',(26.7228215216315,-92.1707794892028,0.999999999999999));
#24886=CARTESIAN_POINT('Ctrl Pts',(26.722130776784,-92.1570079821017,0.999999999999998));
#24887=CARTESIAN_POINT('Ctrl Pts',(26.7213378612372,-92.1432482330244,0.999999999999999));
#24888=CARTESIAN_POINT('Ctrl Pts',(26.7159862604779,-92.050379977503,0.999999999999999));
#24889=CARTESIAN_POINT('Ctrl Pts',(26.7059789499977,-91.9578988173241,0.999999999999997));
#24890=CARTESIAN_POINT('Ctrl Pts',(26.6914389868445,-91.8661766502431,0.999999999999998));
#24891=CARTESIAN_POINT('Ctrl Pts',(26.676936071269,-91.7746881896765,0.999999999999999));
#24892=CARTESIAN_POINT('Ctrl Pts',(26.6579231603966,-91.683953915049,0.999999999999998));
#24893=CARTESIAN_POINT('Ctrl Pts',(26.6344737838481,-91.5943600002269,0.999999999999998));
#24894=CARTESIAN_POINT('Ctrl Pts',(26.6114257043356,-91.5062993360817,0.999999999999999));
#24895=CARTESIAN_POINT('Ctrl Pts',(26.5840912373207,-91.419339551705,0.999999999999997));
#24896=CARTESIAN_POINT('Ctrl Pts',(26.5524998666087,-91.3338765542973,0.999999999999997));
#24897=CARTESIAN_POINT('Ctrl Pts',(26.536637392274,-91.2909643737748,0.999999999999997));
#24898=CARTESIAN_POINT('Ctrl Pts',(26.5197010773947,-91.2484300966479,0.999999999999998));
#24899=CARTESIAN_POINT('Ctrl Pts',(26.5016912656601,-91.2063276214363,0.999999999999997));
#24900=CARTESIAN_POINT('Ctrl Pts',(26.4963919502112,-91.1939391356146,0.999999999999997));
#24901=CARTESIAN_POINT('Ctrl Pts',(26.490999676596,-91.1815880543971,0.999999999999999));
#24902=CARTESIAN_POINT('Ctrl Pts',(26.4855144190875,-91.1692757996963,0.999999999999999));
#24903=CARTESIAN_POINT('Ctrl Pts',(26.4799210003024,-91.1567207652927,0.999999999999999));
#24904=CARTESIAN_POINT('Ctrl Pts',(26.4742345745685,-91.1442143922703,0.999999999999999));
#24905=CARTESIAN_POINT('Ctrl Pts',(26.468456430893,-91.1317600156219,0.999999999999999));
#24906=CARTESIAN_POINT('Ctrl Pts',(26.4309710579662,-91.0509629673911,0.999999999999999));
#24907=CARTESIAN_POINT('Ctrl Pts',(26.3896159814395,-90.9723227777881,0.999999999999999));
#24908=CARTESIAN_POINT('Ctrl Pts',(26.3444610244852,-90.8961871512465,0.999999999999998));
#24909=CARTESIAN_POINT('Ctrl Pts',(26.3000642489853,-90.8213298919974,0.999999999999998));
#24910=CARTESIAN_POINT('Ctrl Pts',(26.2519936723523,-90.7488931258933,0.999999999999997));
#24911=CARTESIAN_POINT('Ctrl Pts',(26.2002794587303,-90.6792415175287,0.999999999999997));
#24912=CARTESIAN_POINT('Ctrl Pts',(26.1501451852494,-90.6117178613118,0.999999999999997));
#24913=CARTESIAN_POINT('Ctrl Pts',(26.0965860669473,-90.5468113408745,1.));
#24914=CARTESIAN_POINT('Ctrl Pts',(26.0396018951918,-90.4848944918556,1.));
#24915=CARTESIAN_POINT('Ctrl Pts',(26.0184128483334,-90.4618712737448,1.));
#24916=CARTESIAN_POINT('Ctrl Pts',(25.9967499854721,-90.4392618665325,0.999999999999998));
#24917=CARTESIAN_POINT('Ctrl Pts',(25.9746124571306,-90.4170870902725,0.999999999999998));
#24918=CARTESIAN_POINT('Ctrl Pts',(25.9557856680546,-90.3982286238251,0.999999999999998));
#24919=CARTESIAN_POINT('Ctrl Pts',(25.9366155517544,-90.3796845329471,0.999999999999999));
#24920=CARTESIAN_POINT('Ctrl Pts',(25.9171118396844,-90.3614597340102,0.999999999999999));
#24921=CARTESIAN_POINT('Origin',(24.,-92.,12.2084234471775));
#24922=CARTESIAN_POINT('Ctrl Pts',(20.9232328435277,-91.9980626432727,9.70842344717746));
#24923=CARTESIAN_POINT('Ctrl Pts',(20.9222986726779,-91.8738980500464,9.70197366100994));
#24924=CARTESIAN_POINT('Ctrl Pts',(20.9853330132547,-90.7368858898031,9.64286281975954));
#24925=CARTESIAN_POINT('Ctrl Pts',(22.4009680446668,-88.7444871744531,9.53109092342626));
#24926=CARTESIAN_POINT('Ctrl Pts',(25.8523951731073,-88.8820464105141,9.37310775817762));
#24927=CARTESIAN_POINT('Ctrl Pts',(27.6235721938174,-91.847285073477,9.215124592929));
#24928=CARTESIAN_POINT('Ctrl Pts',(26.1080771138749,-94.9512425629647,9.05714142768035));
#24929=CARTESIAN_POINT('Ctrl Pts',(22.6804686869861,-95.3782238204297,8.89915826243172));
#24930=CARTESIAN_POINT('Ctrl Pts',(21.0391556852518,-93.4378982357329,8.78291893559742));
#24931=CARTESIAN_POINT('Ctrl Pts',(20.9237203439564,-92.2133137839327,8.719340663846));
#24932=CARTESIAN_POINT('Ctrl Pts',(20.925632185667,-92.002679085539,8.70842344717746));
#24933=CARTESIAN_POINT('Ctrl Pts',(20.9297109890477,-92.0031050978172,9.79157655282255));
#24934=CARTESIAN_POINT('Ctrl Pts',(20.9347146650535,-91.3096207752369,9.75572892504928));
#24935=CARTESIAN_POINT('Ctrl Pts',(21.5077566649197,-89.5876413967006,9.66722024219313));
#24936=CARTESIAN_POINT('Ctrl Pts',(24.3539160472627,-88.3911616367202,9.5260505042541));
#24937=CARTESIAN_POINT('Ctrl Pts',(27.2156039267669,-90.322924702785,9.36806733900546));
#24938=CARTESIAN_POINT('Ctrl Pts',(27.1618223030447,-93.7771165220753,9.21008417375683));
#24939=CARTESIAN_POINT('Ctrl Pts',(24.2395757220273,-95.6187839878382,9.0521010085082));
#24940=CARTESIAN_POINT('Ctrl Pts',(21.4675381047453,-94.3468885879088,8.91259846819676));
#24941=CARTESIAN_POINT('Ctrl Pts',(20.9339207778366,-92.6595175431003,8.82575698296822));
#24942=CARTESIAN_POINT('Ctrl Pts',(20.9296146841086,-91.99786424691,8.79157655282255));
#24943=CARTESIAN_POINT('Ctrl Pts',(25.913465996665,-90.364012796625,10.));
#24944=CARTESIAN_POINT('Ctrl Pts',(26.4547800806522,-90.9971388327508,9.94733894491712));
#24945=CARTESIAN_POINT('Ctrl Pts',(26.8501256748086,-92.8326016501471,9.84201683475137));
#24946=CARTESIAN_POINT('Ctrl Pts',(24.8579877031057,-94.8458064948082,9.68403366950272));
#24947=CARTESIAN_POINT('Ctrl Pts',(22.0866997272543,-94.2718360144008,9.5260505042541));
#24948=CARTESIAN_POINT('Ctrl Pts',(21.0512847401283,-91.6401113487858,9.36806733900546));
#24949=CARTESIAN_POINT('Ctrl Pts',(22.6902349284037,-89.3334135225916,9.21008417375683));
#24950=CARTESIAN_POINT('Ctrl Pts',(25.5172945659013,-89.4460881205366,9.05210100850819));
#24951=CARTESIAN_POINT('Ctrl Pts',(26.9680634449115,-91.8749113949823,8.89411784325956));
#24952=CARTESIAN_POINT('Ctrl Pts',(25.7267233233057,-94.4173590864694,8.73613467801093));
#24953=CARTESIAN_POINT('Ctrl Pts',(22.9191735544127,-94.7670988996037,8.57815151276228));
#24954=CARTESIAN_POINT('Ctrl Pts',(21.0919764590838,-92.6070250632274,8.42016834751366));
#24955=CARTESIAN_POINT('Ctrl Pts',(21.9024529386513,-89.8963394365792,8.26218518226502));
#24956=CARTESIAN_POINT('Ctrl Pts',(24.6154776819786,-89.0937552116682,8.10420201701638));
#24957=CARTESIAN_POINT('Ctrl Pts',(26.7702424329594,-90.9272295704909,7.94621885176776));
#24958=CARTESIAN_POINT('Ctrl Pts',(26.4123030989785,-93.7337455944376,7.78823568651911));
#24959=CARTESIAN_POINT('Ctrl Pts',(23.8663223428292,-94.9676940765812,7.63025252127049));
#24960=CARTESIAN_POINT('Ctrl Pts',(21.441591869785,-93.5098432815441,7.47226935602184));
#24961=CARTESIAN_POINT('Ctrl Pts',(21.3374248530143,-90.6825128295981,7.31428619077321));
#24962=CARTESIAN_POINT('Ctrl Pts',(23.6483043944151,-89.0501883402777,7.15630302552458));
#24963=CARTESIAN_POINT('Ctrl Pts',(26.2781838441901,-90.0934436458725,6.99831986027595));
#24964=CARTESIAN_POINT('Ctrl Pts',(26.8416727928904,-92.8660106707762,6.84033669502731));
#24965=CARTESIAN_POINT('Ctrl Pts',(24.8276675236541,-94.8530764431805,6.68235352977868));
#24966=CARTESIAN_POINT('Ctrl Pts',(22.0629395615723,-94.2523045074984,6.52437036453004));
#24967=CARTESIAN_POINT('Ctrl Pts',(21.055191532594,-91.6086155038653,6.36638719928141));
#24968=CARTESIAN_POINT('Ctrl Pts',(22.7184852964603,-89.3199255988148,6.20840403403277));
#24969=CARTESIAN_POINT('Ctrl Pts',(25.5441566371433,-89.4621546514439,6.05042086878414));
#24970=CARTESIAN_POINT('Ctrl Pts',(26.9692252026282,-91.9062960577465,5.89243770353551));
#24971=CARTESIAN_POINT('Ctrl Pts',(25.7011051632761,-94.4354301377776,5.73445453828687));
#24972=CARTESIAN_POINT('Ctrl Pts',(22.8900246784809,-94.7555459564984,5.57647137303824));
#24973=CARTESIAN_POINT('Ctrl Pts',(21.0857296961368,-92.5762875399299,5.4184882077896));
#24974=CARTESIAN_POINT('Ctrl Pts',(21.9247773496847,-89.8743166547494,5.26050504254097));
#24975=CARTESIAN_POINT('Ctrl Pts',(24.6461227788815,-89.1004131178103,5.10252187729233));
#24976=CARTESIAN_POINT('Ctrl Pts',(26.781412794043,-90.9565338521763,4.9445387120437));
#24977=CARTESIAN_POINT('Ctrl Pts',(26.3938664694978,-93.759113998276,4.78655554679506));
#24978=CARTESIAN_POINT('Ctrl Pts',(23.8350015491774,-94.9661177057642,4.62857238154643));
#24979=CARTESIAN_POINT('Ctrl Pts',(21.4257958558034,-93.4827514138513,4.4705892162978));
#24980=CARTESIAN_POINT('Ctrl Pts',(21.3514811837096,-90.6544789807379,4.31260605104916));
#24981=CARTESIAN_POINT('Ctrl Pts',(23.6794634788655,-89.0466400362912,4.15462288580053));
#24982=CARTESIAN_POINT('Ctrl Pts',(26.2981833367367,-90.1175993861324,3.99663972055189));
#24983=CARTESIAN_POINT('Ctrl Pts',(26.8323724714771,-92.8959603376101,3.83865655530326));
#24984=CARTESIAN_POINT('Ctrl Pts',(24.7975030889958,-94.8616546930815,3.68067339005462));
#24985=CARTESIAN_POINT('Ctrl Pts',(22.0392712060536,-94.231730544535,3.52269022480599));
#24986=CARTESIAN_POINT('Ctrl Pts',(21.059487218677,-91.5775506652918,3.36470705955735));
#24987=CARTESIAN_POINT('Ctrl Pts',(22.7468487806939,-89.3065466558476,3.20672389430872));
#24988=CARTESIAN_POINT('Ctrl Pts',(25.5708610860458,-89.4785969587254,3.04874072906008));
#24989=CARTESIAN_POINT('Ctrl Pts',(26.9700491479982,-91.9376454809303,2.89075756381145));
#24990=CARTESIAN_POINT('Ctrl Pts',(25.6753004854886,-94.4532524972207,2.73277439856281));
#24991=CARTESIAN_POINT('Ctrl Pts',(22.86099868006,-94.7436740950584,2.57479123331418));
#24992=CARTESIAN_POINT('Ctrl Pts',(21.0798067232474,-92.5454930495189,2.41680806806554));
#24993=CARTESIAN_POINT('Ctrl Pts',(21.9473363281977,-89.8525242277567,2.25882490281691));
#24994=CARTESIAN_POINT('Ctrl Pts',(24.6766884907984,-89.1074034480955,2.10084173756828));
#24995=CARTESIAN_POINT('Ctrl Pts',(26.7922885760843,-90.9859374299123,1.94285857231964));
#24996=CARTESIAN_POINT('Ctrl Pts',(26.3751314870431,-93.7843200921868,1.78487540707101));
#24997=CARTESIAN_POINT('Ctrl Pts',(23.8037637139843,-94.96414237307,1.62689224182237));
#24998=CARTESIAN_POINT('Ctrl Pts',(21.4101547923376,-93.4556338085585,1.46890907657374));
#24999=CARTESIAN_POINT('Ctrl Pts',(21.3661021422765,-90.6263102241947,1.3109259113251));
#25000=CARTESIAN_POINT('Ctrl Pts',(23.7101077338689,-89.0440028274616,1.15294274607647));
#25001=CARTESIAN_POINT('Ctrl Pts',(26.3190522551594,-90.1407651728699,0.994959580827836));
#25002=CARTESIAN_POINT('Ctrl Pts',(26.8204142519502,-92.9282808397392,0.836976415579201));
#25003=CARTESIAN_POINT('Ctrl Pts',(25.4549268544596,-94.2169491679593,0.731654305413445));
#25004=CARTESIAN_POINT('Ctrl Pts',(24.6501999979751,-94.4320868020351,0.678993250330566));
#25005=CARTESIAN_POINT('Ctrl Pts',(26.0543315503421,-90.2435746787731,10.1070022498898));
#25006=CARTESIAN_POINT('Ctrl Pts',(26.6354960985062,-90.923310192037,10.0543411948069));
#25007=CARTESIAN_POINT('Ctrl Pts',(27.0599462474923,-92.893896124491,9.94901908464118));
#25008=CARTESIAN_POINT('Ctrl Pts',(24.9211510480811,-95.0553090980671,9.79103591939255));
#25009=CARTESIAN_POINT('Ctrl Pts',(21.945846373842,-94.4390840546534,9.6330527541439));
#25010=CARTESIAN_POINT('Ctrl Pts',(20.8342061986536,-91.6136170634397,9.47506958889528));
#25011=CARTESIAN_POINT('Ctrl Pts',(22.5938126338247,-89.1371047398789,9.31708642364664));
#25012=CARTESIAN_POINT('Ctrl Pts',(25.6289947683033,-89.2580742171957,9.159103258398));
#25013=CARTESIAN_POINT('Ctrl Pts',(27.1865663612134,-91.8657026211473,9.00112009314937));
#25014=CARTESIAN_POINT('Ctrl Pts',(25.8538412534954,-94.5953202453011,8.84313692790073));
#25015=CARTESIAN_POINT('Ctrl Pts',(22.8396052652705,-94.9708072065457,8.6851537626521));
#25016=CARTESIAN_POINT('Ctrl Pts',(20.8778935608714,-92.6517130387526,8.52717059740347));
#25017=CARTESIAN_POINT('Ctrl Pts',(21.7480357038138,-89.7414721379016,8.36918743215483));
#25018=CARTESIAN_POINT('Ctrl Pts',(24.6607879224527,-88.8798032616766,8.21120426690619));
#25019=CARTESIAN_POINT('Ctrl Pts',(26.9741821605629,-90.8482543491991,8.05322110165757));
#25020=CARTESIAN_POINT('Ctrl Pts',(26.5898920460865,-93.8613804902345,7.89523793640892));
#25021=CARTESIAN_POINT('Ctrl Pts',(23.85648126009,-95.1861698007229,7.7372547711603));
#25022=CARTESIAN_POINT('Ctrl Pts',(21.2532469614236,-93.6209949352398,7.57927160591165));
#25023=CARTESIAN_POINT('Ctrl Pts',(21.1414113764537,-90.5855220494931,7.42128844066304));
#25024=CARTESIAN_POINT('Ctrl Pts',(23.6224132647619,-88.8330290840307,7.26330527541438));
#25025=CARTESIAN_POINT('Ctrl Pts',(26.4458991990222,-89.95308676631,7.10532211016576));
#25026=CARTESIAN_POINT('Ctrl Pts',(27.0508710812515,-92.9297646506441,6.94733894491712));
#25027=CARTESIAN_POINT('Ctrl Pts',(24.8885987574379,-95.0631142455517,6.78935577966849));
#25028=CARTESIAN_POINT('Ctrl Pts',(21.9203370321097,-94.4181146771334,6.63137261441986));
#25029=CARTESIAN_POINT('Ctrl Pts',(20.8384006013954,-91.5798025571788,6.47338944917122));
#25030=CARTESIAN_POINT('Ctrl Pts',(22.6241427376826,-89.1226238620309,6.31540628392259));
#25031=CARTESIAN_POINT('Ctrl Pts',(25.6578343717016,-89.2753235340925,6.15742311867394));
#25032=CARTESIAN_POINT('Ctrl Pts',(27.1878136452183,-91.8993977602433,5.99943995342532));
#25033=CARTESIAN_POINT('Ctrl Pts',(25.8263371355742,-94.6147216513961,5.84145678817668));
#25034=CARTESIAN_POINT('Ctrl Pts',(22.8083105071781,-94.9584037587908,5.68347362292805));
#25035=CARTESIAN_POINT('Ctrl Pts',(20.8711869236843,-92.6187126802411,5.52549045767941));
#25036=CARTESIAN_POINT('Ctrl Pts',(21.7720035935013,-89.7178280827588,5.36750729243077));
#25037=CARTESIAN_POINT('Ctrl Pts',(24.6936890503225,-88.8869513096014,5.20952412718214));
#25038=CARTESIAN_POINT('Ctrl Pts',(26.9861748613701,-90.8797159537069,5.05154096193351));
#25039=CARTESIAN_POINT('Ctrl Pts',(26.5700981486823,-93.8886164654116,4.89355779668487));
#25040=CARTESIAN_POINT('Ctrl Pts',(23.8228546920232,-95.1844773806275,4.73557463143624));
#25041=CARTESIAN_POINT('Ctrl Pts',(21.2362880763696,-93.591908618234,4.5775914661876));
#25042=CARTESIAN_POINT('Ctrl Pts',(21.1565025062044,-90.5554244045433,4.41960830093897));
#25043=CARTESIAN_POINT('Ctrl Pts',(23.6558662189184,-88.8292195609754,4.26162513569033));
#25044=CARTESIAN_POINT('Ctrl Pts',(26.4673710143567,-89.9790208040324,4.1036419704417));
#25045=CARTESIAN_POINT('Ctrl Pts',(27.0408860887086,-92.9619191522691,3.94565880519306));
#25046=CARTESIAN_POINT('Ctrl Pts',(24.8562136772092,-95.0723240091164,3.78767563994443));
#25047=CARTESIAN_POINT('Ctrl Pts',(21.8949262594222,-94.3960261000149,3.6296924746958));
#25048=CARTESIAN_POINT('Ctrl Pts',(20.8430125273277,-91.5464507870927,3.47170930944716));
#25049=CARTESIAN_POINT('Ctrl Pts',(22.6545942851051,-89.1082599879432,3.31372614419853));
#25050=CARTESIAN_POINT('Ctrl Pts',(25.686504748918,-89.2929762912711,3.1557429789499));
#25051=CARTESIAN_POINT('Ctrl Pts',(27.1886982478045,-91.9330550654913,2.99775981370126));
#25052=CARTESIAN_POINT('Ctrl Pts',(25.7986327688294,-94.6338560574266,2.83977664845263));
#25053=CARTESIAN_POINT('Ctrl Pts',(22.7771476725941,-94.9456579145687,2.68179348320399));
#25054=CARTESIAN_POINT('Ctrl Pts',(20.8648279133335,-92.585651160811,2.52381031795536));
#25055=CARTESIAN_POINT('Ctrl Pts',(21.7962233190588,-89.6944313407169,2.36582715270672));
#25056=CARTESIAN_POINT('Ctrl Pts',(24.7265049490419,-88.8944562540726,2.20784398745809));
#25057=CARTESIAN_POINT('Ctrl Pts',(26.997851296813,-90.9112841642428,2.04986082220945));
#25058=CARTESIAN_POINT('Ctrl Pts',(26.5499839341528,-93.9156781817274,1.89187765696082));
#25059=CARTESIAN_POINT('Ctrl Pts',(23.7893171896513,-95.1823566278765,1.73389449171218));
#25060=CARTESIAN_POINT('Ctrl Pts',(21.2194955489797,-93.5627946688774,1.57591132646355));
#25061=CARTESIAN_POINT('Ctrl Pts',(21.1721998306057,-90.5251819202757,1.41792816121491));
#25062=CARTESIAN_POINT('Ctrl Pts',(23.6887664429097,-88.826388206087,1.25994499596628));
#25063=CARTESIAN_POINT('Ctrl Pts',(26.4897762609679,-90.0038920098267,1.10196183071765));
#25064=CARTESIAN_POINT('Ctrl Pts',(27.0280475288895,-92.9966190253592,0.943978665469011));
#25065=CARTESIAN_POINT('Ctrl Pts',(25.5620356702265,-94.3801565479507,0.838656555303256));
#25066=CARTESIAN_POINT('Ctrl Pts',(24.698066426161,-94.6111321859386,0.785995500220377));
#25067=CARTESIAN_POINT('Ctrl Pts',(26.1951971040191,-90.1231365609212,10.2140044997796));
#25068=CARTESIAN_POINT('Ctrl Pts',(26.8162121163602,-90.8494815513233,10.1613434446967));
#25069=CARTESIAN_POINT('Ctrl Pts',(27.269766820176,-92.9551905988348,10.056021334531));
#25070=CARTESIAN_POINT('Ctrl Pts',(24.9843143930565,-95.2648117013261,9.89803816928236));
#25071=CARTESIAN_POINT('Ctrl Pts',(21.8049930204297,-94.6063320949058,9.74005500403372));
#25072=CARTESIAN_POINT('Ctrl Pts',(20.6171276571787,-91.5871227780939,9.58207183878508));
#25073=CARTESIAN_POINT('Ctrl Pts',(22.4973903392457,-88.9407959571659,9.42408867353645));
#25074=CARTESIAN_POINT('Ctrl Pts',(25.7406949707053,-89.070060313855,9.26610550828781));
#25075=CARTESIAN_POINT('Ctrl Pts',(27.4050692775154,-91.856493847312,9.10812234303918));
#25076=CARTESIAN_POINT('Ctrl Pts',(25.9809591836852,-94.773281404133,8.95013917779054));
#25077=CARTESIAN_POINT('Ctrl Pts',(22.7600369761283,-95.1745155134876,8.79215601254191));
#25078=CARTESIAN_POINT('Ctrl Pts',(20.663810662659,-92.6964010142779,8.63417284729327));
#25079=CARTESIAN_POINT('Ctrl Pts',(21.5936184689764,-89.5866048392241,8.47618968204464));
#25080=CARTESIAN_POINT('Ctrl Pts',(24.7060981629267,-88.6658513116848,8.31820651679601));
#25081=CARTESIAN_POINT('Ctrl Pts',(27.1781218881664,-90.7692791279071,8.16022335154737));
#25082=CARTESIAN_POINT('Ctrl Pts',(26.7674809931943,-93.9890153860317,8.00224018629874));
#25083=CARTESIAN_POINT('Ctrl Pts',(23.8466401773509,-95.4046455248643,7.84425702105011));
#25084=CARTESIAN_POINT('Ctrl Pts',(21.0649020530622,-93.7321465889358,7.68627385580147));
#25085=CARTESIAN_POINT('Ctrl Pts',(20.945397899893,-90.488531269388,7.52829069055284));
#25086=CARTESIAN_POINT('Ctrl Pts',(23.5965221351088,-88.6158698277836,7.37030752530419));
#25087=CARTESIAN_POINT('Ctrl Pts',(26.6136145538544,-89.8127298867477,7.21232436005558));
#25088=CARTESIAN_POINT('Ctrl Pts',(27.2600693696125,-92.9935186305118,7.05434119480693));
#25089=CARTESIAN_POINT('Ctrl Pts',(24.9495299912216,-95.2731520479227,6.8963580295583));
#25090=CARTESIAN_POINT('Ctrl Pts',(21.7777345026472,-94.5839248467686,6.73837486430966));
#25091=CARTESIAN_POINT('Ctrl Pts',(20.6216096701967,-91.5509896104921,6.58039169906103));
#25092=CARTESIAN_POINT('Ctrl Pts',(22.529800178905,-88.9253221252473,6.42240853381239));
#25093=CARTESIAN_POINT('Ctrl Pts',(25.77151210626,-89.0884924167409,6.26442536856375));
#25094=CARTESIAN_POINT('Ctrl Pts',(27.4064020878083,-91.8924994627401,6.10644220331513));
#25095=CARTESIAN_POINT('Ctrl Pts',(25.9515691078724,-94.7940131650148,5.94845903806649));
#25096=CARTESIAN_POINT('Ctrl Pts',(22.7265963358753,-95.1612615610832,5.79047587281786));
#25097=CARTESIAN_POINT('Ctrl Pts',(20.6566441512317,-92.6611378205523,5.63249270756922));
#25098=CARTESIAN_POINT('Ctrl Pts',(21.6192298373179,-89.5613395107682,5.47450954232059));
#25099=CARTESIAN_POINT('Ctrl Pts',(24.7412553217635,-88.6734895013924,5.31652637707195));
#25100=CARTESIAN_POINT('Ctrl Pts',(27.1909369286972,-90.8028980552376,5.15854321182332));
#25101=CARTESIAN_POINT('Ctrl Pts',(26.7463298278667,-94.0181189325472,5.00056004657468));
#25102=CARTESIAN_POINT('Ctrl Pts',(23.8107078348689,-95.4028370554907,4.84257688132605));
#25103=CARTESIAN_POINT('Ctrl Pts',(21.0467802969359,-93.701065822617,4.68459371607741));
#25104=CARTESIAN_POINT('Ctrl Pts',(20.9615238286993,-90.4563698283487,4.52661055082878));
#25105=CARTESIAN_POINT('Ctrl Pts',(23.6322689589712,-88.6117990856597,4.36862738558015));
#25106=CARTESIAN_POINT('Ctrl Pts',(26.6365586919768,-89.8404422219323,4.21064422033151));
#25107=CARTESIAN_POINT('Ctrl Pts',(27.2493997059402,-93.0278779669281,4.05266105508288));
#25108=CARTESIAN_POINT('Ctrl Pts',(24.9149242654226,-95.2829933251511,3.89467788983424));
#25109=CARTESIAN_POINT('Ctrl Pts',(21.7505813127907,-94.5603216554948,3.73669472458561));
#25110=CARTESIAN_POINT('Ctrl Pts',(20.6265378359784,-91.5153509088937,3.57871155933697));
#25111=CARTESIAN_POINT('Ctrl Pts',(22.5623397895163,-88.9099733200387,3.42072839408834));
#25112=CARTESIAN_POINT('Ctrl Pts',(25.80214841179,-89.1073556238167,3.2627452288397));
#25113=CARTESIAN_POINT('Ctrl Pts',(27.4073473476108,-91.9284646500524,3.10476206359107));
#25114=CARTESIAN_POINT('Ctrl Pts',(25.9219650521703,-94.8144596176324,2.94677889834244));
#25115=CARTESIAN_POINT('Ctrl Pts',(22.6932966651281,-95.1476417340791,2.7887957330938));
#25116=CARTESIAN_POINT('Ctrl Pts',(20.6498491034196,-92.625809272103,2.63081256784516));
#25117=CARTESIAN_POINT('Ctrl Pts',(21.6451103099198,-89.5363384536772,2.47282940259654));
#25118=CARTESIAN_POINT('Ctrl Pts',(24.7763214072854,-88.6815090600494,2.3148462373479));
#25119=CARTESIAN_POINT('Ctrl Pts',(27.2034140175416,-90.8366308985733,2.15686307209927));
#25120=CARTESIAN_POINT('Ctrl Pts',(26.7248363812625,-94.047036271268,1.99887990685063));
#25121=CARTESIAN_POINT('Ctrl Pts',(23.7748706653183,-95.4005708826832,1.840896741602));
#25122=CARTESIAN_POINT('Ctrl Pts',(21.0288363056219,-93.6699555291963,1.68291357635336));
#25123=CARTESIAN_POINT('Ctrl Pts',(20.9782975189348,-90.4240536163567,1.52493041110473));
#25124=CARTESIAN_POINT('Ctrl Pts',(23.6674251519506,-88.6087735847125,1.36694724585609));
#25125=CARTESIAN_POINT('Ctrl Pts',(26.6605002667764,-89.8670188467833,1.20896408060746));
#25126=CARTESIAN_POINT('Ctrl Pts',(27.2356808058288,-93.0649572109792,1.05098091535882));
#25127=CARTESIAN_POINT('Ctrl Pts',(25.6691444859934,-94.5433639279422,0.945658805193066));
#25128=CARTESIAN_POINT('Ctrl Pts',(24.7459328543469,-94.7901775698421,0.892997750110188));
#25129=CARTESIAN_POINT('Ctrl Pts',(26.3360626576961,-90.0026984430693,10.3210067496694));
#25130=CARTESIAN_POINT('Ctrl Pts',(26.9969281342143,-90.7756529106096,10.2683456945866));
#25131=CARTESIAN_POINT('Ctrl Pts',(27.4795873928596,-93.0164850731786,10.1630235844208));
#25132=CARTESIAN_POINT('Ctrl Pts',(25.0474777380319,-95.4743143045851,10.0050404191722));
#25133=CARTESIAN_POINT('Ctrl Pts',(21.6641396670173,-94.7735801351584,9.84705725392352));
#25134=CARTESIAN_POINT('Ctrl Pts',(20.4000491157039,-91.5606284927479,9.6890740886749));
#25135=CARTESIAN_POINT('Ctrl Pts',(22.4009680446668,-88.7444871744531,9.53109092342626));
#25136=CARTESIAN_POINT('Ctrl Pts',(25.8523951731073,-88.8820464105141,9.37310775817762));
#25137=CARTESIAN_POINT('Ctrl Pts',(27.6235721938174,-91.847285073477,9.215124592929));
#25138=CARTESIAN_POINT('Ctrl Pts',(26.1080771138749,-94.9512425629647,9.05714142768035));
#25139=CARTESIAN_POINT('Ctrl Pts',(22.6804686869861,-95.3782238204297,8.89915826243172));
#25140=CARTESIAN_POINT('Ctrl Pts',(20.4497277644465,-92.7410889898032,8.74117509718309));
#25141=CARTESIAN_POINT('Ctrl Pts',(21.4392012341389,-89.4317375405466,8.58319193193445));
#25142=CARTESIAN_POINT('Ctrl Pts',(24.7514084034007,-88.4518993616932,8.42520876668581));
#25143=CARTESIAN_POINT('Ctrl Pts',(27.3820616157699,-90.6903039066151,8.26722560143718));
#25144=CARTESIAN_POINT('Ctrl Pts',(26.9450699403022,-94.1166502818289,8.10924243618855));
#25145=CARTESIAN_POINT('Ctrl Pts',(23.8367990946118,-95.6231212490058,7.95125927093992));
#25146=CARTESIAN_POINT('Ctrl Pts',(20.8765571447007,-93.8432982426317,7.79327610569128));
#25147=CARTESIAN_POINT('Ctrl Pts',(20.7493844233325,-90.391540489283,7.63529294044265));
#25148=CARTESIAN_POINT('Ctrl Pts',(23.5706310054557,-88.3987105715367,7.47730977519401));
#25149=CARTESIAN_POINT('Ctrl Pts',(26.7813299086865,-89.6723730071853,7.31932660994538));
#25150=CARTESIAN_POINT('Ctrl Pts',(27.4692676579736,-93.0572726103796,7.16134344469675));
#25151=CARTESIAN_POINT('Ctrl Pts',(25.0104612250054,-95.483189850294,7.00336027944811));
#25152=CARTESIAN_POINT('Ctrl Pts',(21.6351319731846,-94.7497350164036,6.84537711419948));
#25153=CARTESIAN_POINT('Ctrl Pts',(20.4048187389981,-91.5221766638055,6.68739394895084));
#25154=CARTESIAN_POINT('Ctrl Pts',(22.4354576201274,-88.7280203884636,6.52941078370221));
#25155=CARTESIAN_POINT('Ctrl Pts',(25.8851898408183,-88.9016612993893,6.37142761845357));
#25156=CARTESIAN_POINT('Ctrl Pts',(27.6249905303984,-91.885601165237,6.21344445320494));
#25157=CARTESIAN_POINT('Ctrl Pts',(26.0768010801705,-94.9733046786333,6.0554612879563));
#25158=CARTESIAN_POINT('Ctrl Pts',(22.6448821645724,-95.3641193633754,5.89747812270767));
#25159=CARTESIAN_POINT('Ctrl Pts',(20.4421013787792,-92.7035629608637,5.73949495745903));
#25160=CARTESIAN_POINT('Ctrl Pts',(21.4664560811345,-89.4048509387775,5.5815117922104));
#25161=CARTESIAN_POINT('Ctrl Pts',(24.7888215932045,-88.4600276931838,5.42352862696176));
#25162=CARTESIAN_POINT('Ctrl Pts',(27.3956989960243,-90.726080156768,5.26554546171313));
#25163=CARTESIAN_POINT('Ctrl Pts',(26.9225615070512,-94.1476213996829,5.10756229646449));
#25164=CARTESIAN_POINT('Ctrl Pts',(23.7985609777147,-95.6211967303539,4.94957913121586));
#25165=CARTESIAN_POINT('Ctrl Pts',(20.8572725175022,-93.8102230269998,4.79159596596722));
#25166=CARTESIAN_POINT('Ctrl Pts',(20.7665451511942,-90.3573152521542,4.6336128007186));
#25167=CARTESIAN_POINT('Ctrl Pts',(23.6086716990241,-88.3943786103439,4.47562963546995));
#25168=CARTESIAN_POINT('Ctrl Pts',(26.8057463695968,-89.7018636398323,4.31764647022133));
#25169=CARTESIAN_POINT('Ctrl Pts',(27.4579133231717,-93.0938367815869,4.15966330497269));
#25170=CARTESIAN_POINT('Ctrl Pts',(24.9736348536359,-95.4936626411861,4.00168013972405));
#25171=CARTESIAN_POINT('Ctrl Pts',(21.6062363661592,-94.7246172109745,3.84369697447542));
#25172=CARTESIAN_POINT('Ctrl Pts',(20.410063144629,-91.4842510306948,3.68571380922679));
#25173=CARTESIAN_POINT('Ctrl Pts',(22.4700852939276,-88.7116866521341,3.52773064397815));
#25174=CARTESIAN_POINT('Ctrl Pts',(25.9177920746621,-88.9217349563625,3.36974747872952));
#25175=CARTESIAN_POINT('Ctrl Pts',(27.6259964474171,-91.9238742346134,3.21176431348088));
#25176=CARTESIAN_POINT('Ctrl Pts',(26.0452973355111,-94.9950631778383,3.05378114823225));
#25177=CARTESIAN_POINT('Ctrl Pts',(22.6094456576622,-95.3496255535895,2.89579798298361));
#25178=CARTESIAN_POINT('Ctrl Pts',(20.4348702935058,-92.665967383395,2.73781481773498));
#25179=CARTESIAN_POINT('Ctrl Pts',(21.4939973007808,-89.3782455666376,2.57983165248634));
#25180=CARTESIAN_POINT('Ctrl Pts',(24.8261378655289,-88.4685618660265,2.42184848723771));
#25181=CARTESIAN_POINT('Ctrl Pts',(27.4089767382702,-90.7619776329038,2.26386532198907));
#25182=CARTESIAN_POINT('Ctrl Pts',(26.8996888283721,-94.1783943608088,2.10588215674044));
#25183=CARTESIAN_POINT('Ctrl Pts',(23.7604241409854,-95.6187851374897,1.9478989914918));
#25184=CARTESIAN_POINT('Ctrl Pts',(20.838177062264,-93.7771163895153,1.78991582624317));
#25185=CARTESIAN_POINT('Ctrl Pts',(20.7843952072639,-90.3229253124378,1.63193266099454));
#25186=CARTESIAN_POINT('Ctrl Pts',(23.6460838609915,-88.3911589633379,1.4739494957459));
#25187=CARTESIAN_POINT('Ctrl Pts',(26.8312242725849,-89.7301456837401,1.31596633049727));
#25188=CARTESIAN_POINT('Ctrl Pts',(27.4433140827682,-93.1332953965992,1.15798316524863));
#25189=CARTESIAN_POINT('Ctrl Pts',(25.7762533017603,-94.7065713079336,1.05266105508288));
#25190=CARTESIAN_POINT('Ctrl Pts',(24.7937992825328,-94.9692229537457,0.999999999999999));
#25191=CARTESIAN_POINT('Ctrl Pts',(25.913465996665,-90.364012796625,10.));
#25192=CARTESIAN_POINT('Ctrl Pts',(25.9750770578958,-90.42191206544,10.));
#25193=CARTESIAN_POINT('Ctrl Pts',(26.0333190151654,-90.4829618973507,10.));
#25194=CARTESIAN_POINT('Ctrl Pts',(26.088194198786,-90.5467775157042,10.));
#25195=CARTESIAN_POINT('Ctrl Pts',(26.1445220900387,-90.6122825213128,10.));
#25196=CARTESIAN_POINT('Ctrl Pts',(26.1973030283134,-90.6807021204442,10.));
#25197=CARTESIAN_POINT('Ctrl Pts',(26.2465140266804,-90.7516687130586,10.));
#25198=CARTESIAN_POINT('Ctrl Pts',(26.2970865251746,-90.8245987087349,10.));
#25199=CARTESIAN_POINT('Ctrl Pts',(26.3438893496051,-90.9002191359304,10.));
#25200=CARTESIAN_POINT('Ctrl Pts',(26.3868634537168,-90.9781740458832,10.));
#25201=CARTESIAN_POINT('Ctrl Pts',(26.4057549128521,-91.0124431022419,10.));
#25202=CARTESIAN_POINT('Ctrl Pts',(26.4239059912884,-91.0471637926723,10.));
#25203=CARTESIAN_POINT('Ctrl Pts',(26.4413092551554,-91.0823079492062,10.));
#25204=CARTESIAN_POINT('Ctrl Pts',(26.4512342776009,-91.102350542658,10.));
#25205=CARTESIAN_POINT('Ctrl Pts',(26.460916053907,-91.1225308841626,10.));
#25206=CARTESIAN_POINT('Ctrl Pts',(26.4703529715556,-91.1428438969994,10.));
#25207=CARTESIAN_POINT('Ctrl Pts',(26.4788699915109,-91.1611768254115,10.));
#25208=CARTESIAN_POINT('Ctrl Pts',(26.4871899465583,-91.1796235689466,10.));
#25209=CARTESIAN_POINT('Ctrl Pts',(26.49529795661,-91.1981485646354,10.));
#25210=CARTESIAN_POINT('Ctrl Pts',(26.5318626758695,-91.2816907978493,10.));
#25211=CARTESIAN_POINT('Ctrl Pts',(26.5641670779443,-91.3669165275728,10.));
#25212=CARTESIAN_POINT('Ctrl Pts',(26.5921860624111,-91.4534270378763,10.));
#25213=CARTESIAN_POINT('Ctrl Pts',(26.620667737277,-91.5413661360929,10.));
#25214=CARTESIAN_POINT('Ctrl Pts',(26.6447217851763,-91.6306335526386,10.));
#25215=CARTESIAN_POINT('Ctrl Pts',(26.6642827659638,-91.7208476134984,10.));
#25216=CARTESIAN_POINT('Ctrl Pts',(26.6832631734456,-91.8083841053703,10.));
#25217=CARTESIAN_POINT('Ctrl Pts',(26.6980134264455,-91.8968127992612,10.));
#25218=CARTESIAN_POINT('Ctrl Pts',(26.708432920618,-91.9858069093381,10.));
#25219=CARTESIAN_POINT('Ctrl Pts',(26.7127922670542,-92.0230405936396,10.));
#25220=CARTESIAN_POINT('Ctrl Pts',(26.7163930212362,-92.0603734428051,10.));
#25221=CARTESIAN_POINT('Ctrl Pts',(26.7192254940143,-92.0977821388405,10.));
#25222=CARTESIAN_POINT('Ctrl Pts',(26.7209960695381,-92.1211662723398,10.));
#25223=CARTESIAN_POINT('Ctrl Pts',(26.7224664121851,-92.1445800482928,10.));
#25224=CARTESIAN_POINT('Ctrl Pts',(26.7236338650196,-92.16801780341,10.));
#25225=CARTESIAN_POINT('Ctrl Pts',(26.7243181282437,-92.1817550554931,10.));
#25226=CARTESIAN_POINT('Ctrl Pts',(26.7248980652474,-92.1954959766348,10.));
#25227=CARTESIAN_POINT('Ctrl Pts',(26.7253731538326,-92.2092311923284,10.));
#25228=CARTESIAN_POINT('Ctrl Pts',(26.7287309598136,-92.3063082235341,10.));
#25229=CARTESIAN_POINT('Ctrl Pts',(26.7268615808529,-92.4032207088423,10.));
#25230=CARTESIAN_POINT('Ctrl Pts',(26.7197002220063,-92.4995463878723,10.));
#25231=CARTESIAN_POINT('Ctrl Pts',(26.7125388631598,-92.5958720669024,10.));
#25232=CARTESIAN_POINT('Ctrl Pts',(26.7000859592924,-92.69161199417,10.));
#25233=CARTESIAN_POINT('Ctrl Pts',(26.6822238228945,-92.7863628481204,10.));
#25234=CARTESIAN_POINT('Ctrl Pts',(26.6651462975084,-92.8769516823811,10.));
#25235=CARTESIAN_POINT('Ctrl Pts',(26.6431244275633,-92.9666373988202,10.));
#25236=CARTESIAN_POINT('Ctrl Pts',(26.6164329081475,-93.0551806589545,10.));
#25237=CARTESIAN_POINT('Ctrl Pts',(26.6074980340548,-93.084820143644,10.));
#25238=CARTESIAN_POINT('Ctrl Pts',(26.5980394679049,-93.1143315742049,10.));
#25239=CARTESIAN_POINT('Ctrl Pts',(26.5880662379445,-93.1437057941631,10.));
#25240=CARTESIAN_POINT('Ctrl Pts',(26.5815849548277,-93.1627951600598,10.));
#25241=CARTESIAN_POINT('Ctrl Pts',(26.574886301904,-93.1818265755705,10.));
#25242=CARTESIAN_POINT('Ctrl Pts',(26.5679726206436,-93.2007974926138,10.));
#25243=CARTESIAN_POINT('Ctrl Pts',(26.5613831133059,-93.2188788869321,10.));
#25244=CARTESIAN_POINT('Ctrl Pts',(26.5545965181547,-93.2369095329036,10.));
#25245=CARTESIAN_POINT('Ctrl Pts',(26.5476256545847,-93.2548600742594,10.));
#25246=CARTESIAN_POINT('Ctrl Pts',(26.5137821756247,-93.3420097885806,10.));
#25247=CARTESIAN_POINT('Ctrl Pts',(26.475560354929,-93.4273852002263,10.));
#25248=CARTESIAN_POINT('Ctrl Pts',(26.4332913756107,-93.5107526953461,10.));
#25249=CARTESIAN_POINT('Ctrl Pts',(26.3894531454603,-93.5972152382575,10.));
#25250=CARTESIAN_POINT('Ctrl Pts',(26.3412615514558,-93.6815187324214,10.));
#25251=CARTESIAN_POINT('Ctrl Pts',(26.2890300743574,-93.7633995605516,10.));
#25252=CARTESIAN_POINT('Ctrl Pts',(26.2362101789054,-93.8462028244383,10.));
#25253=CARTESIAN_POINT('Ctrl Pts',(26.1792584552573,-93.9265293490527,10.));
#25254=CARTESIAN_POINT('Ctrl Pts',(26.1184473134232,-94.0040916613995,10.));
#25255=CARTESIAN_POINT('Ctrl Pts',(26.0767848212129,-94.0572305950965,10.));
#25256=CARTESIAN_POINT('Ctrl Pts',(26.0333097149824,-94.1090717581195,10.));
#25257=CARTESIAN_POINT('Ctrl Pts',(25.9880973827582,-94.1595156628907,10.));
#25258=CARTESIAN_POINT('Ctrl Pts',(25.9759903695684,-94.1730235929258,10.));
#25259=CARTESIAN_POINT('Ctrl Pts',(25.9637574536017,-94.1864325457022,10.));
#25260=CARTESIAN_POINT('Ctrl Pts',(25.9514137007238,-94.1997261136577,10.));
#25261=CARTESIAN_POINT('Ctrl Pts',(25.8827528893147,-94.2736701703296,10.));
#25262=CARTESIAN_POINT('Ctrl Pts',(25.810578186298,-94.3441463401242,10.));
#25263=CARTESIAN_POINT('Ctrl Pts',(25.7352000515214,-94.4108648135128,10.));
#25264=CARTESIAN_POINT('Ctrl Pts',(25.6722951822122,-94.4665429867847,10.));
#25265=CARTESIAN_POINT('Ctrl Pts',(25.6071582640081,-94.5196041737155,10.));
#25266=CARTESIAN_POINT('Ctrl Pts',(25.5399460671016,-94.5698661697058,10.));
#25267=CARTESIAN_POINT('Ctrl Pts',(25.5180638151793,-94.5862299505225,10.));
#25268=CARTESIAN_POINT('Ctrl Pts',(25.4959614387747,-94.6022969068063,10.));
#25269=CARTESIAN_POINT('Ctrl Pts',(25.4736439219636,-94.6180603652556,10.));
#25270=CARTESIAN_POINT('Ctrl Pts',(25.4508750769085,-94.6341426089032,10.));
#25271=CARTESIAN_POINT('Ctrl Pts',(25.4278768876981,-94.649912383158,10.));
#25272=CARTESIAN_POINT('Ctrl Pts',(25.4046837834431,-94.665343374446,10.));
#25273=CARTESIAN_POINT('Ctrl Pts',(25.3197384869509,-94.7218597474041,10.));
#25274=CARTESIAN_POINT('Ctrl Pts',(25.2321269167437,-94.773875691111,10.));
#25275=CARTESIAN_POINT('Ctrl Pts',(25.1421393366132,-94.8210831411639,10.));
#25276=CARTESIAN_POINT('Ctrl Pts',(25.0588657411973,-94.8647684374083,10.));
#25277=CARTESIAN_POINT('Ctrl Pts',(24.9735566410333,-94.9043362525237,10.));
#25278=CARTESIAN_POINT('Ctrl Pts',(24.8864146397765,-94.9395136119409,10.));
#25279=CARTESIAN_POINT('Ctrl Pts',(24.8563906944763,-94.9516336355772,10.));
#25280=CARTESIAN_POINT('Ctrl Pts',(24.8261489679874,-94.9632321934335,10.));
#25281=CARTESIAN_POINT('Ctrl Pts',(24.7957018439802,-94.9743128659187,10.));
#25282=CARTESIAN_POINT('Ctrl Pts',(21.4817891743669,-92.002194435609,8.38741669750802));
#25283=CARTESIAN_POINT('Ctrl Pts',(21.4802231872166,-92.1747250532131,8.39833391417657));
#25284=CARTESIAN_POINT('Ctrl Pts',(21.4964591581217,-92.3469627518866,8.40925113084511));
#25285=CARTESIAN_POINT('Ctrl Pts',(21.5315887215666,-92.5152564315154,8.42016834751366));
#25286=CARTESIAN_POINT('Ctrl Pts',(21.7010421575268,-93.3270496753528,8.47282940259653));
#25287=CARTESIAN_POINT('Ctrl Pts',(22.3101078559698,-94.0470742874782,8.52549045767941));
#25288=CARTESIAN_POINT('Ctrl Pts',(23.0825656666734,-94.3487966246852,8.57815151276228));
#25289=CARTESIAN_POINT('Ctrl Pts',(23.8550234773771,-94.6505189618922,8.63081256784516));
#25290=CARTESIAN_POINT('Ctrl Pts',(24.7908734003414,-94.5339390241808,8.68347362292804));
#25291=CARTESIAN_POINT('Ctrl Pts',(25.4656883820912,-94.0519077734106,8.73613467801092));
#25292=CARTESIAN_POINT('Ctrl Pts',(26.1405033638409,-93.5698765226404,8.7887957330938));
#25293=CARTESIAN_POINT('Ctrl Pts',(26.5542834043762,-92.7223939588113,8.84145678817668));
#25294=CARTESIAN_POINT('Ctrl Pts',(26.5193786114755,-91.8938487978225,8.89411784325956));
#25295=CARTESIAN_POINT('Ctrl Pts',(26.4844738185747,-91.0653036368338,8.94677889834244));
#25296=CARTESIAN_POINT('Ctrl Pts',(26.000884192238,-90.2556958786852,8.99943995342531));
#25297=CARTESIAN_POINT('Ctrl Pts',(25.2879127728201,-89.8321128999534,9.05210100850819));
#25298=CARTESIAN_POINT('Ctrl Pts',(24.5749413534021,-89.4085299212216,9.10476206359107));
#25299=CARTESIAN_POINT('Ctrl Pts',(23.6325881409029,-89.3709717219066,9.15742311867395));
#25300=CARTESIAN_POINT('Ctrl Pts',(22.8882531699407,-89.7366422599481,9.21008417375683));
#25301=CARTESIAN_POINT('Ctrl Pts',(22.1439181989786,-90.1023127979897,9.2627452288397));
#25302=CARTESIAN_POINT('Ctrl Pts',(21.5976014695534,-90.8712120733877,9.31540628392258));
#25303=CARTESIAN_POINT('Ctrl Pts',(21.4970122693619,-91.6942824886893,9.36806733900546));
#25304=CARTESIAN_POINT('Ctrl Pts',(21.4846923712707,-91.7950899672169,9.37451712517298));
#25305=CARTESIAN_POINT('Ctrl Pts',(21.4790586980532,-91.8967100507538,9.3809669113405));
#25306=CARTESIAN_POINT('Ctrl Pts',(21.4798238762261,-91.9984131135315,9.38741669750802));
#25307=CARTESIAN_POINT('Ctrl Pts',(23.2062007174671,-94.9692229537457,10.));
#25308=CARTESIAN_POINT('Ctrl Pts',(22.2237466982397,-94.7065713079336,9.94733894491712));
#25309=CARTESIAN_POINT('Ctrl Pts',(20.556684636792,-93.1333040393725,9.84201683475137));
#25310=CARTESIAN_POINT('Ctrl Pts',(21.1687768340777,-89.7301430813077,9.68403366950273));
#25311=CARTESIAN_POINT('Ctrl Pts',(24.3539160472627,-88.3911616367202,9.5260505042541));
#25312=CARTESIAN_POINT('Ctrl Pts',(27.2156039267669,-90.322924702785,9.36806733900546));
#25313=CARTESIAN_POINT('Ctrl Pts',(27.1618223030447,-93.7771165220753,9.21008417375683));
#25314=CARTESIAN_POINT('Ctrl Pts',(24.2395757220273,-95.6187839878382,9.0521010085082));
#25315=CARTESIAN_POINT('Ctrl Pts',(21.1003119065524,-94.1783940085773,8.89411784325955));
#25316=CARTESIAN_POINT('Ctrl Pts',(20.5910240312662,-90.7619778387773,8.73613467801092));
#25317=CARTESIAN_POINT('Ctrl Pts',(23.1738623478633,-88.4685627419331,8.57815151276229));
#25318=CARTESIAN_POINT('Ctrl Pts',(26.5060020988177,-89.3782461595948,8.42016834751365));
#25319=CARTESIAN_POINT('Ctrl Pts',(27.5651288739417,-92.6659672391889,8.26218518226502));
#25320=CARTESIAN_POINT('Ctrl Pts',(25.3905540118639,-95.3496247591348,8.10420201701639));
#25321=CARTESIAN_POINT('Ctrl Pts',(21.9547031474508,-94.9950624766612,7.94621885176775));
#25322=CARTESIAN_POINT('Ctrl Pts',(20.3740044045684,-91.923874250773,7.78823568651912));
#25323=CARTESIAN_POINT('Ctrl Pts',(22.0822083770023,-88.9217356813896,7.63025252127048));
#25324=CARTESIAN_POINT('Ctrl Pts',(25.5299143458989,-88.7116874252054,7.47226935602185));
#25325=CARTESIAN_POINT('Ctrl Pts',(27.5899360110292,-91.4842511522572,7.31428619077322));
#25326=CARTESIAN_POINT('Ctrl Pts',(26.3937630706594,-94.724616569919,7.15630302552458));
#25327=CARTESIAN_POINT('Ctrl Pts',(23.0263653754403,-95.4936618194068,6.99831986027594));
#25328=CARTESIAN_POINT('Ctrl Pts',(20.5420874902395,-93.093836524243,6.84033669502731));
#25329=CARTESIAN_POINT('Ctrl Pts',(21.194254290432,-89.7018641804574,6.68235352977868));
#25330=CARTESIAN_POINT('Ctrl Pts',(24.3913282089151,-88.3943794585145,6.52437036453004));
#25331=CARTESIAN_POINT('Ctrl Pts',(27.2334540881776,-90.35731563858,6.3663871992814));
#25332=CARTESIAN_POINT('Ctrl Pts',(27.1427267432077,-93.8102226011646,6.20840403403277));
#25333=CARTESIAN_POINT('Ctrl Pts',(24.2014389748999,-95.6211958785123,6.05042086878413));
#25334=CARTESIAN_POINT('Ctrl Pts',(21.0774391804456,-94.1476208944804,5.89243770353551));
#25335=CARTESIAN_POINT('Ctrl Pts',(20.604301802773,-90.7260804564426,5.73445453828686));
#25336=CARTESIAN_POINT('Ctrl Pts',(23.2111785923562,-88.4600285259193,5.57647137303824));
#25337=CARTESIAN_POINT('Ctrl Pts',(26.53354332288,-89.404851549255,5.4184882077896));
#25338=CARTESIAN_POINT('Ctrl Pts',(27.5578977842682,-92.7035627953589,5.26050504254097));
#25339=CARTESIAN_POINT('Ctrl Pts',(25.3551175166524,-95.3641185720074,5.10252187729234));
#25340=CARTESIAN_POINT('Ctrl Pts',(21.9231994083718,-94.973303979199,4.94453871204369));
#25341=CARTESIAN_POINT('Ctrl Pts',(20.3750103223368,-91.8856011921486,4.78655554679507));
#25342=CARTESIAN_POINT('Ctrl Pts',(22.1148106026499,-88.9016620282347,4.62857238154642));
#25343=CARTESIAN_POINT('Ctrl Pts',(25.564542011833,-88.7280211581599,4.4705892162978));
#25344=CARTESIAN_POINT('Ctrl Pts',(27.595180415279,-91.5221767762026,4.31260605104916));
#25345=CARTESIAN_POINT('Ctrl Pts',(26.3648674705088,-94.7497343695717,4.15462288580052));
#25346=CARTESIAN_POINT('Ctrl Pts',(22.9895390126931,-95.4831890308962,3.99663972055189));
#25347=CARTESIAN_POINT('Ctrl Pts',(20.5307331581304,-93.0572723617073,3.83865655530325));
#25348=CARTESIAN_POINT('Ctrl Pts',(21.2186707455856,-89.6723735546569,3.68067339005462));
#25349=CARTESIAN_POINT('Ctrl Pts',(24.429368893546,-88.3987114188411,3.52269022480599));
#25350=CARTESIAN_POINT('Ctrl Pts',(27.2506148119859,-90.3915408673734,3.36470705955735));
#25351=CARTESIAN_POINT('Ctrl Pts',(27.1234421205799,-93.8432978095595,3.20672389430872));
#25352=CARTESIAN_POINT('Ctrl Pts',(24.1632008669201,-95.6231203956682,3.04874072906008));
#25353=CARTESIAN_POINT('Ctrl Pts',(21.0549307526672,-94.1166497859116,2.89075756381145));
#25354=CARTESIAN_POINT('Ctrl Pts',(20.6179391794157,-90.6903042108868,2.73277439856281));
#25355=CARTESIAN_POINT('Ctrl Pts',(23.2485917742673,-88.4519002035991,2.57479123331418));
#25356=CARTESIAN_POINT('Ctrl Pts',(26.5607981614372,-89.4317381309793,2.41680806806554));
#25357=CARTESIAN_POINT('Ctrl Pts',(27.5502714048858,-92.7410888412383,2.25882490281691));
#25358=CARTESIAN_POINT('Ctrl Pts',(25.3195309927208,-95.3782229777193,2.10084173756827));
#25359=CARTESIAN_POINT('Ctrl Pts',(21.8919234036861,-94.9512419574066,1.94285857231964));
#25360=CARTESIAN_POINT('Ctrl Pts',(20.3764286113538,-91.8472849474597,1.78487540707101));
#25361=CARTESIAN_POINT('Ctrl Pts',(22.1476053652116,-88.8820474355396,1.62689224182237));
#25362=CARTESIAN_POINT('Ctrl Pts',(25.5990313571955,-88.7444874247256,1.46890907657374));
#25363=CARTESIAN_POINT('Ctrl Pts',(27.5999505159819,-91.5606294856851,1.3109259113251));
#25364=CARTESIAN_POINT('Ctrl Pts',(26.33585874306,-94.7735779839873,1.15294274607647));
#25365=CARTESIAN_POINT('Ctrl Pts',(22.9525246480966,-95.4743158223952,0.994959580827833));
#25366=CARTESIAN_POINT('Ctrl Pts',(20.5204066563018,-93.0164786759463,0.836976415579198));
#25367=CARTESIAN_POINT('Ctrl Pts',(21.0030718657857,-90.7756529106095,0.731654305413442));
#25368=CARTESIAN_POINT('Ctrl Pts',(21.6639373423039,-90.0026984430693,0.678993250330564));
#25369=CARTESIAN_POINT('Ctrl Pts',(23.2540671456531,-94.7901775698421,10.1070022498898));
#25370=CARTESIAN_POINT('Ctrl Pts',(22.3308555140066,-94.5433639279422,10.0543411948069));
#25371=CARTESIAN_POINT('Ctrl Pts',(20.7643179909424,-93.0649653325897,9.94901908464118));
#25372=CARTESIAN_POINT('Ctrl Pts',(21.339500773154,-89.8670164012787,9.79103591939255));
#25373=CARTESIAN_POINT('Ctrl Pts',(24.3325747618359,-88.6087760968887,9.63305275414391));
#25374=CARTESIAN_POINT('Ctrl Pts',(27.0217016673143,-90.4240530434662,9.47506958889526));
#25375=CARTESIAN_POINT('Ctrl Pts',(26.971163097959,-93.669955653763,9.31708642364665));
#25376=CARTESIAN_POINT('Ctrl Pts',(24.2251292059547,-95.400569802356,9.159103258398));
#25377=CARTESIAN_POINT('Ctrl Pts',(21.2751643093458,-94.0470359402763,9.00112009314937));
#25378=CARTESIAN_POINT('Ctrl Pts',(20.7965867055914,-90.8366310920326,8.84313692790074));
#25379=CARTESIAN_POINT('Ctrl Pts',(23.2236787932392,-88.6815098831386,8.6851537626521));
#25380=CARTESIAN_POINT('Ctrl Pts',(26.3548891258831,-89.536339010879,8.52717059740346));
#25381=CARTESIAN_POINT('Ctrl Pts',(27.3501501142311,-92.6258091365926,8.36918743215483));
#25382=CARTESIAN_POINT('Ctrl Pts',(25.3067030243257,-95.1476409875303,8.2112042669062));
#25383=CARTESIAN_POINT('Ctrl Pts',(22.0780354016688,-94.8144589587367,8.05322110165756));
#25384=CARTESIAN_POINT('Ctrl Pts',(20.5926534529996,-91.9284646652375,7.89523793640892));
#25385=CARTESIAN_POINT('Ctrl Pts',(22.1978520126389,-89.1073563051246,7.7372547711603));
#25386=CARTESIAN_POINT('Ctrl Pts',(25.4376598720287,-88.9099740464932,7.57927160591165));
#25387=CARTESIAN_POINT('Ctrl Pts',(27.3734613705941,-91.5153510231261,7.42128844066303));
#25388=CARTESIAN_POINT('Ctrl Pts',(26.249418157988,-94.5603210530949,7.26330527541438));
#25389=CARTESIAN_POINT('Ctrl Pts',(23.0850759498403,-95.2829925529257,7.10532211016576));
#25390=CARTESIAN_POINT('Ctrl Pts',(20.750601058422,-93.0278777251019,6.94733894491711));
#25391=CARTESIAN_POINT('Ctrl Pts',(21.363441928252,-89.8404427299575,6.78935577966849));
#25392=CARTESIAN_POINT('Ctrl Pts',(24.3677309545192,-88.6117998826852,6.63137261441985));
#25393=CARTESIAN_POINT('Ctrl Pts',(27.0384754565387,-90.4563701914731,6.47338944917122));
#25394=CARTESIAN_POINT('Ctrl Pts',(26.9532190083535,-93.7010654224597,6.31540628392258));
#25395=CARTESIAN_POINT('Ctrl Pts',(24.1892921206031,-95.4028362550155,6.15742311867394));
#25396=CARTESIAN_POINT('Ctrl Pts',(21.2536708181737,-94.0181184578086,5.99943995342532));
#25397=CARTESIAN_POINT('Ctrl Pts',(20.8090638219323,-90.8028983368416,5.84145678817667));
#25398=CARTESIAN_POINT('Ctrl Pts',(23.2587448526078,-88.6734902839137,5.68347362292805));
#25399=CARTESIAN_POINT('Ctrl Pts',(26.3807696026348,-89.5613400844337,5.52549045767941));
#25400=CARTESIAN_POINT('Ctrl Pts',(27.3433550622842,-92.6611376650277,5.36750729243077));
#25401=CARTESIAN_POINT('Ctrl Pts',(25.2734033645719,-95.1612608174347,5.20952412718215));
#25402=CARTESIAN_POINT('Ctrl Pts',(22.0484313512106,-94.7940125077567,5.0515409619335));
#25403=CARTESIAN_POINT('Ctrl Pts',(20.5935987135065,-91.8924994880289,4.89355779668487));
#25404=CARTESIAN_POINT('Ctrl Pts',(22.2284883104669,-89.0884931016367,4.73557463143624));
#25405=CARTESIAN_POINT('Ctrl Pts',(25.4701994752483,-88.9253228485306,4.5775914661876));
#25406=CARTESIAN_POINT('Ctrl Pts',(27.3783895350778,-91.5509897161116,4.41960830093897));
#25407=CARTESIAN_POINT('Ctrl Pts',(26.2222649745918,-94.5839242389409,4.26162513569033));
#25408=CARTESIAN_POINT('Ctrl Pts',(23.0504702321435,-95.273151277935,4.1036419704417));
#25409=CARTESIAN_POINT('Ctrl Pts',(20.73993139728,-92.9935183968345,3.94565880519306));
#25410=CARTESIAN_POINT('Ctrl Pts',(21.3863860609648,-89.8127304012066,3.78767563994443));
#25411=CARTESIAN_POINT('Ctrl Pts',(24.4034777699831,-88.6158706239953,3.6296924746958));
#25412=CARTESIAN_POINT('Ctrl Pts',(27.0546013815359,-90.4885316246794,3.47170930944716));
#25413=CARTESIAN_POINT('Ctrl Pts',(26.9350972565224,-93.7321461819781,3.31372614419853));
#25414=CARTESIAN_POINT('Ctrl Pts',(24.1533597865007,-95.4046447229832,3.15574297894989));
#25415=CARTESIAN_POINT('Ctrl Pts',(21.2325196579888,-93.9890149200185,2.99775981370126));
#25416=CARTESIAN_POINT('Ctrl Pts',(20.8218788590692,-90.769279413831,2.83977664845262));
#25417=CARTESIAN_POINT('Ctrl Pts',(23.2939020040279,-88.6658521028235,2.68179348320399));
#25418=CARTESIAN_POINT('Ctrl Pts',(26.4063809630468,-89.5866053940534,2.52381031795535));
#25419=CARTESIAN_POINT('Ctrl Pts',(27.336188556763,-92.6964008746716,2.36582715270672));
#25420=CARTESIAN_POINT('Ctrl Pts',(25.2399627228924,-95.174514721593,2.20784398745808));
#25421=CARTESIAN_POINT('Ctrl Pts',(22.0190413026667,-94.7732808350901,2.04986082220945));
#25422=CARTESIAN_POINT('Ctrl Pts',(20.5949314791037,-91.8564937288938,1.89187765696081));
#25423=CARTESIAN_POINT('Ctrl Pts',(22.2593055351527,-89.0700612770709,1.73389449171218));
#25424=CARTESIAN_POINT('Ctrl Pts',(25.5026090986845,-88.9407961923469,1.57591132646355));
#25425=CARTESIAN_POINT('Ctrl Pts',(27.3828719967166,-91.5871237111565,1.41792816121491));
#25426=CARTESIAN_POINT('Ctrl Pts',(26.1950054855207,-94.6063300734514,1.25994499596628));
#25427=CARTESIAN_POINT('Ctrl Pts',(23.0156878491875,-95.2648131276117,1.10196183071764));
#25428=CARTESIAN_POINT('Ctrl Pts',(20.7302275878235,-92.9551845873582,0.943978665469009));
#25429=CARTESIAN_POINT('Ctrl Pts',(21.1837878836398,-90.8494815513233,0.838656555303253));
#25430=CARTESIAN_POINT('Ctrl Pts',(21.8048028959809,-90.1231365609212,0.785995500220375));
#25431=CARTESIAN_POINT('Ctrl Pts',(23.301933573839,-94.6111321859386,10.2140044997796));
#25432=CARTESIAN_POINT('Ctrl Pts',(22.4379643297735,-94.3801565479507,10.1613434446967));
#25433=CARTESIAN_POINT('Ctrl Pts',(20.9719513450928,-92.9966266258069,10.056021334531));
#25434=CARTESIAN_POINT('Ctrl Pts',(21.5102247122303,-90.0038897212497,9.89803816928235));
#25435=CARTESIAN_POINT('Ctrl Pts',(24.3112334764091,-88.8263905570572,9.74005500403372));
#25436=CARTESIAN_POINT('Ctrl Pts',(26.8277994078617,-90.5251813841474,9.58207183878508));
#25437=CARTESIAN_POINT('Ctrl Pts',(26.7805038928733,-93.5627947854507,9.42408867353645));
#25438=CARTESIAN_POINT('Ctrl Pts',(24.2106826898821,-95.1823556168738,9.26610550828782));
#25439=CARTESIAN_POINT('Ctrl Pts',(21.4500167121393,-93.9156778719755,9.10812234303918));
#25440=CARTESIAN_POINT('Ctrl Pts',(21.0021493799167,-90.9112843452878,8.95013917779055));
#25441=CARTESIAN_POINT('Ctrl Pts',(23.273495238615,-88.8944570243441,8.79215601254191));
#25442=CARTESIAN_POINT('Ctrl Pts',(26.2037761529486,-89.6944318621631,8.63417284729328));
#25443=CARTESIAN_POINT('Ctrl Pts',(27.1351713545205,-92.5856510339964,8.47618968204464));
#25444=CARTESIAN_POINT('Ctrl Pts',(25.2228520367874,-94.9456572159259,8.31820651679601));
#25445=CARTESIAN_POINT('Ctrl Pts',(22.2013676558868,-94.633855440812,8.16022335154738));
#25446=CARTESIAN_POINT('Ctrl Pts',(20.8113025014308,-91.933055079702,8.00224018629874));
#25447=CARTESIAN_POINT('Ctrl Pts',(22.3134956482754,-89.2929769288594,7.8442570210501));
#25448=CARTESIAN_POINT('Ctrl Pts',(25.3454053981585,-89.1082606677813,7.68627385580147));
#25449=CARTESIAN_POINT('Ctrl Pts',(27.1569867301589,-91.5464508939948,7.52829069055284));
#25450=CARTESIAN_POINT('Ctrl Pts',(26.1050732453166,-94.3960255362711,7.37030752530419));
#25451=CARTESIAN_POINT('Ctrl Pts',(23.1437865242403,-95.0723232864444,7.21232436005558));
#25452=CARTESIAN_POINT('Ctrl Pts',(20.9591146266045,-92.961918925961,7.05434119480693));
#25453=CARTESIAN_POINT('Ctrl Pts',(21.5326295660721,-89.9790212794577,6.8963580295583));
#25454=CARTESIAN_POINT('Ctrl Pts',(24.3441337001234,-88.8292203068559,6.73837486430966));
#25455=CARTESIAN_POINT('Ctrl Pts',(26.8434968248997,-90.5554247443661,6.58039169906103));
#25456=CARTESIAN_POINT('Ctrl Pts',(26.7637112734993,-93.5919082437549,6.4224085338124));
#25457=CARTESIAN_POINT('Ctrl Pts',(24.1771452663062,-95.1844766315186,6.26442536856376));
#25458=CARTESIAN_POINT('Ctrl Pts',(21.4299024559019,-93.888616021137,6.10644220331513));
#25459=CARTESIAN_POINT('Ctrl Pts',(21.0138258410916,-90.8797162172404,5.94845903806649));
#25460=CARTESIAN_POINT('Ctrl Pts',(23.3063111128594,-88.8869520419084,5.79047587281785));
#25461=CARTESIAN_POINT('Ctrl Pts',(26.2279958823895,-89.7178286196122,5.63249270756922));
#25462=CARTESIAN_POINT('Ctrl Pts',(27.1288123403003,-92.6187125346964,5.47450954232059));
#25463=CARTESIAN_POINT('Ctrl Pts',(25.1916892124913,-94.9584030628622,5.31652637707195));
#25464=CARTESIAN_POINT('Ctrl Pts',(22.1736632940494,-94.6147210363142,5.15854321182332));
#25465=CARTESIAN_POINT('Ctrl Pts',(20.8121871046763,-91.8993977839094,5.00056004657468));
#25466=CARTESIAN_POINT('Ctrl Pts',(22.3421660182839,-89.2753241750383,4.84257688132605));
#25467=CARTESIAN_POINT('Ctrl Pts',(25.3758569386636,-89.1226245389013,4.68459371607741));
#25468=CARTESIAN_POINT('Ctrl Pts',(27.1615986548766,-91.5798026560206,4.52661055082878));
#25469=CARTESIAN_POINT('Ctrl Pts',(26.0796624786747,-94.41811410831,4.36862738558014));
#25470=CARTESIAN_POINT('Ctrl Pts',(23.111401451594,-95.0631135249739,4.21064422033151));
#25471=CARTESIAN_POINT('Ctrl Pts',(20.9491296364297,-92.9297644319617,4.05266105508288));
#25472=CARTESIAN_POINT('Ctrl Pts',(21.5541013763441,-89.9530872477562,3.89467788983424));
#25473=CARTESIAN_POINT('Ctrl Pts',(24.3775866464203,-88.8330298291496,3.73669472458561));
#25474=CARTESIAN_POINT('Ctrl Pts',(26.8585879510859,-90.5855223819854,3.57871155933697));
#25475=CARTESIAN_POINT('Ctrl Pts',(26.7467523924649,-93.6209945543966,3.42072839408834));
#25476=CARTESIAN_POINT('Ctrl Pts',(24.1435187060812,-95.1861690502982,3.2627452288397));
#25477=CARTESIAN_POINT('Ctrl Pts',(21.4101085633103,-93.8613800541255,3.10476206359107));
#25478=CARTESIAN_POINT('Ctrl Pts',(21.0258185387226,-90.8482546167753,2.94677889834243));
#25479=CARTESIAN_POINT('Ctrl Pts',(23.3392122337884,-88.8798040020478,2.7887957330938));
#25480=CARTESIAN_POINT('Ctrl Pts',(26.2519637646563,-89.7414726571277,2.63081256784516));
#25481=CARTESIAN_POINT('Ctrl Pts',(27.1221057086401,-92.6517129081048,2.47282940259653));
#25482=CARTESIAN_POINT('Ctrl Pts',(25.1603944530641,-94.9708064654669,2.31484623734789));
#25483=CARTESIAN_POINT('Ctrl Pts',(22.1461592016473,-94.5953197127737,2.15686307209926));
#25484=CARTESIAN_POINT('Ctrl Pts',(20.8134343468535,-91.8657025103278,1.99887990685063));
#25485=CARTESIAN_POINT('Ctrl Pts',(22.3710057050938,-89.2580751186022,1.84089674160199));
#25486=CARTESIAN_POINT('Ctrl Pts',(25.4061868401735,-89.1371049599684,1.68291357635336));
#25487=CARTESIAN_POINT('Ctrl Pts',(27.1657934774512,-91.6136179366278,1.52493041110472));
#25488=CARTESIAN_POINT('Ctrl Pts',(26.0541522279814,-94.4390821629154,1.36694724585609));
#25489=CARTESIAN_POINT('Ctrl Pts',(23.0788510502783,-95.0553104328282,1.20896408060746));
#25490=CARTESIAN_POINT('Ctrl Pts',(20.9400485193453,-92.8938904987702,1.05098091535882));
#25491=CARTESIAN_POINT('Ctrl Pts',(21.3645039014938,-90.923310192037,0.945658805193063));
#25492=CARTESIAN_POINT('Ctrl Pts',(21.9456684496579,-90.2435746787731,0.892997750110186));
#25493=CARTESIAN_POINT('Ctrl Pts',(23.3498000020249,-94.4320868020351,10.3210067496694));
#25494=CARTESIAN_POINT('Ctrl Pts',(22.5450731455404,-94.2169491679593,10.2683456945866));
#25495=CARTESIAN_POINT('Ctrl Pts',(21.1795846992431,-92.9282879190241,10.1630235844208));
#25496=CARTESIAN_POINT('Ctrl Pts',(21.6809486513066,-90.1407630412208,10.0050404191722));
#25497=CARTESIAN_POINT('Ctrl Pts',(24.2898921909822,-89.0440050172257,9.84705725392353));
#25498=CARTESIAN_POINT('Ctrl Pts',(26.6338971484092,-90.6263097248287,9.68907408867489));
#25499=CARTESIAN_POINT('Ctrl Pts',(26.5898446877875,-93.4556339171384,9.53109092342626));
#25500=CARTESIAN_POINT('Ctrl Pts',(24.1962361738095,-94.9641414313917,9.37310775817762));
#25501=CARTESIAN_POINT('Ctrl Pts',(21.6248691149327,-93.7843198036745,9.21512459292899));
#25502=CARTESIAN_POINT('Ctrl Pts',(21.2077120542419,-90.985937598543,9.05714142768035));
#25503=CARTESIAN_POINT('Ctrl Pts',(23.3233116839909,-89.1074041655495,8.89915826243173));
#25504=CARTESIAN_POINT('Ctrl Pts',(26.0526631800141,-89.8525247134473,8.74117509718308));
#25505=CARTESIAN_POINT('Ctrl Pts',(26.9201925948099,-92.5454929314,8.58319193193445));
#25506=CARTESIAN_POINT('Ctrl Pts',(25.1390010492492,-94.7436734443214,8.42520876668582));
#25507=CARTESIAN_POINT('Ctrl Pts',(22.3246999101049,-94.4532519228875,8.26722560143718));
#25508=CARTESIAN_POINT('Ctrl Pts',(21.029951549862,-91.9376454941666,8.10924243618855));
#25509=CARTESIAN_POINT('Ctrl Pts',(22.4291392839119,-89.4785975525942,7.95125927093991));
#25510=CARTESIAN_POINT('Ctrl Pts',(25.2531509242884,-89.3065472890693,7.79327610569128));
#25511=CARTESIAN_POINT('Ctrl Pts',(26.9405120897238,-91.5775507648634,7.63529294044265));
#25512=CARTESIAN_POINT('Ctrl Pts',(25.9607283326452,-94.2317300194472,7.47730977519401));
#25513=CARTESIAN_POINT('Ctrl Pts',(23.2024970986403,-94.8616540199631,7.31932660994538));
#25514=CARTESIAN_POINT('Ctrl Pts',(21.167628194787,-92.8959601268202,7.16134344469674));
#25515=CARTESIAN_POINT('Ctrl Pts',(21.7018172038921,-90.1175998289577,7.00336027944811));
#25516=CARTESIAN_POINT('Ctrl Pts',(24.3205364457276,-89.0466407310266,6.84537711419947));
#25517=CARTESIAN_POINT('Ctrl Pts',(26.6485181932608,-90.6544792972588,6.68739394895084));
#25518=CARTESIAN_POINT('Ctrl Pts',(26.574203538645,-93.4827510650503,6.52941078370221));
#25519=CARTESIAN_POINT('Ctrl Pts',(24.1649984120093,-94.9661170080216,6.37142761845356));
#25520=CARTESIAN_POINT('Ctrl Pts',(21.60613409363,-93.7591135844654,6.21344445320494));
#25521=CARTESIAN_POINT('Ctrl Pts',(21.2185878602508,-90.9565340976392,6.0554612879563));
#25522=CARTESIAN_POINT('Ctrl Pts',(23.353877373111,-89.100413799903,5.89747812270767));
#25523=CARTESIAN_POINT('Ctrl Pts',(26.0752221621443,-89.8743171547908,5.73949495745903));
#25524=CARTESIAN_POINT('Ctrl Pts',(26.9142696183163,-92.5762874043651,5.5815117922104));
#25525=CARTESIAN_POINT('Ctrl Pts',(25.1099750604108,-94.7555453082897,5.42352862696176));
#25526=CARTESIAN_POINT('Ctrl Pts',(22.2988952368883,-94.4354295648718,5.26554546171313));
#25527=CARTESIAN_POINT('Ctrl Pts',(21.030775495846,-91.9062960797898,5.10756229646449));
#25528=CARTESIAN_POINT('Ctrl Pts',(22.4558437261009,-89.4621552484402,4.94957913121586));
#25529=CARTESIAN_POINT('Ctrl Pts',(25.2815144020789,-89.3199262292719,4.79159596596723));
#25530=CARTESIAN_POINT('Ctrl Pts',(26.9448077746754,-91.6086155959298,4.63361280071859));
#25531=CARTESIAN_POINT('Ctrl Pts',(25.9370599827577,-94.252303977679,4.47562963546995));
#25532=CARTESIAN_POINT('Ctrl Pts',(23.1723326710444,-94.8530757720127,4.31764647022132));
#25533=CARTESIAN_POINT('Ctrl Pts',(21.1583278755794,-92.866010467089,4.15966330497269));
#25534=CARTESIAN_POINT('Ctrl Pts',(21.7218166917233,-90.0934440943057,4.00168013972405));
#25535=CARTESIAN_POINT('Ctrl Pts',(24.3516955228574,-89.0501890343038,3.84369697447542));
#25536=CARTESIAN_POINT('Ctrl Pts',(26.6625745206359,-90.6825131392915,3.68571380922678));
#25537=CARTESIAN_POINT('Ctrl Pts',(26.5584075284073,-93.5098429268151,3.52773064397815));
#25538=CARTESIAN_POINT('Ctrl Pts',(24.1336776256617,-94.9676933776133,3.36974747872952));
#25539=CARTESIAN_POINT('Ctrl Pts',(21.5876974686318,-93.7337451882324,3.21176431348088));
#25540=CARTESIAN_POINT('Ctrl Pts',(21.2297582183761,-90.9272298197194,3.05378114823225));
#25541=CARTESIAN_POINT('Ctrl Pts',(23.384522463549,-89.0937559012724,2.89579798298361));
#25542=CARTESIAN_POINT('Ctrl Pts',(26.0975465662659,-89.8963399202019,2.73781481773498));
#25543=CARTESIAN_POINT('Ctrl Pts',(26.9080228605173,-92.6070249415381,2.57983165248634));
#25544=CARTESIAN_POINT('Ctrl Pts',(25.0808261832357,-94.7670982093406,2.42184848723771));
#25545=CARTESIAN_POINT('Ctrl Pts',(22.2732771006279,-94.4173585904574,2.26386532198907));
#25546=CARTESIAN_POINT('Ctrl Pts',(21.0319372146033,-91.8749112917618,2.10588215674044));
#25547=CARTESIAN_POINT('Ctrl Pts',(22.482705875035,-89.4460889601337,1.9478989914918));
#25548=CARTESIAN_POINT('Ctrl Pts',(25.3097645816625,-89.3334137275896,1.78991582624317));
#25549=CARTESIAN_POINT('Ctrl Pts',(26.9487149581859,-91.6401121620993,1.63193266099453));
#25550=CARTESIAN_POINT('Ctrl Pts',(25.913298970442,-94.2718342523794,1.4739494957459));
#25551=CARTESIAN_POINT('Ctrl Pts',(23.1420142513692,-94.8458077380446,1.31596633049727));
#25552=CARTESIAN_POINT('Ctrl Pts',(21.149869450867,-92.8325964101822,1.15798316524863));
#25553=CARTESIAN_POINT('Ctrl Pts',(21.5452199193478,-90.9971388327507,1.05266105508287));
#25554=CARTESIAN_POINT('Ctrl Pts',(22.086534003335,-90.364012796625,0.999999999999996));
#25555=CARTESIAN_POINT('Ctrl Pts',(21.4850512338518,-91.9982506073194,9.11258330249198));
#25556=CARTESIAN_POINT('Ctrl Pts',(21.4831441979475,-91.7052247997765,9.09410267755477));
#25557=CARTESIAN_POINT('Ctrl Pts',(21.5304975843651,-91.4127948855722,9.07562205261756));
#25558=CARTESIAN_POINT('Ctrl Pts',(21.6298381693152,-91.1392457272327,9.05714142768035));
#25559=CARTESIAN_POINT('Ctrl Pts',(21.9129119308249,-90.3597597875452,9.00448037259748));
#25560=CARTESIAN_POINT('Ctrl Pts',(22.6181118074079,-89.7335819765474,8.9518193175146));
#25561=CARTESIAN_POINT('Ctrl Pts',(23.4256036617032,-89.5446798290314,8.89915826243172));
#25562=CARTESIAN_POINT('Ctrl Pts',(24.2330955159986,-89.3557776815154,8.84649720734885));
#25563=CARTESIAN_POINT('Ctrl Pts',(25.1428793480064,-89.6041511974813,8.79383615226596));
#25564=CARTESIAN_POINT('Ctrl Pts',(25.7423594998095,-90.1771659917898,8.74117509718309));
#25565=CARTESIAN_POINT('Ctrl Pts',(26.3418396516127,-90.7501807860982,8.68851404210021));
#25566=CARTESIAN_POINT('Ctrl Pts',(26.6310161232113,-91.6478368587491,8.63585298701733));
#25567=CARTESIAN_POINT('Ctrl Pts',(26.4787391014172,-92.4630283138948,8.58319193193445));
#25568=CARTESIAN_POINT('Ctrl Pts',(26.326462079623,-93.2782197690405,8.53053087685157));
#25569=CARTESIAN_POINT('Ctrl Pts',(25.7327315644361,-94.0109466066809,8.4778698217687));
#25570=CARTESIAN_POINT('Ctrl Pts',(24.9668161169853,-94.3289064385955,8.42520876668582));
#25571=CARTESIAN_POINT('Ctrl Pts',(24.2009006695344,-94.6468662705101,8.37254771160294));
#25572=CARTESIAN_POINT('Ctrl Pts',(23.2628002898197,-94.5500590966988,8.31988665652006));
#25573=CARTESIAN_POINT('Ctrl Pts',(22.5779587065885,-94.082387771673,8.26722560143718));
#25574=CARTESIAN_POINT('Ctrl Pts',(21.907599452313,-93.624606281228,8.21567816845545));
#25575=CARTESIAN_POINT('Ctrl Pts',(21.4799009347915,-92.8114801021923,8.16413073547371));
#25576=CARTESIAN_POINT('Ctrl Pts',(21.4784371162896,-91.9996804085349,8.11258330249198));
#25577=CARTESIAN_POINT('Ctrl Pts',(23.2062007174671,-94.9692229537457,10.));
#25578=CARTESIAN_POINT('Ctrl Pts',(23.113147471668,-94.9351836607662,10.));
#25579=CARTESIAN_POINT('Ctrl Pts',(23.0221595031926,-94.8963760597078,10.));
#25580=CARTESIAN_POINT('Ctrl Pts',(22.9334453118218,-94.8531283773252,10.));
#25581=CARTESIAN_POINT('Ctrl Pts',(22.842765482151,-94.8089224570377,10.));
#25582=CARTESIAN_POINT('Ctrl Pts',(22.7544606379768,-94.7600769016052,10.));
#25583=CARTESIAN_POINT('Ctrl Pts',(22.6687823668502,-94.7068967029881,10.));
#25584=CARTESIAN_POINT('Ctrl Pts',(22.5863298883886,-94.6557187424224,10.));
#25585=CARTESIAN_POINT('Ctrl Pts',(22.5063096394394,-94.60052551816,10.));
#25586=CARTESIAN_POINT('Ctrl Pts',(22.428978843944,-94.5415587834331,10.));
#25587=CARTESIAN_POINT('Ctrl Pts',(22.3613143978855,-94.489962890547,10.));
#25588=CARTESIAN_POINT('Ctrl Pts',(22.2957093551137,-94.4354772056916,10.));
#25589=CARTESIAN_POINT('Ctrl Pts',(22.2323606826166,-94.3782509736056,10.));
#25590=CARTESIAN_POINT('Ctrl Pts',(22.2182619575701,-94.3655148438681,10.));
#25591=CARTESIAN_POINT('Ctrl Pts',(22.2042723901562,-94.3526402704909,10.));
#25592=CARTESIAN_POINT('Ctrl Pts',(22.1904136245077,-94.3396473264407,10.));
#25593=CARTESIAN_POINT('Ctrl Pts',(22.1179828954075,-94.27174168213,10.));
#25594=CARTESIAN_POINT('Ctrl Pts',(22.0490178395323,-94.2005142871089,10.));
#25595=CARTESIAN_POINT('Ctrl Pts',(21.9837584040152,-94.1262557408098,10.));
#25596=CARTESIAN_POINT('Ctrl Pts',(21.9188586588109,-94.0524064852059,10.));
#25597=CARTESIAN_POINT('Ctrl Pts',(21.8576233116571,-93.9755586030696,10.));
#25598=CARTESIAN_POINT('Ctrl Pts',(21.8003319724708,-93.8959711475523,10.));
#25599=CARTESIAN_POINT('Ctrl Pts',(21.7451391407492,-93.8192988773297,10.));
#25600=CARTESIAN_POINT('Ctrl Pts',(21.6936065132598,-93.7400833150407,10.));
#25601=CARTESIAN_POINT('Ctrl Pts',(21.6460290163564,-93.6585424656019,10.));
#25602=CARTESIAN_POINT('Ctrl Pts',(21.6260402555732,-93.6242846622374,10.));
#25603=CARTESIAN_POINT('Ctrl Pts',(21.6067501857392,-93.5896163159495,10.));
#25604=CARTESIAN_POINT('Ctrl Pts',(21.5881832814551,-93.5545532938194,10.));
#25605=CARTESIAN_POINT('Ctrl Pts',(21.5751467282381,-93.5299341679298,10.));
#25606=CARTESIAN_POINT('Ctrl Pts',(21.5624667280488,-93.5051204641926,10.));
#25607=CARTESIAN_POINT('Ctrl Pts',(21.5501522393203,-93.4801176691813,10.));
#25608=CARTESIAN_POINT('Ctrl Pts',(21.5423997338202,-93.4643773237952,10.));
#25609=CARTESIAN_POINT('Ctrl Pts',(21.5347912129392,-93.448559913067,10.));
#25610=CARTESIAN_POINT('Ctrl Pts',(21.5273385775685,-93.4326879328307,10.));
#25611=CARTESIAN_POINT('Ctrl Pts',(21.485218006457,-93.3429831721704,10.));
#25612=CARTESIAN_POINT('Ctrl Pts',(21.4479996497417,-93.2513937088983,10.));
#25613=CARTESIAN_POINT('Ctrl Pts',(21.4159751546732,-93.158192004561,10.));
#25614=CARTESIAN_POINT('Ctrl Pts',(21.3861126932925,-93.0712825219783,10.));
#25615=CARTESIAN_POINT('Ctrl Pts',(21.3607666485933,-92.9829703487196,10.));
#25616=CARTESIAN_POINT('Ctrl Pts',(21.3402240440704,-92.8934677197948,10.));
#25617=CARTESIAN_POINT('Ctrl Pts',(21.3387367653612,-92.8869877549847,10.));
#25618=CARTESIAN_POINT('Ctrl Pts',(21.337274687696,-92.8805015489742,10.));
#25619=CARTESIAN_POINT('Ctrl Pts',(21.335837930805,-92.8740091819891,10.));
#25620=CARTESIAN_POINT('Ctrl Pts',(21.3152523340913,-92.7809877047229,10.));
#25621=CARTESIAN_POINT('Ctrl Pts',(21.2998605243046,-92.68670047643,10.));
#25622=CARTESIAN_POINT('Ctrl Pts',(21.2895854935829,-92.591555525086,10.));
#25623=CARTESIAN_POINT('Ctrl Pts',(21.2837678665552,-92.5376853367153,10.));
#25624=CARTESIAN_POINT('Ctrl Pts',(21.2795914703245,-92.4835403753524,10.));
#25625=CARTESIAN_POINT('Ctrl Pts',(21.2770492198358,-92.4291973958091,10.));
#25626=CARTESIAN_POINT('Ctrl Pts',(21.2764018813561,-92.4153599309664,10.));
#25627=CARTESIAN_POINT('Ctrl Pts',(21.2758606481501,-92.4015110329858,10.));
#25628=CARTESIAN_POINT('Ctrl Pts',(21.2754255840256,-92.3876642045,10.));
#25629=CARTESIAN_POINT('Ctrl Pts',(21.2724967852977,-92.2944490406402,10.));
#25630=CARTESIAN_POINT('Ctrl Pts',(21.2743673782168,-92.2011765908985,10.));
#25631=CARTESIAN_POINT('Ctrl Pts',(21.2809024940929,-92.1082221293118,10.));
#25632=CARTESIAN_POINT('Ctrl Pts',(21.2874480476023,-92.0151192044679,10.));
#25633=CARTESIAN_POINT('Ctrl Pts',(21.298673414762,-91.9223343047028,10.));
#25634=CARTESIAN_POINT('Ctrl Pts',(21.3144939864578,-91.8302566590502,10.));
#25635=CARTESIAN_POINT('Ctrl Pts',(21.3300873891571,-91.7395011645042,10.));
#25636=CARTESIAN_POINT('Ctrl Pts',(21.3501454394612,-91.6494319152931,10.));
#25637=CARTESIAN_POINT('Ctrl Pts',(21.3746301066291,-91.5604468625991,10.));
#25638=CARTESIAN_POINT('Ctrl Pts',(21.3838721759165,-91.5268582490842,10.));
#25639=CARTESIAN_POINT('Ctrl Pts',(21.3937453511932,-91.4934244348921,10.));
#25640=CARTESIAN_POINT('Ctrl Pts',(21.4042490107631,-91.4601681501231,10.));
#25641=CARTESIAN_POINT('Ctrl Pts',(21.4119449035391,-91.4358017090739,10.));
#25642=CARTESIAN_POINT('Ctrl Pts',(21.4199792750966,-91.4115305868297,10.));
#25643=CARTESIAN_POINT('Ctrl Pts',(21.4283521278725,-91.3873640201045,10.));
#25644=CARTESIAN_POINT('Ctrl Pts',(21.433519688148,-91.3724488897959,10.));
#25645=CARTESIAN_POINT('Ctrl Pts',(21.4388131893322,-91.3575822730711,10.));
#25646=CARTESIAN_POINT('Ctrl Pts',(21.4442314441212,-91.3427682605191,10.));
#25647=CARTESIAN_POINT('Ctrl Pts',(21.475937504042,-91.2560809436734,10.));
#25648=CARTESIAN_POINT('Ctrl Pts',(21.5119203351589,-91.1711677990126,10.));
#25649=CARTESIAN_POINT('Ctrl Pts',(21.5521196352014,-91.0884296535818,10.));
#25650=CARTESIAN_POINT('Ctrl Pts',(21.5822691102334,-91.0263760445086,10.));
#25651=CARTESIAN_POINT('Ctrl Pts',(21.6147913381673,-90.9655463573648,10.));
#25652=CARTESIAN_POINT('Ctrl Pts',(21.6496759689102,-90.9061246869587,10.));
#25653=CARTESIAN_POINT('Ctrl Pts',(21.6654548107415,-90.8792473739781,10.));
#25654=CARTESIAN_POINT('Ctrl Pts',(21.6817171386646,-90.8526583243667,10.));
#25655=CARTESIAN_POINT('Ctrl Pts',(21.6984627752329,-90.8263756430687,10.));
#25656=CARTESIAN_POINT('Ctrl Pts',(21.7075848158552,-90.812058379853,10.));
#25657=CARTESIAN_POINT('Ctrl Pts',(21.7168450963549,-90.7978401888656,10.));
#25658=CARTESIAN_POINT('Ctrl Pts',(21.726242936938,-90.7837240829108,10.));
#25659=CARTESIAN_POINT('Ctrl Pts',(21.7738179917341,-90.7122635693628,10.));
#25660=CARTESIAN_POINT('Ctrl Pts',(21.8249182481425,-90.6434123196867,10.));
#25661=CARTESIAN_POINT('Ctrl Pts',(21.8795126484339,-90.5775238241616,10.));
#25662=CARTESIAN_POINT('Ctrl Pts',(21.9256431731989,-90.5218501496029,10.));
#25663=CARTESIAN_POINT('Ctrl Pts',(21.9742690921716,-90.4682921528684,10.));
#25664=CARTESIAN_POINT('Ctrl Pts',(22.0253879613002,-90.4170872144436,10.));
#25665=CARTESIAN_POINT('Ctrl Pts',(22.0442197521512,-90.3982237163382,10.));
#25666=CARTESIAN_POINT('Ctrl Pts',(22.0633900127449,-90.3796798067826,10.));
#25667=CARTESIAN_POINT('Ctrl Pts',(22.0828885913556,-90.3614597865289,10.));
#25668=CARTESIAN_POINT('Origin',(24.,-92.,5.));
#25669=CARTESIAN_POINT('Origin',(24.,92.,1.));
#25670=CARTESIAN_POINT('Ctrl Pts',(22.086534003335,93.635987203375,0.999999999999996));
#25671=CARTESIAN_POINT('Ctrl Pts',(22.0243936537292,93.5775905334555,0.999999999999996));
#25672=CARTESIAN_POINT('Ctrl Pts',(21.9656286004882,93.5159401741294,1.));
#25673=CARTESIAN_POINT('Ctrl Pts',(21.9102508840716,93.4514125531564,1.));
#25674=CARTESIAN_POINT('Ctrl Pts',(21.8535184531584,93.3853063820152,1.));
#25675=CARTESIAN_POINT('Ctrl Pts',(21.8003406478354,93.3161799623012,1.));
#25676=CARTESIAN_POINT('Ctrl Pts',(21.7507593016407,93.2443917538332,1.));
#25677=CARTESIAN_POINT('Ctrl Pts',(21.737815461655,93.2256505304784,1.));
#25678=CARTESIAN_POINT('Ctrl Pts',(21.725116904748,93.2067276794587,1.));
#25679=CARTESIAN_POINT('Ctrl Pts',(21.7126647511951,93.1876291448935,1.));
#25680=CARTESIAN_POINT('Ctrl Pts',(21.7025039315265,93.1720449517797,1.));
#25681=CARTESIAN_POINT('Ctrl Pts',(21.692506743615,93.1563428865691,1.00000000000001));
#25682=CARTESIAN_POINT('Ctrl Pts',(21.6826826224521,93.1405407386175,1.00000000000001));
#25683=CARTESIAN_POINT('Ctrl Pts',(21.6352352783886,93.0642214487416,1.));
#25684=CARTESIAN_POINT('Ctrl Pts',(21.5917715084846,92.9854949382645,1.));
#25685=CARTESIAN_POINT('Ctrl Pts',(21.5523260660392,92.9047536926221,1.));
#25686=CARTESIAN_POINT('Ctrl Pts',(21.5204851858192,92.8395782966339,1.));
#25687=CARTESIAN_POINT('Ctrl Pts',(21.4912631199125,92.7730890245751,1.));
#25688=CARTESIAN_POINT('Ctrl Pts',(21.4646953254222,92.705474488561,1.));
#25689=CARTESIAN_POINT('Ctrl Pts',(21.4539704656061,92.6781799225575,1.));
#25690=CARTESIAN_POINT('Ctrl Pts',(21.4436783241418,92.6507018322004,1.));
#25691=CARTESIAN_POINT('Ctrl Pts',(21.4338220238392,92.6230520580924,1.));
#25692=CARTESIAN_POINT('Ctrl Pts',(21.4286038503028,92.6084135715299,1.));
#25693=CARTESIAN_POINT('Ctrl Pts',(21.423508396409,92.593728292269,1.));
#25694=CARTESIAN_POINT('Ctrl Pts',(21.418539882074,92.5790097941693,1.));
#25695=CARTESIAN_POINT('Ctrl Pts',(21.3890258008439,92.4915786388573,1.));
#25696=CARTESIAN_POINT('Ctrl Pts',(21.3639479991318,92.4028676021535,1.));
#25697=CARTESIAN_POINT('Ctrl Pts',(21.3433392458007,92.3132743760856,1.));
#25698=CARTESIAN_POINT('Ctrl Pts',(21.3224115739842,92.2222947034187,1.));
#25699=CARTESIAN_POINT('Ctrl Pts',(21.3060918366944,92.1304045204495,1.));
#25700=CARTESIAN_POINT('Ctrl Pts',(21.294456192223,92.037987131823,1.));
#25701=CARTESIAN_POINT('Ctrl Pts',(21.2829117114681,91.9462938210629,1.00000000000001));
#25702=CARTESIAN_POINT('Ctrl Pts',(21.2759778687866,91.8540806036969,1.00000000000001));
#25703=CARTESIAN_POINT('Ctrl Pts',(21.2737760007306,91.7617026862606,1.00000000000001));
#25704=CARTESIAN_POINT('Ctrl Pts',(21.2726808057975,91.7157545074694,1.00000000000001));
#25705=CARTESIAN_POINT('Ctrl Pts',(21.2727570661743,91.6697653696922,1.00000000000001));
#25706=CARTESIAN_POINT('Ctrl Pts',(21.2740245030464,91.6237782897535,1.00000000000001));
#25707=CARTESIAN_POINT('Ctrl Pts',(21.274441278932,91.6086561906641,1.00000000000001));
#25708=CARTESIAN_POINT('Ctrl Pts',(21.2749869696768,91.5935324627226,1.00000000000001));
#25709=CARTESIAN_POINT('Ctrl Pts',(21.2756620918863,91.5784144613223,1.00000000000001));
#25710=CARTESIAN_POINT('Ctrl Pts',(21.2799360091138,91.4827086976554,1.00000000000001));
#25711=CARTESIAN_POINT('Ctrl Pts',(21.2893769677446,91.3875701031935,1.));
#25712=CARTESIAN_POINT('Ctrl Pts',(21.304049141918,91.293397004279,1.));
#25713=CARTESIAN_POINT('Ctrl Pts',(21.3082037219408,91.2667309034811,1.));
#25714=CARTESIAN_POINT('Ctrl Pts',(21.312778033191,91.2401420861585,1.));
#25715=CARTESIAN_POINT('Ctrl Pts',(21.3177742468288,91.213639336714,1.));
#25716=CARTESIAN_POINT('Ctrl Pts',(21.3347391581856,91.1236478296194,1.));
#25717=CARTESIAN_POINT('Ctrl Pts',(21.3565643641115,91.0346487842335,1.));
#25718=CARTESIAN_POINT('Ctrl Pts',(21.3829472264989,90.9468744390412,1.));
#25719=CARTESIAN_POINT('Ctrl Pts',(21.4099265677811,90.8571156410763,1.));
#25720=CARTESIAN_POINT('Ctrl Pts',(21.4416721888843,90.7686368464218,1.));
#25721=CARTESIAN_POINT('Ctrl Pts',(21.477914698699,90.6816901122385,1.00000000000001));
#25722=CARTESIAN_POINT('Ctrl Pts',(21.4905815187717,90.6513020777609,1.00000000000001));
#25723=CARTESIAN_POINT('Ctrl Pts',(21.503798101033,90.6211012697161,1.));
#25724=CARTESIAN_POINT('Ctrl Pts',(21.5175543776486,90.5910988047965,1.));
#25725=CARTESIAN_POINT('Ctrl Pts',(21.5245011977626,90.5759477771896,1.));
#25726=CARTESIAN_POINT('Ctrl Pts',(21.531585660728,90.5608473343688,1.));
#25727=CARTESIAN_POINT('Ctrl Pts',(21.5388065373063,90.5457989336951,1.));
#25728=CARTESIAN_POINT('Ctrl Pts',(21.5448162867257,90.5332745377674,1.));
#25729=CARTESIAN_POINT('Ctrl Pts',(21.5509186842686,90.5207901234418,1.));
#25730=CARTESIAN_POINT('Ctrl Pts',(21.5571091309232,90.5083537168634,1.));
#25731=CARTESIAN_POINT('Ctrl Pts',(21.6000723361674,90.4220420307874,1.));
#25732=CARTESIAN_POINT('Ctrl Pts',(21.6473225861462,90.3379370104883,1.00000000000001));
#25733=CARTESIAN_POINT('Ctrl Pts',(21.6985178120761,90.2562887354739,1.));
#25734=CARTESIAN_POINT('Ctrl Pts',(21.7507178509555,90.1730379429873,1.));
#25735=CARTESIAN_POINT('Ctrl Pts',(21.8070195594671,90.09234050566,1.));
#25736=CARTESIAN_POINT('Ctrl Pts',(21.8671152463541,90.0144688409555,1.));
#25737=CARTESIAN_POINT('Ctrl Pts',(21.9276789686894,89.935990698459,1.));
#25738=CARTESIAN_POINT('Ctrl Pts',(21.9920964584949,89.8603816780714,1.));
#25739=CARTESIAN_POINT('Ctrl Pts',(22.0601019288122,89.7879401984298,1.));
#25740=CARTESIAN_POINT('Ctrl Pts',(22.0970286032151,89.7486047902705,1.));
#25741=CARTESIAN_POINT('Ctrl Pts',(22.1350139813229,89.7102037256098,1.));
#25742=CARTESIAN_POINT('Ctrl Pts',(22.1740207512752,89.6727885379724,1.));
#25743=CARTESIAN_POINT('Ctrl Pts',(22.1861506068063,89.6611536135409,1.));
#25744=CARTESIAN_POINT('Ctrl Pts',(22.1983792566453,89.649614047221,0.999999999999999));
#25745=CARTESIAN_POINT('Ctrl Pts',(22.2107056435596,89.6381714533068,0.999999999999999));
#25746=CARTESIAN_POINT('Ctrl Pts',(22.2219939233191,89.6276925350176,0.999999999999999));
#25747=CARTESIAN_POINT('Ctrl Pts',(22.2333584419761,89.6173003020909,1.));
#25748=CARTESIAN_POINT('Ctrl Pts',(22.2447937619035,89.6069996114494,1.));
#25749=CARTESIAN_POINT('Ctrl Pts',(22.3206028372318,89.5387124242319,1.));
#25750=CARTESIAN_POINT('Ctrl Pts',(22.3995782016253,89.4743922577898,1.));
#25751=CARTESIAN_POINT('Ctrl Pts',(22.4813936894611,89.4143217385371,1.));
#25752=CARTESIAN_POINT('Ctrl Pts',(22.5632801173719,89.3541991337043,1.));
#25753=CARTESIAN_POINT('Ctrl Pts',(22.6480121729186,89.2983327116039,1.));
#25754=CARTESIAN_POINT('Ctrl Pts',(22.7353078046389,89.2470320376965,1.));
#25755=CARTESIAN_POINT('Ctrl Pts',(22.8208396627921,89.19676787353,1.00000000000001));
#25756=CARTESIAN_POINT('Ctrl Pts',(22.9088332159369,89.1508861491376,1.));
#25757=CARTESIAN_POINT('Ctrl Pts',(22.9990569156287,89.1097141764903,1.));
#25758=CARTESIAN_POINT('Ctrl Pts',(23.0368467522455,89.0924694600261,1.));
#25759=CARTESIAN_POINT('Ctrl Pts',(23.0750281838879,89.076051483811,1.));
#25760=CARTESIAN_POINT('Ctrl Pts',(23.113585589812,89.0604866736419,1.));
#25761=CARTESIAN_POINT('Ctrl Pts',(23.1435992944682,89.048370775172,1.));
#25762=CARTESIAN_POINT('Ctrl Pts',(23.1738408319514,89.0367718698255,1.));
#25763=CARTESIAN_POINT('Ctrl Pts',(23.2042984301043,89.0256873776386,1.));
#25764=CARTESIAN_POINT('Ctrl Pts',(24.7937992825328,89.0307770462543,0.999999999999999));
#25765=CARTESIAN_POINT('Ctrl Pts',(24.8886355471735,89.0654685754907,0.999999999999998));
#25766=CARTESIAN_POINT('Ctrl Pts',(24.9814285805964,89.1051505313142,0.999999999999997));
#25767=CARTESIAN_POINT('Ctrl Pts',(25.0719374504717,89.1495026644971,0.999999999999998));
#25768=CARTESIAN_POINT('Ctrl Pts',(25.1637178578188,89.1944778901943,0.999999999999999));
#25769=CARTESIAN_POINT('Ctrl Pts',(25.2531501398721,89.2442561371166,0.999999999999999));
#25770=CARTESIAN_POINT('Ctrl Pts',(25.3399490408368,89.2985441486808,1.));
#25771=CARTESIAN_POINT('Ctrl Pts',(25.3644577827616,89.3138730393723,1.));
#25772=CARTESIAN_POINT('Ctrl Pts',(25.3887563292847,89.3295616964546,0.999999999999998));
#25773=CARTESIAN_POINT('Ctrl Pts',(25.4128376626789,89.3456039735087,0.999999999999998));
#25774=CARTESIAN_POINT('Ctrl Pts',(25.4321684184181,89.3584815552504,0.999999999999998));
#25775=CARTESIAN_POINT('Ctrl Pts',(25.4513613133248,89.3715886264076,1.));
#25776=CARTESIAN_POINT('Ctrl Pts',(25.470393428536,89.3849082415597,1.));
#25777=CARTESIAN_POINT('Ctrl Pts',(25.5531010558328,89.4427911281182,1.));
#25778=CARTESIAN_POINT('Ctrl Pts',(25.6328538472513,89.5047358079436,1.));
#25779=CARTESIAN_POINT('Ctrl Pts',(25.7093854476093,89.5704450410727,1.));
#25780=CARTESIAN_POINT('Ctrl Pts',(25.7683982886674,89.621112850351,1.));
#25781=CARTESIAN_POINT('Ctrl Pts',(25.8254952342947,89.6740199049035,1.));
#25782=CARTESIAN_POINT('Ctrl Pts',(25.8805365803869,89.729041709489,1.));
#25783=CARTESIAN_POINT('Ctrl Pts',(25.9098566849157,89.7583514044064,1.));
#25784=CARTESIAN_POINT('Ctrl Pts',(25.9385932131621,89.7882613323854,1.));
#25785=CARTESIAN_POINT('Ctrl Pts',(25.9667230183165,89.8187535094836,1.));
#25786=CARTESIAN_POINT('Ctrl Pts',(25.9763569993312,89.829196562809,1.));
#25787=CARTESIAN_POINT('Ctrl Pts',(25.9859190157893,89.8397071306231,1.));
#25788=CARTESIAN_POINT('Ctrl Pts',(25.9954015809131,89.8502769623014,1.));
#25789=CARTESIAN_POINT('Ctrl Pts',(26.0611940654473,89.9236131828441,1.));
#25790=CARTESIAN_POINT('Ctrl Pts',(26.1232543000056,89.9998957525233,1.));
#25791=CARTESIAN_POINT('Ctrl Pts',(26.1813384938245,90.0788462502489,1.));
#25792=CARTESIAN_POINT('Ctrl Pts',(26.2389162823223,90.1571084204016,1.));
#25793=CARTESIAN_POINT('Ctrl Pts',(26.2925874948895,90.2379929848863,1.));
#25794=CARTESIAN_POINT('Ctrl Pts',(26.3420688573896,90.3212511466106,1.));
#25795=CARTESIAN_POINT('Ctrl Pts',(26.3901172405319,90.402098153486,1.));
#25796=CARTESIAN_POINT('Ctrl Pts',(26.4342151409376,90.4851839694043,1.));
#25797=CARTESIAN_POINT('Ctrl Pts',(26.4740553950964,90.5702911116909,1.));
#25798=CARTESIAN_POINT('Ctrl Pts',(26.4948666592665,90.614748338641,1.));
#25799=CARTESIAN_POINT('Ctrl Pts',(26.5145153290957,90.6597572305164,0.999999999999999));
#25800=CARTESIAN_POINT('Ctrl Pts',(26.5329519176203,90.7052870235978,0.999999999999999));
#25801=CARTESIAN_POINT('Ctrl Pts',(26.5400925813213,90.7229211396022,0.999999999999999));
#25802=CARTESIAN_POINT('Ctrl Pts',(26.547051378829,90.7406333940251,1.));
#25803=CARTESIAN_POINT('Ctrl Pts',(26.5538252663872,90.7584219903797,1.));
#25804=CARTESIAN_POINT('Ctrl Pts',(26.5589791553111,90.7719563824014,1.));
#25805=CARTESIAN_POINT('Ctrl Pts',(26.5640259615885,90.7855350878376,1.));
#25806=CARTESIAN_POINT('Ctrl Pts',(26.5689595142418,90.7991434113625,1.));
#25807=CARTESIAN_POINT('Ctrl Pts',(26.6006313709989,90.8865045694709,1.));
#25808=CARTESIAN_POINT('Ctrl Pts',(26.6276945169744,90.9752266494668,0.999999999999999));
#25809=CARTESIAN_POINT('Ctrl Pts',(26.6498976668617,91.0650862423011,1.));
#25810=CARTESIAN_POINT('Ctrl Pts',(26.6549002607872,91.085332516165,1.));
#25811=CARTESIAN_POINT('Ctrl Pts',(26.659655933915,91.1056365753757,1.));
#25812=CARTESIAN_POINT('Ctrl Pts',(26.6641614464107,91.1259959208575,1.));
#25813=CARTESIAN_POINT('Ctrl Pts',(26.6845069776771,91.2179325652363,1.));
#25814=CARTESIAN_POINT('Ctrl Pts',(26.699755509991,91.3109969010619,1.));
#25815=CARTESIAN_POINT('Ctrl Pts',(26.7100169526549,91.4047971880179,1.));
#25816=CARTESIAN_POINT('Ctrl Pts',(26.7207301009459,91.50272653546,0.999999999999999));
#25817=CARTESIAN_POINT('Ctrl Pts',(26.7260074241422,91.6014592922206,0.999999999999999));
#25818=CARTESIAN_POINT('Ctrl Pts',(26.7259165033721,91.7005349801406,0.999999999999998));
#25819=CARTESIAN_POINT('Ctrl Pts',(26.7258813891798,91.7387986546182,0.999999999999998));
#25820=CARTESIAN_POINT('Ctrl Pts',(26.7250449852701,91.7771132264438,0.999999999999998));
#25821=CARTESIAN_POINT('Ctrl Pts',(26.7234090502603,91.8154509913201,0.999999999999998));
#25822=CARTESIAN_POINT('Ctrl Pts',(26.7228214486219,91.8292213020722,0.999999999999998));
#25823=CARTESIAN_POINT('Ctrl Pts',(26.7221307047635,91.8429928069669,1.));
#25824=CARTESIAN_POINT('Ctrl Pts',(26.7213377901891,91.8567525537414,1.));
#25825=CARTESIAN_POINT('Ctrl Pts',(26.7159861969284,91.9496207774894,1.));
#25826=CARTESIAN_POINT('Ctrl Pts',(26.7059788948232,92.0421019016628,0.999999999999995));
#25827=CARTESIAN_POINT('Ctrl Pts',(26.6914389406466,92.1338240299277,0.999999999999995));
#25828=CARTESIAN_POINT('Ctrl Pts',(26.6769360335326,92.2253124548821,0.999999999999995));
#25829=CARTESIAN_POINT('Ctrl Pts',(26.6579231314149,92.316046691047,1.));
#25830=CARTESIAN_POINT('Ctrl Pts',(26.6344737636544,92.4056405659079,1.));
#25831=CARTESIAN_POINT('Ctrl Pts',(26.6114256904433,92.4937011997024,1.));
#25832=CARTESIAN_POINT('Ctrl Pts',(26.584091228894,92.5806609520556,0.999999999999998));
#25833=CARTESIAN_POINT('Ctrl Pts',(26.552499862565,92.6661239169473,0.999999999999998));
#25834=CARTESIAN_POINT('Ctrl Pts',(26.5366373926815,92.709036075055,0.999999999999998));
#25835=CARTESIAN_POINT('Ctrl Pts',(26.5197010822847,92.7515703297502,0.999999999999998));
#25836=CARTESIAN_POINT('Ctrl Pts',(26.5016912750301,92.7936727826891,0.999999999999998));
#25837=CARTESIAN_POINT('Ctrl Pts',(26.4963919590575,92.806061266263,0.999999999999998));
#25838=CARTESIAN_POINT('Ctrl Pts',(26.4909996848537,92.8184123452205,0.999999999999999));
#25839=CARTESIAN_POINT('Ctrl Pts',(26.485514426691,92.8307245976522,0.999999999999999));
#25840=CARTESIAN_POINT('Ctrl Pts',(26.4799210122187,92.8432796185637,0.999999999999999));
#25841=CARTESIAN_POINT('Ctrl Pts',(26.474234590912,92.8557859781359,0.999999999999996));
#25842=CARTESIAN_POINT('Ctrl Pts',(26.4684564517529,92.8682403414366,0.999999999999996));
#25843=CARTESIAN_POINT('Ctrl Pts',(26.4309710839664,92.9490373551493,0.999999999999997));
#25844=CARTESIAN_POINT('Ctrl Pts',(26.3896160116609,93.0276775110388,0.999999999999999));
#25845=CARTESIAN_POINT('Ctrl Pts',(26.3444610577778,93.1038131058523,0.999999999999999));
#25846=CARTESIAN_POINT('Ctrl Pts',(26.3000642810644,93.1786703410435,0.999999999999999));
#25847=CARTESIAN_POINT('Ctrl Pts',(26.2519937014066,93.2511070845464,0.999999999999997));
#25848=CARTESIAN_POINT('Ctrl Pts',(26.200279482717,93.3207586728076,0.999999999999998));
#25849=CARTESIAN_POINT('Ctrl Pts',(26.1501451977981,93.388282318324,0.999999999999998));
#25850=CARTESIAN_POINT('Ctrl Pts',(26.0965860652472,93.4531888297271,1.));
#25851=CARTESIAN_POINT('Ctrl Pts',(26.0396018761895,93.5151056722102,1.));
#25852=CARTESIAN_POINT('Ctrl Pts',(26.0184128642862,93.5381288429192,1.));
#25853=CARTESIAN_POINT('Ctrl Pts',(25.9967500378082,93.5607382046918,0.999999999999995));
#25854=CARTESIAN_POINT('Ctrl Pts',(25.9746125472697,93.5829129376406,0.999999999999995));
#25855=CARTESIAN_POINT('Ctrl Pts',(25.9557857592069,93.6017713984426,0.999999999999995));
#25856=CARTESIAN_POINT('Ctrl Pts',(25.9366156438111,93.6203154841753,0.999999999999998));
#25857=CARTESIAN_POINT('Ctrl Pts',(25.9171119325404,93.6385402784441,0.999999999999998));
#25858=CARTESIAN_POINT('Origin',(24.,92.,12.2084234471775));
#25859=CARTESIAN_POINT('Ctrl Pts',(20.9232326966468,92.0019373937314,9.70842344717745));
#25860=CARTESIAN_POINT('Ctrl Pts',(20.9222985312732,92.1261020010043,9.70197366100993));
#25861=CARTESIAN_POINT('Ctrl Pts',(20.9853329189178,93.2631142772851,9.64286281975953));
#25862=CARTESIAN_POINT('Ctrl Pts',(22.4009679157595,95.2555128800838,9.53109092342627));
#25863=CARTESIAN_POINT('Ctrl Pts',(25.8523952892237,95.1179538105413,9.37310775817762));
#25864=CARTESIAN_POINT('Ctrl Pts',(27.6235723677573,92.1527148994824,9.215124592929));
#25865=CARTESIAN_POINT('Ctrl Pts',(26.1080772256066,89.0487573061685,9.05714142768035));
#25866=CARTESIAN_POINT('Ctrl Pts',(22.6804686178369,88.6217759976465,8.89915826243173));
#25867=CARTESIAN_POINT('Ctrl Pts',(21.0391555349925,90.5621016925695,8.78291893559742));
#25868=CARTESIAN_POINT('Ctrl Pts',(20.9237201879855,91.786686207045,8.719340663846));
#25869=CARTESIAN_POINT('Ctrl Pts',(20.925632029797,91.9973209161002,8.70842344717745));
#25870=CARTESIAN_POINT('Ctrl Pts',(20.929711085108,91.9968960951898,9.79157655282254));
#25871=CARTESIAN_POINT('Ctrl Pts',(20.9347146766409,92.6903800819212,9.75572892504927));
#25872=CARTESIAN_POINT('Ctrl Pts',(21.5077563627457,94.4123579721078,9.66722024219313));
#25873=CARTESIAN_POINT('Ctrl Pts',(24.3539160756188,95.60883918843,9.5260505042541));
#25874=CARTESIAN_POINT('Ctrl Pts',(27.2156041936735,93.6770751085582,9.36806733900546));
#25875=CARTESIAN_POINT('Ctrl Pts',(27.1618224985939,90.2228835192267,9.21008417375683));
#25876=CARTESIAN_POINT('Ctrl Pts',(24.2395757642923,88.3812156575976,9.05210100850819));
#25877=CARTESIAN_POINT('Ctrl Pts',(21.4675379096604,89.6531112748897,8.91259846819677));
#25878=CARTESIAN_POINT('Ctrl Pts',(20.9339205520176,91.3404824212939,8.82575698296822));
#25879=CARTESIAN_POINT('Ctrl Pts',(20.9296144608475,92.0021357572271,8.79157655282255));
#25880=CARTESIAN_POINT('Ctrl Pts',(25.9134659966651,93.6359872033749,10.));
#25881=CARTESIAN_POINT('Ctrl Pts',(26.4547800806522,93.0028611672492,9.94733894491712));
#25882=CARTESIAN_POINT('Ctrl Pts',(26.850124624194,91.1673972202025,9.84201683475137));
#25883=CARTESIAN_POINT('Ctrl Pts',(24.8579881232767,89.1541937717729,9.68403366950273));
#25884=CARTESIAN_POINT('Ctrl Pts',(22.0866994468078,89.7281636060897,9.5260505042541));
#25885=CARTESIAN_POINT('Ctrl Pts',(21.0512846745644,92.3598888261915,9.36806733900546));
#25886=CARTESIAN_POINT('Ctrl Pts',(22.6902348228159,94.6665865220793,9.21008417375683));
#25887=CARTESIAN_POINT('Ctrl Pts',(25.5172946610121,94.5539120605297,9.0521010085082));
#25888=CARTESIAN_POINT('Ctrl Pts',(26.9680635873854,92.1250885828686,8.89411784325955));
#25889=CARTESIAN_POINT('Ctrl Pts',(25.726723414825,89.5826408063379,8.73613467801094));
#25890=CARTESIAN_POINT('Ctrl Pts',(22.9191734977727,89.2329009513827,8.57815151276228));
#25891=CARTESIAN_POINT('Ctrl Pts',(21.0919763121477,91.3929749104687,8.42016834751366));
#25892=CARTESIAN_POINT('Ctrl Pts',(21.9024528317436,94.1036606678714,8.26218518226502));
#25893=CARTESIAN_POINT('Ctrl Pts',(24.6154777134031,94.9062449372411,8.10420201701639));
#25894=CARTESIAN_POINT('Ctrl Pts',(26.7702425736135,93.0727704833333,7.94621885176775));
#25895=CARTESIAN_POINT('Ctrl Pts',(26.4123032215513,90.2662543178418,7.78823568651912));
#25896=CARTESIAN_POINT('Ctrl Pts',(23.866322336025,89.0323057724808,7.63025252127049));
#25897=CARTESIAN_POINT('Ctrl Pts',(21.441591739827,90.4901566418531,7.47226935602184));
#25898=CARTESIAN_POINT('Ctrl Pts',(21.3374247177567,93.3174872372793,7.31428619077322));
#25899=CARTESIAN_POINT('Ctrl Pts',(23.6483043765504,94.9498118095941,7.15630302552458));
#25900=CARTESIAN_POINT('Ctrl Pts',(26.2781839599184,93.9065564509649,6.99831986027594));
#25901=CARTESIAN_POINT('Ctrl Pts',(26.8416729372437,91.1339892852382,6.84033669502732));
#25902=CARTESIAN_POINT('Ctrl Pts',(24.8276675656985,89.1469234118836,6.68235352977867));
#25903=CARTESIAN_POINT('Ctrl Pts',(22.0629394631722,89.7476953780895,6.52437036453004));
#25904=CARTESIAN_POINT('Ctrl Pts',(21.0551913830017,92.3913845160155,6.36638719928141));
#25905=CARTESIAN_POINT('Ctrl Pts',(22.7184852313611,94.68007453733,6.20840403403277));
#25906=CARTESIAN_POINT('Ctrl Pts',(25.5441567155844,94.5378454774748,6.05042086878414));
#25907=CARTESIAN_POINT('Ctrl Pts',(26.9692253534609,92.0937039470137,5.8924377035355));
#25908=CARTESIAN_POINT('Ctrl Pts',(25.7011052496899,89.5645697385057,5.73445453828687));
#25909=CARTESIAN_POINT('Ctrl Pts',(22.8900246220956,89.2444539035236,5.57647137303823));
#25910=CARTESIAN_POINT('Ctrl Pts',(21.0857295480958,91.4237124307955,5.4184882077896));
#25911=CARTESIAN_POINT('Ctrl Pts',(21.9247772442663,94.1256834532324,5.26050504254097));
#25912=CARTESIAN_POINT('Ctrl Pts',(24.6461228117037,94.8995870294848,5.10252187729233));
#25913=CARTESIAN_POINT('Ctrl Pts',(26.7814129353351,93.0434662008304,4.9445387120437));
#25914=CARTESIAN_POINT('Ctrl Pts',(26.3938665911029,90.2408859123632,4.78655554679506));
#25915=CARTESIAN_POINT('Ctrl Pts',(23.8350015407958,89.0338821435612,4.62857238154643));
#25916=CARTESIAN_POINT('Ctrl Pts',(21.425795725037,90.5172485108267,4.4705892162978));
#25917=CARTESIAN_POINT('Ctrl Pts',(21.3514810491689,93.3455210876134,4.31260605104916));
#25918=CARTESIAN_POINT('Ctrl Pts',(23.6794634625817,94.953360113734,4.15462288580053));
#25919=CARTESIAN_POINT('Ctrl Pts',(26.2981834534832,93.8824007094939,3.99663972055189));
#25920=CARTESIAN_POINT('Ctrl Pts',(26.8323726153541,91.1040396168705,3.83865655530326));
#25921=CARTESIAN_POINT('Ctrl Pts',(24.7975031295149,89.1383451615613,3.68067339005462));
#25922=CARTESIAN_POINT('Ctrl Pts',(22.0392711064376,89.7682693420747,3.52269022480599));
#25923=CARTESIAN_POINT('Ctrl Pts',(21.0594870693288,92.42244935621,3.36470705955735));
#25924=CARTESIAN_POINT('Ctrl Pts',(22.7468487169864,94.6934534808946,3.20672389430872));
#25925=CARTESIAN_POINT('Ctrl Pts',(25.5708611659362,94.5214031695169,3.04874072906008));
#25926=CARTESIAN_POINT('Ctrl Pts',(26.9700492986992,92.0623545219302,2.89075756381145));
#25927=CARTESIAN_POINT('Ctrl Pts',(25.6753005709136,89.5467473787502,2.73277439856282));
#25928=CARTESIAN_POINT('Ctrl Pts',(22.8609986216085,89.2563257644252,2.57479123331418));
#25929=CARTESIAN_POINT('Ctrl Pts',(21.0798065759794,91.45450692496,2.41680806806555));
#25930=CARTESIAN_POINT('Ctrl Pts',(21.9473362220071,94.1474758771513,2.25882490281691));
#25931=CARTESIAN_POINT('Ctrl Pts',(24.6766885285288,94.8925967067901,2.10084173756828));
#25932=CARTESIAN_POINT('Ctrl Pts',(26.792288712224,93.0140626065851,1.94285857231964));
#25933=CARTESIAN_POINT('Ctrl Pts',(26.3751316170022,90.2156798453631,1.78487540707101));
#25934=CARTESIAN_POINT('Ctrl Pts',(23.8037636898017,89.0358574238383,1.62689224182237));
#25935=CARTESIAN_POINT('Ctrl Pts',(21.410154680019,90.5443662144373,1.46890907657374));
#25936=CARTESIAN_POINT('Ctrl Pts',(21.3661019891308,93.3736896687444,1.3109259113251));
#25937=CARTESIAN_POINT('Ctrl Pts',(23.7101077177223,94.9559976441495,1.15294274607647));
#25938=CARTESIAN_POINT('Ctrl Pts',(26.3190524504206,93.8592343694375,0.994959580827835));
#25939=CARTESIAN_POINT('Ctrl Pts',(26.8204140260175,91.0717206863196,0.836976415579202));
#25940=CARTESIAN_POINT('Ctrl Pts',(25.4549268544596,89.7830508320407,0.731654305413445));
#25941=CARTESIAN_POINT('Ctrl Pts',(24.6501999979751,89.5679131979649,0.678993250330566));
#25942=CARTESIAN_POINT('Ctrl Pts',(26.0543315503421,93.7564253212268,10.1070022498898));
#25943=CARTESIAN_POINT('Ctrl Pts',(26.6354960985062,93.0766898079629,10.0543411948069));
#25944=CARTESIAN_POINT('Ctrl Pts',(27.0599451195336,91.1061026626961,9.94901908464117));
#25945=CARTESIAN_POINT('Ctrl Pts',(24.9211514991843,88.944691188139,9.79103591939255));
#25946=CARTESIAN_POINT('Ctrl Pts',(21.9458460727495,89.5609155378986,9.63305275414391));
#25947=CARTESIAN_POINT('Ctrl Pts',(20.8342061282629,92.3863831244189,9.47506958889527));
#25948=CARTESIAN_POINT('Ctrl Pts',(22.5938125204638,94.8628953080809,9.31708642364664));
#25949=CARTESIAN_POINT('Ctrl Pts',(25.6289948704159,94.7419259772003,9.159103258398));
#25950=CARTESIAN_POINT('Ctrl Pts',(27.186566514176,92.1342973550732,9.00112009314937));
#25951=CARTESIAN_POINT('Ctrl Pts',(25.8538413517522,89.4046796396148,8.84313692790074));
#25952=CARTESIAN_POINT('Ctrl Pts',(22.8396052044608,89.0291926334707,8.6851537626521));
#25953=CARTESIAN_POINT('Ctrl Pts',(20.8778934031181,91.348286933007,8.52717059740347));
#25954=CARTESIAN_POINT('Ctrl Pts',(21.7480355890358,94.2585279742383,8.36918743215483));
#25955=CARTESIAN_POINT('Ctrl Pts',(24.6607879561905,95.1201968981952,8.2112042669062));
#25956=CARTESIAN_POINT('Ctrl Pts',(26.9741823115717,93.1517457085875,8.05322110165757));
#25957=CARTESIAN_POINT('Ctrl Pts',(26.5898921776827,90.1386194155869,7.89523793640892));
#25958=CARTESIAN_POINT('Ctrl Pts',(23.856481252785,88.8138300372275,7.7372547711603));
#25959=CARTESIAN_POINT('Ctrl Pts',(21.2532468218983,90.3790049825179,7.57927160591166));
#25960=CARTESIAN_POINT('Ctrl Pts',(21.1414112312387,93.4144780223077,7.42128844066303));
#25961=CARTESIAN_POINT('Ctrl Pts',(23.6224132455821,95.1669710768744,7.26330527541439));
#25962=CARTESIAN_POINT('Ctrl Pts',(26.4458993232703,94.0469133376563,7.10532211016575));
#25963=CARTESIAN_POINT('Ctrl Pts',(27.0508712362317,91.0702353021323,6.94733894491713));
#25964=CARTESIAN_POINT('Ctrl Pts',(24.8885988025775,88.9368855988426,6.78935577966848));
#25965=CARTESIAN_POINT('Ctrl Pts',(21.9203369264656,89.5818852000315,6.63137261441985));
#25966=CARTESIAN_POINT('Ctrl Pts',(20.8384004407904,92.4201974641658,6.47338944917122));
#25967=CARTESIAN_POINT('Ctrl Pts',(22.624142667791,94.8773762841363,6.31540628392259));
#25968=CARTESIAN_POINT('Ctrl Pts',(25.6578344559174,94.7246766043172,6.15742311867394));
#25969=CARTESIAN_POINT('Ctrl Pts',(27.187813807155,92.1006022448672,5.99943995342532));
#25970=CARTESIAN_POINT('Ctrl Pts',(25.8263372283496,89.3852782157793,5.84145678817669));
#25971=CARTESIAN_POINT('Ctrl Pts',(22.8083104466418,89.0415960909264,5.68347362292804));
#25972=CARTESIAN_POINT('Ctrl Pts',(20.8711867647448,91.381287288329,5.52549045767941));
#25973=CARTESIAN_POINT('Ctrl Pts',(21.7720034803222,94.2821720331726,5.36750729243078));
#25974=CARTESIAN_POINT('Ctrl Pts',(24.693689085561,95.1130488485371,5.20952412718214));
#25975=CARTESIAN_POINT('Ctrl Pts',(26.9861750130638,93.1202841032021,5.05154096193351));
#25976=CARTESIAN_POINT('Ctrl Pts',(26.5700982792397,90.111383438649,4.89355779668487));
#25977=CARTESIAN_POINT('Ctrl Pts',(23.8228546830245,88.8155224576056,4.73557463143624));
#25978=CARTESIAN_POINT('Ctrl Pts',(21.2362879359765,90.4080913008988,4.57759146618761));
#25979=CARTESIAN_POINT('Ctrl Pts',(21.1565023617591,93.44457566884,4.41960830093897));
#25980=CARTESIAN_POINT('Ctrl Pts',(23.6558662014358,95.1707806000944,4.26162513569034));
#25981=CARTESIAN_POINT('Ctrl Pts',(26.4673711396979,94.0209792986338,4.1036419704417));
#25982=CARTESIAN_POINT('Ctrl Pts',(27.0408862431775,91.0380807988605,3.94565880519307));
#25983=CARTESIAN_POINT('Ctrl Pts',(24.8562137207113,88.9276758348256,3.78767563994443));
#25984=CARTESIAN_POINT('Ctrl Pts',(21.8949261524726,89.6039737782472,3.6296924746958));
#25985=CARTESIAN_POINT('Ctrl Pts',(20.8430123669848,92.453549235992,3.47170930944716));
#25986=CARTESIAN_POINT('Ctrl Pts',(22.6545942167076,94.8917401588658,3.31372614419853));
#25987=CARTESIAN_POINT('Ctrl Pts',(25.6865048346897,94.7070238464122,3.15574297894989));
#25988=CARTESIAN_POINT('Ctrl Pts',(27.1886984095998,92.0669449375797,2.99775981370126));
#25989=CARTESIAN_POINT('Ctrl Pts',(25.7986328605433,89.3661438094137,2.83977664845263));
#25990=CARTESIAN_POINT('Ctrl Pts',(22.7771476098395,89.0543419345702,2.68179348320399));
#25991=CARTESIAN_POINT('Ctrl Pts',(20.864827755224,91.4143488117893,2.52381031795536));
#25992=CARTESIAN_POINT('Ctrl Pts',(21.7962232050505,94.305568771914,2.36582715270672));
#25993=CARTESIAN_POINT('Ctrl Pts',(24.7265049895499,95.1055439122155,2.20784398745809));
#25994=CARTESIAN_POINT('Ctrl Pts',(26.9978514429749,93.0887158749414,2.04986082220945));
#25995=CARTESIAN_POINT('Ctrl Pts',(26.5499840736792,90.0843217512249,1.89187765696082));
#25996=CARTESIAN_POINT('Ctrl Pts',(23.7893171636885,88.8176431540805,1.73389449171218));
#25997=CARTESIAN_POINT('Ctrl Pts',(21.2194954283924,90.4372053558113,1.57591132646355));
#25998=CARTESIAN_POINT('Ctrl Pts',(21.1721996661856,93.4748179647817,1.41792816121491));
#25999=CARTESIAN_POINT('Ctrl Pts',(23.6887664255745,95.1736123002431,1.25994499596628));
#26000=CARTESIAN_POINT('Ctrl Pts',(26.4897764706038,93.9961074987864,1.10196183071765));
#26001=CARTESIAN_POINT('Ctrl Pts',(27.0280472863242,91.0033826130449,0.943978665469013));
#26002=CARTESIAN_POINT('Ctrl Pts',(25.5620356702265,89.6198434520492,0.838656555303256));
#26003=CARTESIAN_POINT('Ctrl Pts',(24.698066426161,89.3888678140614,0.785995500220377));
#26004=CARTESIAN_POINT('Ctrl Pts',(26.1951971040191,93.8768634390787,10.2140044997796));
#26005=CARTESIAN_POINT('Ctrl Pts',(26.8162121163603,93.1505184486766,10.1613434446967));
#26006=CARTESIAN_POINT('Ctrl Pts',(27.2697656148731,91.0448081051896,10.056021334531));
#26007=CARTESIAN_POINT('Ctrl Pts',(24.9843148750919,88.7351886045053,9.89803816928235));
#26008=CARTESIAN_POINT('Ctrl Pts',(21.8049926986913,89.3936674697073,9.74005500403372));
#26009=CARTESIAN_POINT('Ctrl Pts',(20.6171275819614,92.4128774226463,9.58207183878508));
#26010=CARTESIAN_POINT('Ctrl Pts',(22.4973902181116,95.0592040940823,9.42408867353646));
#26011=CARTESIAN_POINT('Ctrl Pts',(25.7406950798198,94.9299398938708,9.26610550828781));
#26012=CARTESIAN_POINT('Ctrl Pts',(27.4050694409667,92.1435061272778,9.10812234303919));
#26013=CARTESIAN_POINT('Ctrl Pts',(25.9809592886793,89.2267184728917,8.95013917779054));
#26014=CARTESIAN_POINT('Ctrl Pts',(22.7600369111489,88.8254843155586,8.79215601254192));
#26015=CARTESIAN_POINT('Ctrl Pts',(20.6638104940885,91.3035989555452,8.63417284729328));
#26016=CARTESIAN_POINT('Ctrl Pts',(21.593618346328,94.4133952806054,8.47618968204464));
#26017=CARTESIAN_POINT('Ctrl Pts',(24.706098198978,95.3341488591492,8.31820651679601));
#26018=CARTESIAN_POINT('Ctrl Pts',(27.1781220495298,93.2307209338419,8.16022335154737));
#26019=CARTESIAN_POINT('Ctrl Pts',(26.7674811338141,90.0109845133321,8.00224018629874));
#26020=CARTESIAN_POINT('Ctrl Pts',(23.846640169545,88.5953543019741,7.84425702105011));
#26021=CARTESIAN_POINT('Ctrl Pts',(21.0649019039697,90.2678533231826,7.68627385580147));
#26022=CARTESIAN_POINT('Ctrl Pts',(20.9453977447207,93.5114688073361,7.52829069055284));
#26023=CARTESIAN_POINT('Ctrl Pts',(23.5965221146138,95.3841303441547,7.3703075253042));
#26024=CARTESIAN_POINT('Ctrl Pts',(26.6136146866221,94.1872702243476,7.21232436005557));
#26025=CARTESIAN_POINT('Ctrl Pts',(27.2600695352198,91.0064813190264,7.05434119480693));
#26026=CARTESIAN_POINT('Ctrl Pts',(24.9495300394564,88.7268477858015,6.8963580295583));
#26027=CARTESIAN_POINT('Ctrl Pts',(21.7777343897591,89.4160750219737,6.73837486430966));
#26028=CARTESIAN_POINT('Ctrl Pts',(20.6216094985791,92.449010412316,6.58039169906103));
#26029=CARTESIAN_POINT('Ctrl Pts',(22.5298001042209,95.0746780309427,6.42240853381239));
#26030=CARTESIAN_POINT('Ctrl Pts',(25.7715121962504,94.9115077311594,6.26442536856376));
#26031=CARTESIAN_POINT('Ctrl Pts',(27.406402260849,92.1075005427209,6.10644220331512));
#26032=CARTESIAN_POINT('Ctrl Pts',(25.9515692070094,89.205986693053,5.94845903806649));
#26033=CARTESIAN_POINT('Ctrl Pts',(22.7265962711881,88.8387382783291,5.79047587281786));
#26034=CARTESIAN_POINT('Ctrl Pts',(20.6566439813937,91.3388621458626,5.63249270756922));
#26035=CARTESIAN_POINT('Ctrl Pts',(21.6192297163781,94.4386606131126,5.47450954232059));
#26036=CARTESIAN_POINT('Ctrl Pts',(24.7412553594183,95.3265106675896,5.31652637707196));
#26037=CARTESIAN_POINT('Ctrl Pts',(27.1909370907926,93.1971020055737,5.15854321182332));
#26038=CARTESIAN_POINT('Ctrl Pts',(26.7463299673765,89.9818809649348,5.00056004657469));
#26039=CARTESIAN_POINT('Ctrl Pts',(23.8107078252533,88.5971627716501,4.84257688132604));
#26040=CARTESIAN_POINT('Ctrl Pts',(21.046780146916,90.2989340909708,4.68459371607742));
#26041=CARTESIAN_POINT('Ctrl Pts',(20.9615236743494,93.5436302500665,4.52661055082878));
#26042=CARTESIAN_POINT('Ctrl Pts',(23.6322689402899,95.3882010864546,4.36862738558015));
#26043=CARTESIAN_POINT('Ctrl Pts',(26.6365588259126,94.1595578877736,4.21064422033151));
#26044=CARTESIAN_POINT('Ctrl Pts',(27.249399871001,90.9721219808506,4.05266105508288));
#26045=CARTESIAN_POINT('Ctrl Pts',(24.9149243119076,88.7170065080898,3.89467788983424));
#26046=CARTESIAN_POINT('Ctrl Pts',(21.7505811985076,89.4396782144198,3.73669472458561));
#26047=CARTESIAN_POINT('Ctrl Pts',(20.6265376646408,92.4846491157738,3.57871155933697));
#26048=CARTESIAN_POINT('Ctrl Pts',(22.5623397164288,95.0900268368369,3.42072839408834));
#26049=CARTESIAN_POINT('Ctrl Pts',(25.8021485034432,94.8926445233076,3.2627452288397));
#26050=CARTESIAN_POINT('Ctrl Pts',(27.4073475205004,92.0715353532292,3.10476206359107));
#26051=CARTESIAN_POINT('Ctrl Pts',(25.921965150173,89.1855402400772,2.94677889834244));
#26052=CARTESIAN_POINT('Ctrl Pts',(22.6932965980704,88.8523581047152,2.7887957330938));
#26053=CARTESIAN_POINT('Ctrl Pts',(20.6498489344685,91.3741906986186,2.63081256784517));
#26054=CARTESIAN_POINT('Ctrl Pts',(21.645110188094,94.4636616666768,2.47282940259653));
#26055=CARTESIAN_POINT('Ctrl Pts',(24.7763214505711,95.318491117641,2.3148462373479));
#26056=CARTESIAN_POINT('Ctrl Pts',(27.2034141737259,93.1633691432978,2.15686307209926));
#26057=CARTESIAN_POINT('Ctrl Pts',(26.7248365303562,89.9529636570868,1.99887990685063));
#26058=CARTESIAN_POINT('Ctrl Pts',(23.7748706375752,88.5994288843227,1.84089674160199));
#26059=CARTESIAN_POINT('Ctrl Pts',(21.0288361767659,90.3300444971853,1.68291357635336));
#26060=CARTESIAN_POINT('Ctrl Pts',(20.9782973432405,93.5759462608191,1.52493041110473));
#26061=CARTESIAN_POINT('Ctrl Pts',(23.6674251334267,95.3912269563368,1.36694724585609));
#26062=CARTESIAN_POINT('Ctrl Pts',(26.6605004907871,94.1329806281353,1.20896408060746));
#26063=CARTESIAN_POINT('Ctrl Pts',(27.2356805466308,90.9350445397703,1.05098091535882));
#26064=CARTESIAN_POINT('Ctrl Pts',(25.6691444859934,89.4566360720578,0.945658805193066));
#26065=CARTESIAN_POINT('Ctrl Pts',(24.7459328543469,89.2098224301578,0.892997750110188));
#26066=CARTESIAN_POINT('Ctrl Pts',(26.3360626576962,93.9973015569306,10.3210067496694));
#26067=CARTESIAN_POINT('Ctrl Pts',(26.9969281342143,93.2243470893904,10.2683456945866));
#26068=CARTESIAN_POINT('Ctrl Pts',(27.4795861102127,90.9835135476831,10.1630235844208));
#26069=CARTESIAN_POINT('Ctrl Pts',(25.0474782509994,88.5256860208715,10.0050404191722));
#26070=CARTESIAN_POINT('Ctrl Pts',(21.664139324633,89.2264194015161,9.84705725392353));
#26071=CARTESIAN_POINT('Ctrl Pts',(20.4000490356599,92.4393717208737,9.68907408867489));
#26072=CARTESIAN_POINT('Ctrl Pts',(22.4009679157595,95.2555128800838,9.53109092342627));
#26073=CARTESIAN_POINT('Ctrl Pts',(25.8523952892237,95.1179538105413,9.37310775817762));
#26074=CARTESIAN_POINT('Ctrl Pts',(27.6235723677573,92.1527148994824,9.215124592929));
#26075=CARTESIAN_POINT('Ctrl Pts',(26.1080772256066,89.0487573061685,9.05714142768035));
#26076=CARTESIAN_POINT('Ctrl Pts',(22.6804686178369,88.6217759976465,8.89915826243173));
#26077=CARTESIAN_POINT('Ctrl Pts',(20.4497275850589,91.2589109780836,8.74117509718308));
#26078=CARTESIAN_POINT('Ctrl Pts',(21.4392011036202,94.5682625869723,8.58319193193445));
#26079=CARTESIAN_POINT('Ctrl Pts',(24.7514084417654,95.5481008201034,8.42520876668582));
#26080=CARTESIAN_POINT('Ctrl Pts',(27.382061787488,93.3096961590962,8.26722560143718));
#26081=CARTESIAN_POINT('Ctrl Pts',(26.9450700899455,89.8833496110771,8.10924243618856));
#26082=CARTESIAN_POINT('Ctrl Pts',(23.8367990863051,88.3768785667208,7.95125927093992));
#26083=CARTESIAN_POINT('Ctrl Pts',(20.876556986041,90.1567016638474,7.79327610569128));
#26084=CARTESIAN_POINT('Ctrl Pts',(20.7493842582027,93.6084595923645,7.63529294044265));
#26085=CARTESIAN_POINT('Ctrl Pts',(23.5706309836456,95.601289611435,7.47730977519401));
#26086=CARTESIAN_POINT('Ctrl Pts',(26.7813300499739,94.327627111039,7.31932660994538));
#26087=CARTESIAN_POINT('Ctrl Pts',(27.4692678342079,90.9427273359204,7.16134344469674));
#26088=CARTESIAN_POINT('Ctrl Pts',(25.0104612763354,88.5168099727604,7.00336027944811));
#26089=CARTESIAN_POINT('Ctrl Pts',(21.6351318530525,89.2502648439158,6.84537711419948));
#26090=CARTESIAN_POINT('Ctrl Pts',(20.4048185563677,92.4778233604662,6.68739394895084));
#26091=CARTESIAN_POINT('Ctrl Pts',(22.4354575406508,95.2719797777492,6.5294107837022));
#26092=CARTESIAN_POINT('Ctrl Pts',(25.8851899365834,95.0983388580017,6.37142761845357));
#26093=CARTESIAN_POINT('Ctrl Pts',(27.624990714543,92.1143988405745,6.21344445320494));
#26094=CARTESIAN_POINT('Ctrl Pts',(26.0768011856691,89.0266951703267,6.0554612879563));
#26095=CARTESIAN_POINT('Ctrl Pts',(22.6448820957342,88.6358804657318,5.89747812270767));
#26096=CARTESIAN_POINT('Ctrl Pts',(20.4421011980427,91.2964370033963,5.73949495745903));
#26097=CARTESIAN_POINT('Ctrl Pts',(21.4664559524339,94.5951491930526,5.5815117922104));
#26098=CARTESIAN_POINT('Ctrl Pts',(24.7888216332756,95.5399724866421,5.42352862696176));
#26099=CARTESIAN_POINT('Ctrl Pts',(27.3956991685213,93.2739199079453,5.26554546171313));
#26100=CARTESIAN_POINT('Ctrl Pts',(26.9225616555133,89.8523784912207,5.1075622964645));
#26101=CARTESIAN_POINT('Ctrl Pts',(23.798560967482,88.3788030856943,4.94957913121586));
#26102=CARTESIAN_POINT('Ctrl Pts',(20.8572723578555,90.189776881043,4.79159596596723));
#26103=CARTESIAN_POINT('Ctrl Pts',(20.7665449869397,93.642684831293,4.63361280071859));
#26104=CARTESIAN_POINT('Ctrl Pts',(23.608671679144,95.6056215728149,4.47562963546996));
#26105=CARTESIAN_POINT('Ctrl Pts',(26.8057465121274,94.2981364769134,4.31764647022132));
#26106=CARTESIAN_POINT('Ctrl Pts',(27.4579134988245,90.9061631628407,4.15966330497269));
#26107=CARTESIAN_POINT('Ctrl Pts',(24.973634903104,88.5063371813541,4.00168013972405));
#26108=CARTESIAN_POINT('Ctrl Pts',(21.6062362445426,89.2753826505923,3.84369697447542));
#26109=CARTESIAN_POINT('Ctrl Pts',(20.4100629622968,92.5157489955558,3.68571380922678));
#26110=CARTESIAN_POINT('Ctrl Pts',(22.47008521615,95.288313514808,3.52773064397815));
#26111=CARTESIAN_POINT('Ctrl Pts',(25.9177921721966,95.0782652002028,3.36974747872952));
#26112=CARTESIAN_POINT('Ctrl Pts',(27.625996631401,92.0761257688787,3.21176431348088));
#26113=CARTESIAN_POINT('Ctrl Pts',(26.0452974398026,89.0049366707406,3.05378114823225));
#26114=CARTESIAN_POINT('Ctrl Pts',(22.6094455863014,88.6503742748602,2.89579798298361));
#26115=CARTESIAN_POINT('Ctrl Pts',(20.4348701137131,91.3340325854478,2.73781481773498));
#26116=CARTESIAN_POINT('Ctrl Pts',(21.4939971711375,94.6217545614396,2.57983165248634));
#26117=CARTESIAN_POINT('Ctrl Pts',(24.8261379115922,95.5314383230663,2.42184848723771));
#26118=CARTESIAN_POINT('Ctrl Pts',(27.4089769044768,93.2380224116542,2.26386532198907));
#26119=CARTESIAN_POINT('Ctrl Pts',(26.8996889870333,89.8216055629486,2.10588215674044));
#26120=CARTESIAN_POINT('Ctrl Pts',(23.760424111462,88.3812146145649,1.94789899149181));
#26121=CARTESIAN_POINT('Ctrl Pts',(20.8381769251394,90.2228836385593,1.78991582624317));
#26122=CARTESIAN_POINT('Ctrl Pts',(20.7843950202953,93.6770745568564,1.63193266099454));
#26123=CARTESIAN_POINT('Ctrl Pts',(23.6460838412789,95.6088416124304,1.47394949574591));
#26124=CARTESIAN_POINT('Ctrl Pts',(26.8312245109703,94.2698537574842,1.31596633049727));
#26125=CARTESIAN_POINT('Ctrl Pts',(27.4433138069374,90.8667064664957,1.15798316524863));
#26126=CARTESIAN_POINT('Ctrl Pts',(25.7762533017603,89.2934286920663,1.05266105508288));
#26127=CARTESIAN_POINT('Ctrl Pts',(24.7937992825328,89.0307770462543,0.999999999999999));
#26128=CARTESIAN_POINT('Ctrl Pts',(25.9134659966651,93.6359872033749,10.));
#26129=CARTESIAN_POINT('Ctrl Pts',(25.9750770243707,93.5780879660653,10.));
#26130=CARTESIAN_POINT('Ctrl Pts',(26.0333189464395,93.5170381633422,10.));
#26131=CARTESIAN_POINT('Ctrl Pts',(26.0881940942714,93.4532225723798,10.));
#26132=CARTESIAN_POINT('Ctrl Pts',(26.1445219524098,93.3877175906754,10.));
#26133=CARTESIAN_POINT('Ctrl Pts',(26.1973028564924,93.3192980131808,10.));
#26134=CARTESIAN_POINT('Ctrl Pts',(26.2465138207378,93.2483314405832,10.));
#26135=CARTESIAN_POINT('Ctrl Pts',(26.2970863146455,93.1754014215236,10.));
#26136=CARTESIAN_POINT('Ctrl Pts',(26.3438891300209,93.0997809659943,10.));
#26137=CARTESIAN_POINT('Ctrl Pts',(26.3868632217464,93.0218260240972,10.));
#26138=CARTESIAN_POINT('Ctrl Pts',(26.4057547014839,92.9875569064464,10.));
#26139=CARTESIAN_POINT('Ctrl Pts',(26.4239057978364,92.95283615278,10.));
#26140=CARTESIAN_POINT('Ctrl Pts',(26.4413090769957,92.9176919312917,10.));
#26141=CARTESIAN_POINT('Ctrl Pts',(26.4512341001089,92.8976493170593,10.));
#26142=CARTESIAN_POINT('Ctrl Pts',(26.460915876624,92.8774689544388,10.));
#26143=CARTESIAN_POINT('Ctrl Pts',(26.4703527940365,92.857155920179,10.));
#26144=CARTESIAN_POINT('Ctrl Pts',(26.4788698089222,92.8388229828856,10.));
#26145=CARTESIAN_POINT('Ctrl Pts',(26.4871897587641,92.8203762303378,10.));
#26146=CARTESIAN_POINT('Ctrl Pts',(26.4952977634944,92.8018512255385,10.));
#26147=CARTESIAN_POINT('Ctrl Pts',(26.5318624413855,92.7183089909258,10.));
#26148=CARTESIAN_POINT('Ctrl Pts',(26.5641668037515,92.6330832593894,10.));
#26149=CARTESIAN_POINT('Ctrl Pts',(26.5921857513776,92.5465727476703,10.));
#26150=CARTESIAN_POINT('Ctrl Pts',(26.620667393952,92.4586336320905,10.));
#26151=CARTESIAN_POINT('Ctrl Pts',(26.6447214109184,92.3693661981114,10.));
#26152=CARTESIAN_POINT('Ctrl Pts',(26.6642823633745,92.2791521208042,10.));
#26153=CARTESIAN_POINT('Ctrl Pts',(26.6832627492248,92.191615585952,10.));
#26154=CARTESIAN_POINT('Ctrl Pts',(26.698012980431,92.1031868494578,10.));
#26155=CARTESIAN_POINT('Ctrl Pts',(26.7084324537049,92.0141926984168,10.));
#26156=CARTESIAN_POINT('Ctrl Pts',(26.7127917941084,91.9769589738208,10.));
#26157=CARTESIAN_POINT('Ctrl Pts',(26.716392541471,91.9396260845242,10.));
#26158=CARTESIAN_POINT('Ctrl Pts',(26.7192250067013,91.9022173486574,10.));
#26159=CARTESIAN_POINT('Ctrl Pts',(26.7209955764808,91.8788332038123,10.));
#26160=CARTESIAN_POINT('Ctrl Pts',(26.7224659134468,91.8554194166649,10.));
#26161=CARTESIAN_POINT('Ctrl Pts',(26.723633360682,91.831981650528,10.));
#26162=CARTESIAN_POINT('Ctrl Pts',(26.7243176203471,91.8182443975509,10.));
#26163=CARTESIAN_POINT('Ctrl Pts',(26.7248975539059,91.8045034755717,10.));
#26164=CARTESIAN_POINT('Ctrl Pts',(26.7253726391654,91.7907682591116,10.));
#26165=CARTESIAN_POINT('Ctrl Pts',(26.7287304225257,91.693691196935,10.));
#26166=CARTESIAN_POINT('Ctrl Pts',(26.7268610241309,91.5967786841457,10.));
#26167=CARTESIAN_POINT('Ctrl Pts',(26.7196996503277,91.5004529825227,10.));
#26168=CARTESIAN_POINT('Ctrl Pts',(26.7125382765246,91.4041272808997,10.));
#26169=CARTESIAN_POINT('Ctrl Pts',(26.7000853621757,91.3083873359242,10.));
#26170=CARTESIAN_POINT('Ctrl Pts',(26.6822232210627,91.2136364705516,10.));
#26171=CARTESIAN_POINT('Ctrl Pts',(26.6651456877558,91.1230476072669,10.));
#26172=CARTESIAN_POINT('Ctrl Pts',(26.6431238131837,91.0333618679074,10.));
#26173=CARTESIAN_POINT('Ctrl Pts',(26.6164322917029,90.9448185902174,10.));
#26174=CARTESIAN_POINT('Ctrl Pts',(26.607497412219,90.9151790840601,10.));
#26175=CARTESIAN_POINT('Ctrl Pts',(26.5980388404141,90.8856676327678,10.));
#26176=CARTESIAN_POINT('Ctrl Pts',(26.5880656045218,90.8562933928029,10.));
#26177=CARTESIAN_POINT('Ctrl Pts',(26.5815842777575,90.8372038967034,10.));
#26178=CARTESIAN_POINT('Ctrl Pts',(26.5748855784003,90.8181723520075,10.));
#26179=CARTESIAN_POINT('Ctrl Pts',(26.5679718479592,90.7992013068406,10.));
#26180=CARTESIAN_POINT('Ctrl Pts',(26.5613824030662,90.7811200903749,10.));
#26181=CARTESIAN_POINT('Ctrl Pts',(26.5545958744166,90.763089621577,10.));
#26182=CARTESIAN_POINT('Ctrl Pts',(26.5476250811218,90.7451392560968,10.));
#26183=CARTESIAN_POINT('Ctrl Pts',(26.5137816042599,90.6579895224725,10.));
#26184=CARTESIAN_POINT('Ctrl Pts',(26.4755597867788,90.5726140968035,10.));
#26185=CARTESIAN_POINT('Ctrl Pts',(26.4332908111474,90.4892465922176,10.));
#26186=CARTESIAN_POINT('Ctrl Pts',(26.389452592761,90.4027840551495,10.));
#26187=CARTESIAN_POINT('Ctrl Pts',(26.3412610126046,90.3184805709489,10.));
#26188=CARTESIAN_POINT('Ctrl Pts',(26.2890295505471,90.2365997560241,10.));
#26189=CARTESIAN_POINT('Ctrl Pts',(26.236209676095,90.1537965145679,10.));
#26190=CARTESIAN_POINT('Ctrl Pts',(26.1792579755727,90.073470015158,10.));
#26191=CARTESIAN_POINT('Ctrl Pts',(26.1184468579959,89.9959077298432,10.));
#26192=CARTESIAN_POINT('Ctrl Pts',(26.0767843459152,89.9427687681253,10.));
#26193=CARTESIAN_POINT('Ctrl Pts',(26.0333092171723,89.8909275802125,10.));
#26194=CARTESIAN_POINT('Ctrl Pts',(25.9880968596718,89.8404836536506,10.));
#26195=CARTESIAN_POINT('Ctrl Pts',(25.9759899524187,89.8269758435267,10.));
#26196=CARTESIAN_POINT('Ctrl Pts',(25.9637571445712,89.8135670090811,10.));
#26197=CARTESIAN_POINT('Ctrl Pts',(25.9514135016898,89.8002735575422,10.));
#26198=CARTESIAN_POINT('Ctrl Pts',(25.8827527214455,89.7263295230642,10.));
#26199=CARTESIAN_POINT('Ctrl Pts',(25.8105780493431,89.6558533763024,10.));
#26200=CARTESIAN_POINT('Ctrl Pts',(25.7351999442575,89.5891349257962,10.));
#26201=CARTESIAN_POINT('Ctrl Pts',(25.6722950969812,89.5334567691903,10.));
#26202=CARTESIAN_POINT('Ctrl Pts',(25.6071581997643,89.4803955990503,10.));
#26203=CARTESIAN_POINT('Ctrl Pts',(25.5399460222554,89.4301336194353,10.));
#26204=CARTESIAN_POINT('Ctrl Pts',(25.5180637924313,89.4137698557527,10.));
#26205=CARTESIAN_POINT('Ctrl Pts',(25.4959614382739,89.3977029161308,10.));
#26206=CARTESIAN_POINT('Ctrl Pts',(25.4736439438293,89.3819394738383,10.));
#26207=CARTESIAN_POINT('Ctrl Pts',(25.4508750630273,89.3658572053077,10.));
#26208=CARTESIAN_POINT('Ctrl Pts',(25.427876837014,89.3500874072515,10.));
#26209=CARTESIAN_POINT('Ctrl Pts',(25.40468369501,89.3346563933276,10.));
#26210=CARTESIAN_POINT('Ctrl Pts',(25.3197384270948,89.2781400484641,10.));
#26211=CARTESIAN_POINT('Ctrl Pts',(25.2321268832309,89.2261241307586,10.));
#26212=CARTESIAN_POINT('Ctrl Pts',(25.1421393261502,89.1789167035765,10.));
#26213=CARTESIAN_POINT('Ctrl Pts',(25.058865760574,89.1352314329607,10.));
#26214=CARTESIAN_POINT('Ctrl Pts',(24.9735566878463,89.0956636399533,10.));
#26215=CARTESIAN_POINT('Ctrl Pts',(24.8864147107142,89.0604862982088,10.));
#26216=CARTESIAN_POINT('Ctrl Pts',(24.856390770472,89.0483662793479,10.));
#26217=CARTESIAN_POINT('Ctrl Pts',(24.8261490486008,89.0367677258533,10.));
#26218=CARTESIAN_POINT('Ctrl Pts',(24.7957019287906,89.0256870573369,10.));
#26219=CARTESIAN_POINT('Ctrl Pts',(21.481789046694,91.9978055657336,8.38741669750803));
#26220=CARTESIAN_POINT('Ctrl Pts',(21.480223059461,91.8252749393967,8.39833391417657));
#26221=CARTESIAN_POINT('Ctrl Pts',(21.4964590311695,91.653037231908,8.40925113084512));
#26222=CARTESIAN_POINT('Ctrl Pts',(21.5315885963512,91.4847435435215,8.42016834751366));
#26223=CARTESIAN_POINT('Ctrl Pts',(21.7010420406894,90.67295025744,8.47282940259653));
#26224=CARTESIAN_POINT('Ctrl Pts',(22.310107769231,89.9529256044114,8.52549045767941));
#26225=CARTESIAN_POINT('Ctrl Pts',(23.0825656196773,89.6512032537229,8.57815151276229));
#26226=CARTESIAN_POINT('Ctrl Pts',(23.8550234701235,89.3494809030345,8.63081256784517));
#26227=CARTESIAN_POINT('Ctrl Pts',(24.7908734424742,89.4660608546862,8.68347362292805));
#26228=CARTESIAN_POINT('Ctrl Pts',(25.4656884574097,89.9480921266005,8.73613467801093));
#26229=CARTESIAN_POINT('Ctrl Pts',(26.1405034723451,90.4301233985148,8.78879573309381));
#26230=CARTESIAN_POINT('Ctrl Pts',(26.5542835298653,91.2776059906917,8.84145678817668));
#26231=CARTESIAN_POINT('Ctrl Pts',(26.5193787375631,92.1061511997237,8.89411784325956));
#26232=CARTESIAN_POINT('Ctrl Pts',(26.484473945261,92.9346964087556,8.94677889834243));
#26233=CARTESIAN_POINT('Ctrl Pts',(26.0008843031365,93.7443042346426,8.99943995342532));
#26234=CARTESIAN_POINT('Ctrl Pts',(25.2879128423749,94.1678872245111,9.0521010085082));
#26235=CARTESIAN_POINT('Ctrl Pts',(24.5749413816134,94.5914702143796,9.10476206359107));
#26236=CARTESIAN_POINT('Ctrl Pts',(23.6325881022146,94.6290283682295,9.15742311867395));
#26237=CARTESIAN_POINT('Ctrl Pts',(22.8882531044733,94.2633578291731,9.21008417375683));
#26238=CARTESIAN_POINT('Ctrl Pts',(22.1439181067321,93.8976872901167,9.2627452288397));
#26239=CARTESIAN_POINT('Ctrl Pts',(21.5976013906482,93.1287880581541,9.31540628392258));
#26240=CARTESIAN_POINT('Ctrl Pts',(21.4970121613136,92.3057175721559,9.36806733900546));
#26241=CARTESIAN_POINT('Ctrl Pts',(21.484692259653,92.2049100849695,9.37451712517298));
#26242=CARTESIAN_POINT('Ctrl Pts',(21.4790585822288,92.1032899910618,9.3809669113405));
#26243=CARTESIAN_POINT('Ctrl Pts',(21.4798237559162,92.0015869167785,9.38741669750802));
#26244=CARTESIAN_POINT('Ctrl Pts',(23.2062007174671,89.0307770462543,10.));
#26245=CARTESIAN_POINT('Ctrl Pts',(22.2237466982397,89.2934286920664,9.94733894491712));
#26246=CARTESIAN_POINT('Ctrl Pts',(20.556685031954,90.8666986268702,9.84201683475136));
#26247=CARTESIAN_POINT('Ctrl Pts',(21.1687764925373,94.2698561140494,9.68403366950273));
#26248=CARTESIAN_POINT('Ctrl Pts',(24.3539160756188,95.60883918843,9.5260505042541));
#26249=CARTESIAN_POINT('Ctrl Pts',(27.2156041936735,93.6770751085582,9.36806733900546));
#26250=CARTESIAN_POINT('Ctrl Pts',(27.1618224985939,90.2228835192267,9.21008417375683));
#26251=CARTESIAN_POINT('Ctrl Pts',(24.2395757642923,88.3812156575976,9.05210100850819));
#26252=CARTESIAN_POINT('Ctrl Pts',(21.1003116800245,89.8216058830164,8.89411784325956));
#26253=CARTESIAN_POINT('Ctrl Pts',(20.5910237941294,93.238022224588,8.73613467801092));
#26254=CARTESIAN_POINT('Ctrl Pts',(23.1738622820844,95.5314375280541,8.57815151276229));
#26255=CARTESIAN_POINT('Ctrl Pts',(26.5060022838615,94.621754023121,8.42016834751365));
#26256=CARTESIAN_POINT('Ctrl Pts',(27.5651291305171,91.3340327163824,8.26218518226502));
#26257=CARTESIAN_POINT('Ctrl Pts',(25.3905541137142,88.6503749960184,8.10420201701638));
#26258=CARTESIAN_POINT('Ctrl Pts',(21.9547029986072,89.0049373072501,7.94621885176775));
#26259=CARTESIAN_POINT('Ctrl Pts',(20.3740041419998,92.0761257542051,7.78823568651912));
#26260=CARTESIAN_POINT('Ctrl Pts',(22.0822082378054,95.0782645420543,7.63025252127048));
#26261=CARTESIAN_POINT('Ctrl Pts',(25.5299144568995,95.2883128130433,7.47226935602185));
#26262=CARTESIAN_POINT('Ctrl Pts',(27.5899362712429,92.5157488852068,7.31428619077321));
#26263=CARTESIAN_POINT('Ctrl Pts',(26.3937632442238,89.2753832325168,7.15630302552458));
#26264=CARTESIAN_POINT('Ctrl Pts',(23.0263653048422,88.5063379273328,6.99831986027595));
#26265=CARTESIAN_POINT('Ctrl Pts',(20.542087239558,90.9061633964473,6.84033669502731));
#26266=CARTESIAN_POINT('Ctrl Pts',(21.1942540870207,94.2981359861555,6.68235352977868));
#26267=CARTESIAN_POINT('Ctrl Pts',(24.3913282372869,95.6056208028792,6.52437036453004));
#26268=CARTESIAN_POINT('Ctrl Pts',(27.2334543225922,93.6426844805108,6.36638719928141));
#26269=CARTESIAN_POINT('Ctrl Pts',(27.1427269710462,90.1897772675991,6.20840403403277));
#26270=CARTESIAN_POINT('Ctrl Pts',(24.2014389895034,88.3788038589624,6.05042086878413));
#26271=CARTESIAN_POINT('Ctrl Pts',(21.077438968569,89.8523789498237,5.8924377035355));
#26272=CARTESIAN_POINT('Ctrl Pts',(20.6043015565953,93.2739196359127,5.73445453828687));
#26273=CARTESIAN_POINT('Ctrl Pts',(23.2111785351691,95.5399717307178,5.57647137303823));
#26274=CARTESIAN_POINT('Ctrl Pts',(26.5335435065542,94.5951486388852,5.4184882077896));
#26275=CARTESIAN_POINT('Ctrl Pts',(27.5578980422048,91.2964371536349,5.26050504254097));
#26276=CARTESIAN_POINT('Ctrl Pts',(25.3551176148943,88.6358811841043,5.10252187729233));
#26277=CARTESIAN_POINT('Ctrl Pts',(21.9231992578101,89.0266958052455,4.94453871204369));
#26278=CARTESIAN_POINT('Ctrl Pts',(20.3750100595362,92.1143988161452,4.78655554679506));
#26279=CARTESIAN_POINT('Ctrl Pts',(22.1148104659795,95.0983381963849,4.62857238154642));
#26280=CARTESIAN_POINT('Ctrl Pts',(25.5645421252575,95.2719790790493,4.47058921629779));
#26281=CARTESIAN_POINT('Ctrl Pts',(27.5951806759185,92.4778232584365,4.31260605104916));
#26282=CARTESIAN_POINT('Ctrl Pts',(26.3648676419543,89.2502654310841,4.15462288580052));
#26283=CARTESIAN_POINT('Ctrl Pts',(22.9895389394378,88.5168107165773,3.99663972055189));
#26284=CARTESIAN_POINT('Ctrl Pts',(20.5307329066189,90.9427275616556,3.83865655530325));
#26285=CARTESIAN_POINT('Ctrl Pts',(21.2186705439485,94.3276266140658,3.68067339005462));
#26286=CARTESIAN_POINT('Ctrl Pts',(24.4293689246723,95.601288842286,3.52269022480598));
#26287=CARTESIAN_POINT('Ctrl Pts',(27.2506150476498,93.6084592491481,3.36470705955735));
#26288=CARTESIAN_POINT('Ctrl Pts',(27.1234423470096,90.1567020569745,3.20672389430872));
#26289=CARTESIAN_POINT('Ctrl Pts',(24.1632008787755,88.3768793413442,3.04874072906008));
#26290=CARTESIAN_POINT('Ctrl Pts',(21.0549305391037,89.8833500612564,2.89075756381145));
#26291=CARTESIAN_POINT('Ctrl Pts',(20.6179389343519,93.309695882881,2.73277439856281));
#26292=CARTESIAN_POINT('Ctrl Pts',(23.2485917195109,95.548100055872,2.57479123331418));
#26293=CARTESIAN_POINT('Ctrl Pts',(26.5607983477153,94.5682620509693,2.41680806806554));
#26294=CARTESIAN_POINT('Ctrl Pts',(27.5502716608787,91.2589111130016,2.25882490281691));
#26295=CARTESIAN_POINT('Ctrl Pts',(25.3195310914441,88.6217767625239,2.10084173756827));
#26296=CARTESIAN_POINT('Ctrl Pts',(21.891923244154,89.0487578560498,1.94285857231964));
#26297=CARTESIAN_POINT('Ctrl Pts',(20.376428363266,92.1527150135633,1.78487540707101));
#26298=CARTESIAN_POINT('Ctrl Pts',(22.1476051992024,95.1179528805984,1.62689224182237));
#26299=CARTESIAN_POINT('Ctrl Pts',(25.5990315417433,95.2555126520043,1.46890907657374));
#26300=CARTESIAN_POINT('Ctrl Pts',(27.5999506290771,92.4393708209745,1.3109259113251));
#26301=CARTESIAN_POINT('Ctrl Pts',(26.3358592338276,89.2264213520665,1.15294274607647));
#26302=CARTESIAN_POINT('Ctrl Pts',(22.9525239108491,88.5256846472501,0.994959580827833));
#26303=CARTESIAN_POINT('Ctrl Pts',(20.5204084922262,90.9835193506338,0.836976415579198));
#26304=CARTESIAN_POINT('Ctrl Pts',(21.0030718657858,93.2243470893905,0.731654305413442));
#26305=CARTESIAN_POINT('Ctrl Pts',(21.6639373423039,93.9973015569307,0.678993250330564));
#26306=CARTESIAN_POINT('Ctrl Pts',(23.254067145653,89.2098224301579,10.1070022498898));
#26307=CARTESIAN_POINT('Ctrl Pts',(22.3308555140066,89.4566360720578,10.0543411948069));
#26308=CARTESIAN_POINT('Ctrl Pts',(20.7643183622759,90.9350371728775,9.94901908464117));
#26309=CARTESIAN_POINT('Ctrl Pts',(21.3395004522086,94.1329828425986,9.79103591939255));
#26310=CARTESIAN_POINT('Ctrl Pts',(24.332574788482,95.3912246785046,9.6330527541439));
#26311=CARTESIAN_POINT('Ctrl Pts',(27.0217019181264,93.5759467792531,9.47506958889527));
#26312=CARTESIAN_POINT('Ctrl Pts',(26.9711632817165,90.3300443850485,9.31708642364663));
#26313=CARTESIAN_POINT('Ctrl Pts',(24.2251292456712,88.5994298644601,9.15910325839801));
#26314=CARTESIAN_POINT('Ctrl Pts',(21.2751640964776,89.9529639578542,9.00112009314937));
#26315=CARTESIAN_POINT('Ctrl Pts',(20.7965864827541,93.1633689675119,8.84313692790073));
#26316=CARTESIAN_POINT('Ctrl Pts',(23.2236787314268,95.3184903705681,8.6851537626521));
#26317=CARTESIAN_POINT('Ctrl Pts',(26.3548892997688,94.4636611608191,8.52717059740346));
#26318=CARTESIAN_POINT('Ctrl Pts',(27.3501503553349,91.3741908216577,8.36918743215484));
#26319=CARTESIAN_POINT('Ctrl Pts',(25.3067031200343,88.8523587823873,8.21120426690619));
#26320=CARTESIAN_POINT('Ctrl Pts',(22.0780352618005,89.1855408382048,8.05322110165756));
#26321=CARTESIAN_POINT('Ctrl Pts',(20.592653206264,92.0715353394405,7.89523793640893));
#26322=CARTESIAN_POINT('Ctrl Pts',(22.1978518818355,94.8926439048456,7.73725477116029));
#26323=CARTESIAN_POINT('Ctrl Pts',(25.4376599763359,95.0900261773889,7.57927160591166));
#26324=CARTESIAN_POINT('Ctrl Pts',(27.3734616151168,92.4846490120789,7.42128844066302));
#26325=CARTESIAN_POINT('Ctrl Pts',(26.2494183210864,89.439678761254,7.26330527541439));
#26326=CARTESIAN_POINT('Ctrl Pts',(23.0850758834993,88.7170072090857,7.10532211016575));
#26327=CARTESIAN_POINT('Ctrl Pts',(20.7506008228567,90.9721222003707,6.94733894491712));
#26328=CARTESIAN_POINT('Ctrl Pts',(21.3634417371065,94.1595574266086,6.78935577966849));
#26329=CARTESIAN_POINT('Ctrl Pts',(24.3677309811802,95.3882003629463,6.63137261441985));
#26330=CARTESIAN_POINT('Ctrl Pts',(27.038475676818,93.5436299204366,6.47338944917122));
#26331=CARTESIAN_POINT('Ctrl Pts',(26.9532192224532,90.2989344542175,6.31540628392258));
#26332=CARTESIAN_POINT('Ctrl Pts',(24.1892921343259,88.5971634982897,6.15742311867395));
#26333=CARTESIAN_POINT('Ctrl Pts',(21.2536706190734,89.9818813958839,5.99943995342532));
#26334=CARTESIAN_POINT('Ctrl Pts',(20.8090635905992,93.1971017499447,5.84145678817668));
#26335=CARTESIAN_POINT('Ctrl Pts',(23.2587447988691,95.3265099572479,5.68347362292804));
#26336=CARTESIAN_POINT('Ctrl Pts',(26.3807697752333,94.4386600923617,5.52549045767941));
#26337=CARTESIAN_POINT('Ctrl Pts',(27.3433553046672,91.3388622870417,5.36750729243078));
#26338=CARTESIAN_POINT('Ctrl Pts',(25.2734034568897,88.8387389533836,5.20952412718214));
#26339=CARTESIAN_POINT('Ctrl Pts',(22.0484312097279,89.205987289686,5.05154096193351));
#26340=CARTESIAN_POINT('Ctrl Pts',(20.5935984665529,92.1075005197647,4.89355779668487));
#26341=CARTESIAN_POINT('Ctrl Pts',(22.2284881820378,94.9115071094384,4.73557463143624));
#26342=CARTESIAN_POINT('Ctrl Pts',(25.4701995818333,95.0746773743747,4.5775914661876));
#26343=CARTESIAN_POINT('Ctrl Pts',(27.3783897800007,92.4490103164387,4.41960830093897));
#26344=CARTESIAN_POINT('Ctrl Pts',(26.2222651356991,89.4160755737354,4.26162513569033));
#26345=CARTESIAN_POINT('Ctrl Pts',(23.0504701633055,88.726848484766,4.1036419704417));
#26346=CARTESIAN_POINT('Ctrl Pts',(20.7399311609349,91.0064815311496,3.94565880519306));
#26347=CARTESIAN_POINT('Ctrl Pts',(21.3863858714865,94.1872697573423,3.78767563994443));
#26348=CARTESIAN_POINT('Ctrl Pts',(24.4034777992324,95.3841296213856,3.6296924746958));
#26349=CARTESIAN_POINT('Ctrl Pts',(27.0546016029892,93.5114684848159,3.47170930944716));
#26350=CARTESIAN_POINT('Ctrl Pts',(26.9350974692983,90.267853692604,3.31372614419853));
#26351=CARTESIAN_POINT('Ctrl Pts',(24.1533597976412,88.5953550298875,3.15574297894989));
#26352=CARTESIAN_POINT('Ctrl Pts',(21.2325194573032,90.0109849363652,2.99775981370126));
#26353=CARTESIAN_POINT('Ctrl Pts',(20.8218786287828,93.2307206742826,2.83977664845262));
#26354=CARTESIAN_POINT('Ctrl Pts',(23.2939019525734,95.3341481410013,2.68179348320399));
#26355=CARTESIAN_POINT('Ctrl Pts',(26.4063811380923,94.4133947769235,2.52381031795535));
#26356=CARTESIAN_POINT('Ctrl Pts',(27.3361887973193,91.3035990823277,2.36582715270672));
#26357=CARTESIAN_POINT('Ctrl Pts',(25.2399628156627,88.8254850343136,2.20784398745808));
#26358=CARTESIAN_POINT('Ctrl Pts',(22.0190411527544,89.2267189896149,2.04986082220945));
#26359=CARTESIAN_POINT('Ctrl Pts',(20.5949312459756,92.1435062344795,1.89187765696082));
#26360=CARTESIAN_POINT('Ctrl Pts',(22.259305379154,94.9299390200038,1.73389449171218));
#26361=CARTESIAN_POINT('Ctrl Pts',(25.502609272104,95.0592038797561,1.57591132646355));
#26362=CARTESIAN_POINT('Ctrl Pts',(27.382872102992,92.4128765770114,1.41792816121491));
#26363=CARTESIAN_POINT('Ctrl Pts',(26.1950059466948,89.3936693026388,1.25994499596628));
#26364=CARTESIAN_POINT('Ctrl Pts',(23.0156871563963,88.7351873137138,1.10196183071764));
#26365=CARTESIAN_POINT('Ctrl Pts',(20.7302293130409,91.04481355822,0.94397866546901));
#26366=CARTESIAN_POINT('Ctrl Pts',(21.1837878836398,93.1505184486768,0.838656555303253));
#26367=CARTESIAN_POINT('Ctrl Pts',(21.8048028959809,93.8768634390788,0.785995500220375));
#26368=CARTESIAN_POINT('Ctrl Pts',(23.3019335738389,89.3888678140614,10.2140044997796));
#26369=CARTESIAN_POINT('Ctrl Pts',(22.4379643297735,89.6198434520493,10.1613434446967));
#26370=CARTESIAN_POINT('Ctrl Pts',(20.9719516925979,91.0033757188849,10.056021334531));
#26371=CARTESIAN_POINT('Ctrl Pts',(21.5102244118799,93.9961095711478,9.89803816928235));
#26372=CARTESIAN_POINT('Ctrl Pts',(24.3112335013453,95.1736101685792,9.74005500403372));
#26373=CARTESIAN_POINT('Ctrl Pts',(26.8277996425793,93.4748184499478,9.58207183878509));
#26374=CARTESIAN_POINT('Ctrl Pts',(26.780504064839,90.4372052508703,9.42408867353644));
#26375=CARTESIAN_POINT('Ctrl Pts',(24.21068272705,88.8176440713225,9.26610550828783));
#26376=CARTESIAN_POINT('Ctrl Pts',(21.4500165129308,90.0843220326922,9.10812234303918));
#26377=CARTESIAN_POINT('Ctrl Pts',(21.0021491713788,93.0887157104357,8.95013917779055));
#26378=CARTESIAN_POINT('Ctrl Pts',(23.2734951807691,95.1055432130824,8.79215601254191));
#26379=CARTESIAN_POINT('Ctrl Pts',(26.2037763156761,94.305568298517,8.63417284729328));
#26380=CARTESIAN_POINT('Ctrl Pts',(27.1351715801527,91.4143489269332,8.47618968204464));
#26381=CARTESIAN_POINT('Ctrl Pts',(25.2228521263544,89.054342568756,8.31820651679601));
#26382=CARTESIAN_POINT('Ctrl Pts',(22.2013675249939,89.3661443691598,8.16022335154737));
#26383=CARTESIAN_POINT('Ctrl Pts',(20.8113022705282,92.0669449246757,8.00224018629874));
#26384=CARTESIAN_POINT('Ctrl Pts',(22.3134955258657,94.707023267637,7.8442570210501));
#26385=CARTESIAN_POINT('Ctrl Pts',(25.3454054957724,94.8917395417344,7.68627385580147));
#26386=CARTESIAN_POINT('Ctrl Pts',(27.1569869589906,92.4535491389511,7.52829069055284));
#26387=CARTESIAN_POINT('Ctrl Pts',(26.105073397949,89.603974289991,7.37030752530419));
#26388=CARTESIAN_POINT('Ctrl Pts',(23.1437864621564,88.9276764908387,7.21232436005557));
#26389=CARTESIAN_POINT('Ctrl Pts',(20.9591144061554,91.038081004294,7.05434119480692));
#26390=CARTESIAN_POINT('Ctrl Pts',(21.5326293871924,94.0209788670617,6.8963580295583));
#26391=CARTESIAN_POINT('Ctrl Pts',(24.3441337250736,95.1707799230134,6.73837486430966));
#26392=CARTESIAN_POINT('Ctrl Pts',(26.8434970310438,93.4445753603625,6.58039169906103));
#26393=CARTESIAN_POINT('Ctrl Pts',(26.7637114738602,90.4080916408359,6.42240853381239));
#26394=CARTESIAN_POINT('Ctrl Pts',(24.1771452791484,88.8155231376169,6.26442536856376));
#26395=CARTESIAN_POINT('Ctrl Pts',(21.4299022695778,90.1113838419441,6.10644220331513));
#26396=CARTESIAN_POINT('Ctrl Pts',(21.0138256246031,93.1202838639768,5.94845903806649));
#26397=CARTESIAN_POINT('Ctrl Pts',(23.3063110625691,95.113048183778,5.79047587281785));
#26398=CARTESIAN_POINT('Ctrl Pts',(26.2279960439124,94.2821715458382,5.63249270756922));
#26399=CARTESIAN_POINT('Ctrl Pts',(27.1288125671295,91.3812874204487,5.47450954232058));
#26400=CARTESIAN_POINT('Ctrl Pts',(25.1916892988851,89.0415967226626,5.31652637707195));
#26401=CARTESIAN_POINT('Ctrl Pts',(22.1736631616456,89.3852787741264,5.15854321182332));
#26402=CARTESIAN_POINT('Ctrl Pts',(20.8121868735697,92.1006022233842,5.00056004657468));
#26403=CARTESIAN_POINT('Ctrl Pts',(22.3421658980961,94.7246760224918,4.84257688132605));
#26404=CARTESIAN_POINT('Ctrl Pts',(25.375857038409,94.8773756697003,4.68459371607741));
#26405=CARTESIAN_POINT('Ctrl Pts',(27.1615988840828,92.4201973744409,4.52661055082878));
#26406=CARTESIAN_POINT('Ctrl Pts',(26.0796626294438,89.5818857163869,4.36862738558014));
#26407=CARTESIAN_POINT('Ctrl Pts',(23.1114013871733,88.9368862529545,4.21064422033151));
#26408=CARTESIAN_POINT('Ctrl Pts',(20.9491294152507,91.0702355006436,4.05266105508287));
#26409=CARTESIAN_POINT('Ctrl Pts',(21.5541011990246,94.0469129006186,3.89467788983424));
#26410=CARTESIAN_POINT('Ctrl Pts',(24.3775866737926,95.1669704004854,3.7366947245856));
#26411=CARTESIAN_POINT('Ctrl Pts',(26.8585881583285,93.4144777204836,3.57871155933697));
#26412=CARTESIAN_POINT('Ctrl Pts',(26.7467525915869,90.3790053282334,3.42072839408834));
#26413=CARTESIAN_POINT('Ctrl Pts',(24.1435187165069,88.8138307184307,3.2627452288397));
#26414=CARTESIAN_POINT('Ctrl Pts',(21.4101083755027,90.138619811474,3.10476206359106));
#26415=CARTESIAN_POINT('Ctrl Pts',(21.0258183232138,93.1517454656843,2.94677889834244));
#26416=CARTESIAN_POINT('Ctrl Pts',(23.3392121856357,95.1201962261306,2.78879573309379));
#26417=CARTESIAN_POINT('Ctrl Pts',(26.2519639284692,94.2585275028778,2.63081256784517));
#26418=CARTESIAN_POINT('Ctrl Pts',(27.1221059337601,91.3482870516537,2.47282940259653));
#26419=CARTESIAN_POINT('Ctrl Pts',(25.1603945398812,89.0291933061033,2.3148462373479));
#26420=CARTESIAN_POINT('Ctrl Pts',(22.1461590613549,89.4046801231798,2.15686307209926));
#26421=CARTESIAN_POINT('Ctrl Pts',(20.8134341286852,92.134297455396,1.99887990685063));
#26422=CARTESIAN_POINT('Ctrl Pts',(22.3710055591055,94.741925159409,1.84089674160199));
#26423=CARTESIAN_POINT('Ctrl Pts',(25.4061870024647,94.8628951075081,1.68291357635336));
#26424=CARTESIAN_POINT('Ctrl Pts',(27.1657935769071,92.3863823330482,1.52493041110472));
#26425=CARTESIAN_POINT('Ctrl Pts',(26.0541526595619,89.560917253211,1.36694724585609));
#26426=CARTESIAN_POINT('Ctrl Pts',(23.0788504019435,88.9446899801776,1.20896408060745));
#26427=CARTESIAN_POINT('Ctrl Pts',(20.9400501338557,91.106107765806,1.05098091535882));
#26428=CARTESIAN_POINT('Ctrl Pts',(21.3645039014938,93.076689807963,0.945658805193063));
#26429=CARTESIAN_POINT('Ctrl Pts',(21.945668449658,93.7564253212269,0.892997750110186));
#26430=CARTESIAN_POINT('Ctrl Pts',(23.3498000020249,89.5679131979649,10.3210067496694));
#26431=CARTESIAN_POINT('Ctrl Pts',(22.5450731455404,89.7830508320407,10.2683456945866));
#26432=CARTESIAN_POINT('Ctrl Pts',(21.1795850229198,91.0717142648921,10.1630235844208));
#26433=CARTESIAN_POINT('Ctrl Pts',(21.6809483715512,93.859236299697,10.0050404191722));
#26434=CARTESIAN_POINT('Ctrl Pts',(24.2898922142086,94.9559956586539,9.84705725392353));
#26435=CARTESIAN_POINT('Ctrl Pts',(26.6338973670321,93.3736901206426,9.68907408867489));
#26436=CARTESIAN_POINT('Ctrl Pts',(26.5898448479616,90.5443661166922,9.53109092342625));
#26437=CARTESIAN_POINT('Ctrl Pts',(24.1962362084288,89.0358582781851,9.37310775817764));
#26438=CARTESIAN_POINT('Ctrl Pts',(21.6248689293839,90.2156801075301,9.21512459292898));
#26439=CARTESIAN_POINT('Ctrl Pts',(21.2077118600035,93.0140624533595,9.05714142768036));
#26440=CARTESIAN_POINT('Ctrl Pts',(23.3233116301114,94.8925960555965,8.89915826243172));
#26441=CARTESIAN_POINT('Ctrl Pts',(26.0526633315834,94.1474754362151,8.74117509718309));
#26442=CARTESIAN_POINT('Ctrl Pts',(26.9201928049705,91.4545070322085,8.58319193193445));
#26443=CARTESIAN_POINT('Ctrl Pts',(25.1390011326746,89.2563263551249,8.42520876668581));
#26444=CARTESIAN_POINT('Ctrl Pts',(22.3246997881873,89.5467479001147,8.26722560143719));
#26445=CARTESIAN_POINT('Ctrl Pts',(21.0299513347924,92.0623545099109,8.10924243618855));
#26446=CARTESIAN_POINT('Ctrl Pts',(22.4291391698959,94.5214026304284,7.95125927093991));
#26447=CARTESIAN_POINT('Ctrl Pts',(25.2531510152088,94.69345290608,7.79327610569128));
#26448=CARTESIAN_POINT('Ctrl Pts',(26.9405123028645,92.4224492658233,7.63529294044264));
#26449=CARTESIAN_POINT('Ctrl Pts',(25.9607284748115,89.7682698187282,7.47730977519401));
#26450=CARTESIAN_POINT('Ctrl Pts',(23.2024970408135,89.1383457725916,7.31932660994538));
#26451=CARTESIAN_POINT('Ctrl Pts',(21.1676279894541,91.1040398082174,7.16134344469674));
#26452=CARTESIAN_POINT('Ctrl Pts',(21.7018170372782,93.8824003075146,7.00336027944811));
#26453=CARTESIAN_POINT('Ctrl Pts',(24.3205364689669,94.9533594830808,6.84537711419947));
#26454=CARTESIAN_POINT('Ctrl Pts',(26.6485183852695,93.3455208002881,6.68739394895084));
#26455=CARTESIAN_POINT('Ctrl Pts',(26.5742037252672,90.5172488274544,6.5294107837022));
#26456=CARTESIAN_POINT('Ctrl Pts',(24.1649984239709,89.0338827769442,6.37142761845357));
#26457=CARTESIAN_POINT('Ctrl Pts',(21.6061339200822,90.2408862880042,6.21344445320494));
#26458=CARTESIAN_POINT('Ctrl Pts',(21.218587658607,93.0434659780088,6.0554612879563));
#26459=CARTESIAN_POINT('Ctrl Pts',(23.3538773262692,94.8995864103082,5.89747812270766));
#26460=CARTESIAN_POINT('Ctrl Pts',(26.0752223125915,94.1256829993147,5.73949495745903));
#26461=CARTESIAN_POINT('Ctrl Pts',(26.9142698295919,91.4237125538557,5.5815117922104));
#26462=CARTESIAN_POINT('Ctrl Pts',(25.1099751408805,89.2444544919418,5.42352862696176));
#26463=CARTESIAN_POINT('Ctrl Pts',(22.2988951135634,89.5645702585668,5.26554546171313));
#26464=CARTESIAN_POINT('Ctrl Pts',(21.0307752805864,92.0937039270037,5.10756229646449));
#26465=CARTESIAN_POINT('Ctrl Pts',(22.4558436141543,94.5378449355453,4.94957913121586));
#26466=CARTESIAN_POINT('Ctrl Pts',(25.2815144949848,94.6800739650258,4.79159596596722));
#26467=CARTESIAN_POINT('Ctrl Pts',(26.9448079881649,92.3913844324431,4.63361280071859));
#26468=CARTESIAN_POINT('Ctrl Pts',(25.9370601231886,89.7476958590382,4.47562963546995));
#26469=CARTESIAN_POINT('Ctrl Pts',(23.172332611041,89.1469240211431,4.31764647022132));
#26470=CARTESIAN_POINT('Ctrl Pts',(21.1583276695667,91.1339894701376,4.15966330497269));
#26471=CARTESIAN_POINT('Ctrl Pts',(21.7218165265627,93.9065560438949,4.00168013972405));
#26472=CARTESIAN_POINT('Ctrl Pts',(24.3516955483528,94.9498111795851,3.84369697447542));
#26473=CARTESIAN_POINT('Ctrl Pts',(26.6625747136679,93.3174869561512,3.68571380922678));
#26474=CARTESIAN_POINT('Ctrl Pts',(26.5584077138756,90.4901569638631,3.52773064397815));
#26475=CARTESIAN_POINT('Ctrl Pts',(24.1336776353725,89.0323064069738,3.36974747872951));
#26476=CARTESIAN_POINT('Ctrl Pts',(21.5876972937022,90.266254686583,3.21176431348088));
#26477=CARTESIAN_POINT('Ctrl Pts',(21.2297580176447,93.0727702570857,3.05378114823224));
#26478=CARTESIAN_POINT('Ctrl Pts',(23.3845224186982,94.90624431126,2.89579798298361));
#26479=CARTESIAN_POINT('Ctrl Pts',(26.0975467188461,94.103660228832,2.73781481773498));
#26480=CARTESIAN_POINT('Ctrl Pts',(26.9080230702008,91.3929750209798,2.57983165248634));
#26481=CARTESIAN_POINT('Ctrl Pts',(25.0808262640998,89.232901577893,2.42184848723771));
#26482=CARTESIAN_POINT('Ctrl Pts',(22.2732769699553,89.5826412567449,2.26386532198907));
#26483=CARTESIAN_POINT('Ctrl Pts',(21.0319370113949,92.1250886763122,2.10588215674044));
#26484=CARTESIAN_POINT('Ctrl Pts',(22.4827057390571,94.5539112988145,1.9478989914918));
#26485=CARTESIAN_POINT('Ctrl Pts',(25.3097647328254,94.6665863352599,1.78991582624317));
#26486=CARTESIAN_POINT('Ctrl Pts',(26.948715050822,92.3598880890851,1.63193266099453));
#26487=CARTESIAN_POINT('Ctrl Pts',(25.9132993724291,89.7281652037832,1.4739494957459));
#26488=CARTESIAN_POINT('Ctrl Pts',(23.1420136474907,89.1541926466413,1.31596633049726));
#26489=CARTESIAN_POINT('Ctrl Pts',(21.1498709546704,91.1674019733922,1.15798316524863));
#26490=CARTESIAN_POINT('Ctrl Pts',(21.5452199193479,93.0028611672493,1.05266105508287));
#26491=CARTESIAN_POINT('Ctrl Pts',(22.086534003335,93.635987203375,0.999999999999996));
#26492=CARTESIAN_POINT('Ctrl Pts',(21.4850510509789,92.0017493960693,9.11258330249198));
#26493=CARTESIAN_POINT('Ctrl Pts',(21.4831440162074,92.2947752212131,9.09410267755477));
#26494=CARTESIAN_POINT('Ctrl Pts',(21.5304974072668,92.5872051529597,9.07562205261756));
#26495=CARTESIAN_POINT('Ctrl Pts',(21.6298379999182,92.8607543294275,9.05714142768035));
#26496=CARTESIAN_POINT('Ctrl Pts',(21.9129117833728,93.6402403207719,9.00448037259747));
#26497=CARTESIAN_POINT('Ctrl Pts',(22.6181117067421,94.2664181881842,8.95181931751459));
#26498=CARTESIAN_POINT('Ctrl Pts',(23.4256036186721,94.4553203519934,8.89915826243172));
#26499=CARTESIAN_POINT('Ctrl Pts',(24.2330955306021,94.6442225158027,8.84649720734884));
#26500=CARTESIAN_POINT('Ctrl Pts',(25.1428794310927,94.3958489760089,8.79383615226596));
#26501=CARTESIAN_POINT('Ctrl Pts',(25.7423596269026,93.8228341387776,8.74117509718308));
#26502=CARTESIAN_POINT('Ctrl Pts',(26.3418398227124,93.2498193015462,8.6885140421002));
#26503=CARTESIAN_POINT('Ctrl Pts',(26.6310163138414,92.3521631668773,8.63585298701732));
#26504=CARTESIAN_POINT('Ctrl Pts',(26.47873928069,91.5369716533623,8.58319193193445));
#26505=CARTESIAN_POINT('Ctrl Pts',(26.3264622475385,90.7217801398473,8.53053087685157));
#26506=CARTESIAN_POINT('Ctrl Pts',(25.7327316901066,89.9890532474861,8.47786982176869));
#26507=CARTESIAN_POINT('Ctrl Pts',(24.9668161873094,89.6710933921371,8.42520876668581));
#26508=CARTESIAN_POINT('Ctrl Pts',(24.2009006845121,89.3531335367881,8.37254771160293));
#26509=CARTESIAN_POINT('Ctrl Pts',(23.2628002363497,89.4499407184514,8.31988665652006));
#26510=CARTESIAN_POINT('Ctrl Pts',(22.5779586033693,89.9176120775824,8.26722560143718));
#26511=CARTESIAN_POINT('Ctrl Pts',(21.9075993003968,90.3753936014114,8.21567816845545));
#26512=CARTESIAN_POINT('Ctrl Pts',(21.4799007520941,91.1885198389857,8.16413073547371));
#26513=CARTESIAN_POINT('Ctrl Pts',(21.4784369335473,92.0003195913806,8.11258330249198));
#26514=CARTESIAN_POINT('Ctrl Pts',(23.2062007174671,89.0307770462543,10.));
#26515=CARTESIAN_POINT('Ctrl Pts',(23.1131475235312,89.064816320262,10.));
#26516=CARTESIAN_POINT('Ctrl Pts',(23.0221596064779,89.1036239095806,10.));
#26517=CARTESIAN_POINT('Ctrl Pts',(22.9334454653316,89.1468715855098,10.));
#26518=CARTESIAN_POINT('Ctrl Pts',(22.8427656611047,89.1910775118239,10.));
#26519=CARTESIAN_POINT('Ctrl Pts',(22.7544608424803,89.2399230814568,10.));
#26520=CARTESIAN_POINT('Ctrl Pts',(22.6687825963672,89.2931033001226,10.));
#26521=CARTESIAN_POINT('Ctrl Pts',(22.586330110816,89.3442812993241,10.));
#26522=CARTESIAN_POINT('Ctrl Pts',(22.5063098561179,89.3994745706755,10.));
#26523=CARTESIAN_POINT('Ctrl Pts',(22.4289790559017,89.458441358607,10.));
#26524=CARTESIAN_POINT('Ctrl Pts',(22.3613146057126,89.5100372980471,10.));
#26525=CARTESIAN_POINT('Ctrl Pts',(22.2957095595976,89.5645230341413,10.));
#26526=CARTESIAN_POINT('Ctrl Pts',(22.2323608843388,89.6217493205767,10.));
#26527=CARTESIAN_POINT('Ctrl Pts',(22.218262116408,89.6344855005946,10.));
#26528=CARTESIAN_POINT('Ctrl Pts',(22.2042725067628,89.6473601252669,10.));
#26529=CARTESIAN_POINT('Ctrl Pts',(22.1904136996835,89.6603531214548,10.));
#26530=CARTESIAN_POINT('Ctrl Pts',(22.1179829795791,89.7282588268171,10.));
#26531=CARTESIAN_POINT('Ctrl Pts',(22.0490179328543,89.799486285336,10.));
#26532=CARTESIAN_POINT('Ctrl Pts',(21.9837585062309,89.8737448951122,10.));
#26533=CARTESIAN_POINT('Ctrl Pts',(21.918858759645,89.9475942254794,10.));
#26534=CARTESIAN_POINT('Ctrl Pts',(21.8576234120103,90.0244421833075,10.));
#26535=CARTESIAN_POINT('Ctrl Pts',(21.800332072969,90.1040297128831,10.));
#26536=CARTESIAN_POINT('Ctrl Pts',(21.7451392509027,90.1807020412326,10.));
#26537=CARTESIAN_POINT('Ctrl Pts',(21.6936066323894,90.2599176592597,10.));
#26538=CARTESIAN_POINT('Ctrl Pts',(21.6460291433951,90.341458559806,10.));
#26539=CARTESIAN_POINT('Ctrl Pts',(21.626040380651,90.3757163936978,10.));
#26540=CARTESIAN_POINT('Ctrl Pts',(21.606750309037,90.4103847699114,10.));
#26541=CARTESIAN_POINT('Ctrl Pts',(21.5881834031431,90.4454478211808,10.));
#26542=CARTESIAN_POINT('Ctrl Pts',(21.5751468384104,90.4700669871428,10.));
#26543=CARTESIAN_POINT('Ctrl Pts',(21.5624668273574,90.4948807308745,10.));
#26544=CARTESIAN_POINT('Ctrl Pts',(21.5501523284354,90.5198835657242,10.));
#26545=CARTESIAN_POINT('Ctrl Pts',(21.5423998388932,90.5356238907609,10.));
#26546=CARTESIAN_POINT('Ctrl Pts',(21.5347913334218,90.551441280599,10.));
#26547=CARTESIAN_POINT('Ctrl Pts',(21.5273387128466,90.5673132394905,10.));
#26548=CARTESIAN_POINT('Ctrl Pts',(21.4852181501849,90.6570180396091,10.));
#26549=CARTESIAN_POINT('Ctrl Pts',(21.4479997999212,90.748607534526,10.));
#26550=CARTESIAN_POINT('Ctrl Pts',(21.4159753088276,90.8418092601306,10.));
#26551=CARTESIAN_POINT('Ctrl Pts',(21.3861128448267,90.9287187809577,10.));
#26552=CARTESIAN_POINT('Ctrl Pts',(21.360766797266,91.0170309840337,10.));
#26553=CARTESIAN_POINT('Ctrl Pts',(21.340224189409,91.1065336320268,10.));
#26554=CARTESIAN_POINT('Ctrl Pts',(21.3387369151257,91.1130135778824,10.));
#26555=CARTESIAN_POINT('Ctrl Pts',(21.3372748417258,91.1194997648427,10.));
#26556=CARTESIAN_POINT('Ctrl Pts',(21.3358380889382,91.125992112682,10.));
#26557=CARTESIAN_POINT('Ctrl Pts',(21.3152524900323,91.219013591207,10.));
#26558=CARTESIAN_POINT('Ctrl Pts',(21.2998606756254,91.3133008086048,10.));
#26559=CARTESIAN_POINT('Ctrl Pts',(21.2895856382541,91.4084457389737,10.));
#26560=CARTESIAN_POINT('Ctrl Pts',(21.2837680062684,91.4623159265151,10.));
#26561=CARTESIAN_POINT('Ctrl Pts',(21.2795916051018,91.5164608839292,10.));
#26562=CARTESIAN_POINT('Ctrl Pts',(21.2770493497667,91.5708038567304,10.));
#26563=CARTESIAN_POINT('Ctrl Pts',(21.2764020101031,91.5846413187856,10.));
#26564=CARTESIAN_POINT('Ctrl Pts',(21.2758607757032,91.5984902137829,10.));
#26565=CARTESIAN_POINT('Ctrl Pts',(21.2754257103763,91.612337039112,10.));
#26566=CARTESIAN_POINT('Ctrl Pts',(21.2724969038989,91.7055521707492,10.));
#26567=CARTESIAN_POINT('Ctrl Pts',(21.2743674875468,91.7988245803011,10.));
#26568=CARTESIAN_POINT('Ctrl Pts',(21.28090259303,91.8917789957835,10.));
#26569=CARTESIAN_POINT('Ctrl Pts',(21.287448136198,91.9848818754176,10.));
#26570=CARTESIAN_POINT('Ctrl Pts',(21.2986734919875,92.0776667240288,10.));
#26571=CARTESIAN_POINT('Ctrl Pts',(21.3144940516725,92.1697443145829,10.));
#26572=CARTESIAN_POINT('Ctrl Pts',(21.330087444504,92.2604997662911,10.));
#26573=CARTESIAN_POINT('Ctrl Pts',(21.3501454854448,92.3505689686558,10.));
#26574=CARTESIAN_POINT('Ctrl Pts',(21.3746301441159,92.4395539722668,10.));
#26575=CARTESIAN_POINT('Ctrl Pts',(21.3838722153142,92.4731425858555,10.));
#26576=CARTESIAN_POINT('Ctrl Pts',(21.3937453933244,92.5065763996315,10.));
#26577=CARTESIAN_POINT('Ctrl Pts',(21.4042490564703,92.5398326835533,10.));
#26578=CARTESIAN_POINT('Ctrl Pts',(21.4119449767332,92.5641992027144,10.));
#26579=CARTESIAN_POINT('Ctrl Pts',(21.4199793784173,92.5884704022233,10.));
#26580=CARTESIAN_POINT('Ctrl Pts',(21.4283522639682,92.6126370452986,10.));
#26581=CARTESIAN_POINT('Ctrl Pts',(21.4335197893842,92.6275520637297,10.));
#26582=CARTESIAN_POINT('Ctrl Pts',(21.4388132538925,92.6424185688738,10.));
#26583=CARTESIAN_POINT('Ctrl Pts',(21.4442314703781,92.6572324707066,10.));
#26584=CARTESIAN_POINT('Ctrl Pts',(21.4759375175441,92.7439197176034,10.));
#26585=CARTESIAN_POINT('Ctrl Pts',(21.511920335298,92.8288327924596,10.));
#26586=CARTESIAN_POINT('Ctrl Pts',(21.552119621785,92.9115708703277,10.));
#26587=CARTESIAN_POINT('Ctrl Pts',(21.5822690866502,92.9736244287288,10.));
#26588=CARTESIAN_POINT('Ctrl Pts',(21.6147913043088,93.0344540664617,10.));
#26589=CARTESIAN_POINT('Ctrl Pts',(21.6496759248426,93.0938756896316,10.));
#26590=CARTESIAN_POINT('Ctrl Pts',(21.6654547887392,93.1207530266977,10.));
#26591=CARTESIAN_POINT('Ctrl Pts',(21.6817171403762,93.1473420998653,10.));
#26592=CARTESIAN_POINT('Ctrl Pts',(21.6984628023229,93.1736248041848,10.));
#26593=CARTESIAN_POINT('Ctrl Pts',(21.7075848153972,93.1879420150059,10.));
#26594=CARTESIAN_POINT('Ctrl Pts',(21.7168450674866,93.2021601541862,10.));
#26595=CARTESIAN_POINT('Ctrl Pts',(21.7262428789321,93.2162762091593,10.));
#26596=CARTESIAN_POINT('Ctrl Pts',(21.7738179410717,93.2877366972111,10.));
#26597=CARTESIAN_POINT('Ctrl Pts',(21.8249182080518,93.3565879238228,10.));
#26598=CARTESIAN_POINT('Ctrl Pts',(21.8795126224576,93.4224764000789,10.));
#26599=CARTESIAN_POINT('Ctrl Pts',(21.9256431150068,93.4781500050822,10.));
#26600=CARTESIAN_POINT('Ctrl Pts',(21.9742689995204,93.5317079390157,10.));
#26601=CARTESIAN_POINT('Ctrl Pts',(22.0253878321675,93.58291282293,10.));
#26602=CARTESIAN_POINT('Ctrl Pts',(22.0442196215672,93.6017763129624,10.));
#26603=CARTESIAN_POINT('Ctrl Pts',(22.0633898808657,93.6203202151646,10.));
#26604=CARTESIAN_POINT('Ctrl Pts',(22.0828884583321,93.6385402287508,10.));
#26605=CARTESIAN_POINT('Origin',(24.,92.,5.));
#26606=CARTESIAN_POINT('Origin',(92.,-24.,1.));
#26607=CARTESIAN_POINT('Ctrl Pts',(90.0865340033349,-22.3640127966251,1.));
#26608=CARTESIAN_POINT('Ctrl Pts',(90.0243936079936,-22.4224095095248,1.));
#26609=CARTESIAN_POINT('Ctrl Pts',(89.9656285062059,-22.4840599082556,1.));
#26610=CARTESIAN_POINT('Ctrl Pts',(89.9102507400287,-22.5485875658771,1.));
#26611=CARTESIAN_POINT('Ctrl Pts',(89.8535182657226,-22.6146937657251,1.));
#26612=CARTESIAN_POINT('Ctrl Pts',(89.8003404147793,-22.6838202104461,1.00000000000001));
#26613=CARTESIAN_POINT('Ctrl Pts',(89.7507590224199,-22.7556084412598,1.00000000000001));
#26614=CARTESIAN_POINT('Ctrl Pts',(89.7378150803961,-22.7743498007381,1.00000000000001));
#26615=CARTESIAN_POINT('Ctrl Pts',(89.7251164248241,-22.793272790225,1.));
#26616=CARTESIAN_POINT('Ctrl Pts',(89.7126641760334,-22.8123714654963,1.));
#26617=CARTESIAN_POINT('Ctrl Pts',(89.7025035055584,-22.8279554254061,1.));
#26618=CARTESIAN_POINT('Ctrl Pts',(89.6925064619188,-22.8436572534766,1.));
#26619=CARTESIAN_POINT('Ctrl Pts',(89.6826824797406,-22.8594591610939,1.));
#26620=CARTESIAN_POINT('Ctrl Pts',(89.6352350825432,-22.9357784554084,1.));
#26621=CARTESIAN_POINT('Ctrl Pts',(89.5917712590377,-23.0145049677974,1.00000000000001));
#26622=CARTESIAN_POINT('Ctrl Pts',(89.5523257642681,-23.09524621402,1.00000000000001));
#26623=CARTESIAN_POINT('Ctrl Pts',(89.5204848605231,-23.1604215721755,1.00000000000001));
#26624=CARTESIAN_POINT('Ctrl Pts',(89.4912627688458,-23.2269108039903,1.));
#26625=CARTESIAN_POINT('Ctrl Pts',(89.4646949471924,-23.2945252983029,1.));
#26626=CARTESIAN_POINT('Ctrl Pts',(89.453969916764,-23.3218202537706,1.00000000000001));
#26627=CARTESIAN_POINT('Ctrl Pts',(89.4436776173418,-23.3492987388173,1.));
#26628=CARTESIAN_POINT('Ctrl Pts',(89.4338211719337,-23.3769489123748,1.));
#26629=CARTESIAN_POINT('Ctrl Pts',(89.4286030055382,-23.3915873748747,1.));
#26630=CARTESIAN_POINT('Ctrl Pts',(89.4235075587072,-23.4062726291406,1.00000000000001));
#26631=CARTESIAN_POINT('Ctrl Pts',(89.41853905105,-23.4209911021932,1.00000000000001));
#26632=CARTESIAN_POINT('Ctrl Pts',(89.3890249549379,-23.5084222703165,1.00000000000001));
#26633=CARTESIAN_POINT('Ctrl Pts',(89.3639471428126,-23.5971333184058,1.));
#26634=CARTESIAN_POINT('Ctrl Pts',(89.3433383854818,-23.6867265557536,1.));
#26635=CARTESIAN_POINT('Ctrl Pts',(89.3224107214163,-23.7777061885211,1.));
#26636=CARTESIAN_POINT('Ctrl Pts',(89.3060909932886,-23.8695963304555,1.));
#26637=CARTESIAN_POINT('Ctrl Pts',(89.294455361361,-23.962013678881,1.));
#26638=CARTESIAN_POINT('Ctrl Pts',(89.282910896282,-24.0537069240991,1.));
#26639=CARTESIAN_POINT('Ctrl Pts',(89.275977070024,-24.1459200764499,1.));
#26640=CARTESIAN_POINT('Ctrl Pts',(89.2737752209874,-24.2382979315414,1.));
#26641=CARTESIAN_POINT('Ctrl Pts',(89.2726800380544,-24.2842459727554,1.));
#26642=CARTESIAN_POINT('Ctrl Pts',(89.272756305641,-24.330234973425,1.00000000000001));
#26643=CARTESIAN_POINT('Ctrl Pts',(89.2740237450201,-24.3762219172853,1.00000000000001));
#26644=CARTESIAN_POINT('Ctrl Pts',(89.2744405290818,-24.3913442383727,1.00000000000001));
#26645=CARTESIAN_POINT('Ctrl Pts',(89.2749862320744,-24.4064681891601,1.));
#26646=CARTESIAN_POINT('Ctrl Pts',(89.2756613705299,-24.4215864117119,1.));
#26647=CARTESIAN_POINT('Ctrl Pts',(89.2799353263961,-24.5172921376071,1.));
#26648=CARTESIAN_POINT('Ctrl Pts',(89.2893763302497,-24.6124306981363,1.00000000000001));
#26649=CARTESIAN_POINT('Ctrl Pts',(89.3040485582739,-24.7066037689229,1.00000000000001));
#26650=CARTESIAN_POINT('Ctrl Pts',(89.3082030634041,-24.73326928319,1.00000000000001));
#26651=CARTESIAN_POINT('Ctrl Pts',(89.3127772822415,-24.7598575178004,1.));
#26652=CARTESIAN_POINT('Ctrl Pts',(89.3177733858486,-24.7863596889658,1.));
#26653=CARTESIAN_POINT('Ctrl Pts',(89.3347382842714,-24.8763511457426,1.));
#26654=CARTESIAN_POINT('Ctrl Pts',(89.3565634809553,-24.9653501497165,1.));
#26655=CARTESIAN_POINT('Ctrl Pts',(89.3829463368407,-25.053124461385,1.));
#26656=CARTESIAN_POINT('Ctrl Pts',(89.4099256760068,-25.1428832401492,1.));
#26657=CARTESIAN_POINT('Ctrl Pts',(89.4416712994606,-25.2313620234223,1.));
#26658=CARTESIAN_POINT('Ctrl Pts',(89.477913814938,-25.318308752927,1.));
#26659=CARTESIAN_POINT('Ctrl Pts',(89.4905805865942,-25.348696664869,1.));
#26660=CARTESIAN_POINT('Ctrl Pts',(89.5037971164698,-25.3788973526874,1.));
#26661=CARTESIAN_POINT('Ctrl Pts',(89.5175533368002,-25.4088996997776,1.));
#26662=CARTESIAN_POINT('Ctrl Pts',(89.5245000449555,-25.4240504856912,1.));
#26663=CARTESIAN_POINT('Ctrl Pts',(89.5315843916574,-25.4391506886467,1.));
#26664=CARTESIAN_POINT('Ctrl Pts',(89.5388051477195,-25.4541988513475,1.));
#26665=CARTESIAN_POINT('Ctrl Pts',(89.5448146544974,-25.46672275258,1.));
#26666=CARTESIAN_POINT('Ctrl Pts',(89.5509168026676,-25.4792066766568,1.));
#26667=CARTESIAN_POINT('Ctrl Pts',(89.5571069929132,-25.4916425965977,1.));
#26668=CARTESIAN_POINT('Ctrl Pts',(89.6000701103193,-25.5779543038758,1.));
#26669=CARTESIAN_POINT('Ctrl Pts',(89.6473202761524,-25.6620593555128,1.));
#26670=CARTESIAN_POINT('Ctrl Pts',(89.6985154201672,-25.7437076710158,1.));
#26671=CARTESIAN_POINT('Ctrl Pts',(89.7507153893452,-25.8269585268285,1.));
#26672=CARTESIAN_POINT('Ctrl Pts',(89.8070170326452,-25.9076560356431,1.));
#26673=CARTESIAN_POINT('Ctrl Pts',(89.8671126570608,-25.9855277789599,1.));
#26674=CARTESIAN_POINT('Ctrl Pts',(89.927676334208,-26.0640060237073,1.));
#26675=CARTESIAN_POINT('Ctrl Pts',(89.9920937838692,-26.1396151519006,1.));
#26676=CARTESIAN_POINT('Ctrl Pts',(90.0600992171408,-26.2120567437867,1.));
#26677=CARTESIAN_POINT('Ctrl Pts',(90.0970259686533,-26.2513923164617,1.));
#26678=CARTESIAN_POINT('Ctrl Pts',(90.1350114303598,-26.2897935420312,1.));
#26679=CARTESIAN_POINT('Ctrl Pts',(90.1740182898104,-26.3272088864004,1.));
#26680=CARTESIAN_POINT('Ctrl Pts',(90.1861457891855,-26.3388415728522,1.));
#26681=CARTESIAN_POINT('Ctrl Pts',(90.1983720446101,-26.3503789382668,1.));
#26682=CARTESIAN_POINT('Ctrl Pts',(90.2106959994552,-26.3618193692872,1.));
#26683=CARTESIAN_POINT('Ctrl Pts',(90.2219869755512,-26.3723008774397,1.));
#26684=CARTESIAN_POINT('Ctrl Pts',(90.2333542353844,-26.3826956655534,1.));
#26685=CARTESIAN_POINT('Ctrl Pts',(90.2447923276116,-26.3929988640505,1.));
#26686=CARTESIAN_POINT('Ctrl Pts',(90.3206014106021,-26.4612861286066,1.));
#26687=CARTESIAN_POINT('Ctrl Pts',(90.3995767828363,-26.5256063737863,0.999999999999999));
#26688=CARTESIAN_POINT('Ctrl Pts',(90.4813922770108,-26.5856769718563,0.999999999999999));
#26689=CARTESIAN_POINT('Ctrl Pts',(90.5632787218729,-26.6457996633627,1.));
#26690=CARTESIAN_POINT('Ctrl Pts',(90.6480107936052,-26.701666171117,1.));
#26691=CARTESIAN_POINT('Ctrl Pts',(90.7353064390064,-26.7529669283143,1.));
#26692=CARTESIAN_POINT('Ctrl Pts',(90.8208383089426,-26.803231173135,1.));
#26693=CARTESIAN_POINT('Ctrl Pts',(90.9088318713758,-26.8491129760809,1.));
#26694=CARTESIAN_POINT('Ctrl Pts',(90.9990555762685,-26.8902850239778,1.));
#26695=CARTESIAN_POINT('Ctrl Pts',(91.0368458850231,-26.9075299864179,1.));
#26696=CARTESIAN_POINT('Ctrl Pts',(91.0750277978247,-26.9239481874698,1.));
#26697=CARTESIAN_POINT('Ctrl Pts',(91.1135856932338,-26.9395132002532,1.));
#26698=CARTESIAN_POINT('Ctrl Pts',(91.1435994051254,-26.9516291055512,1.));
#26699=CARTESIAN_POINT('Ctrl Pts',(91.1738409492154,-26.9632280171349,1.));
#26700=CARTESIAN_POINT('Ctrl Pts',(91.2042985533737,-26.9743125149969,1.));
#26701=CARTESIAN_POINT('Ctrl Pts',(92.7937992825329,-26.9692229537457,1.));
#26702=CARTESIAN_POINT('Ctrl Pts',(92.8886355742527,-26.9345314146036,1.));
#26703=CARTESIAN_POINT('Ctrl Pts',(92.9814286349373,-26.8948494551323,0.999999999999998));
#26704=CARTESIAN_POINT('Ctrl Pts',(93.0719375317565,-26.8504973230386,0.999999999999999));
#26705=CARTESIAN_POINT('Ctrl Pts',(93.1637179471412,-26.8055221078961,1.));
#26706=CARTESIAN_POINT('Ctrl Pts',(93.253150237892,-26.7557438784191,1.));
#26707=CARTESIAN_POINT('Ctrl Pts',(93.3399491478414,-26.701455889429,1.));
#26708=CARTESIAN_POINT('Ctrl Pts',(93.3644578975098,-26.6861270018551,1.));
#26709=CARTESIAN_POINT('Ctrl Pts',(93.38875645171,-26.6704383481465,0.999999999999999));
#26710=CARTESIAN_POINT('Ctrl Pts',(93.4128377927018,-26.6543960746865,0.999999999999999));
#26711=CARTESIAN_POINT('Ctrl Pts',(93.4321685183665,-26.6415185199275,0.999999999999999));
#26712=CARTESIAN_POINT('Ctrl Pts',(93.4513613836409,-26.62841147677,1.));
#26713=CARTESIAN_POINT('Ctrl Pts',(93.4703934697505,-26.6150918905377,1.));
#26714=CARTESIAN_POINT('Ctrl Pts',(93.5531011008219,-26.5572090385068,0.999999999999999));
#26715=CARTESIAN_POINT('Ctrl Pts',(93.6328538966534,-26.4952643978376,0.999999999999999));
#26716=CARTESIAN_POINT('Ctrl Pts',(93.7093855017744,-26.4295552066869,1.));
#26717=CARTESIAN_POINT('Ctrl Pts',(93.7683983463317,-26.3788874299269,1.));
#26718=CARTESIAN_POINT('Ctrl Pts',(93.8254952956778,-26.3259804095853,1.));
#26719=CARTESIAN_POINT('Ctrl Pts',(93.8805366455773,-26.2709586400739,1.));
#26720=CARTESIAN_POINT('Ctrl Pts',(93.9098567587088,-26.2416489572678,1.));
#26721=CARTESIAN_POINT('Ctrl Pts',(93.9385932953215,-26.2117390413757,1.));
#26722=CARTESIAN_POINT('Ctrl Pts',(93.9667231085696,-26.1812468762253,1.));
#26723=CARTESIAN_POINT('Ctrl Pts',(93.976357091693,-26.1708038277108,1.));
#26724=CARTESIAN_POINT('Ctrl Pts',(93.9859191102224,-26.1602932647167,0.999999999999999));
#26725=CARTESIAN_POINT('Ctrl Pts',(93.9954016773941,-26.1497234378417,0.999999999999999));
#26726=CARTESIAN_POINT('Ctrl Pts',(94.0611941644384,-26.0763872636661,0.999999999999999));
#26727=CARTESIAN_POINT('Ctrl Pts',(94.1232544016247,-26.0001047407494,1.));
#26728=CARTESIAN_POINT('Ctrl Pts',(94.1813385979309,-25.9211542884475,1.));
#26729=CARTESIAN_POINT('Ctrl Pts',(94.2389163888163,-25.8428921634285,1.));
#26730=CARTESIAN_POINT('Ctrl Pts',(94.2925876036441,-25.7620076427722,1.));
#26731=CARTESIAN_POINT('Ctrl Pts',(94.3420689680264,-25.6787495218591,1.));
#26732=CARTESIAN_POINT('Ctrl Pts',(94.3901173496858,-25.5979025601834,0.999999999999999));
#26733=CARTESIAN_POINT('Ctrl Pts',(94.4342152487962,-25.5148167869307,1.));
#26734=CARTESIAN_POINT('Ctrl Pts',(94.4740555016775,-25.4297096831016,1.));
#26735=CARTESIAN_POINT('Ctrl Pts',(94.4948667673004,-25.3852524717113,1.));
#26736=CARTESIAN_POINT('Ctrl Pts',(94.5145154383506,-25.3402435941338,1.));
#26737=CARTESIAN_POINT('Ctrl Pts',(94.5329520278252,-25.2947138138489,1.));
#26738=CARTESIAN_POINT('Ctrl Pts',(94.5400926945258,-25.2770796963019,1.));
#26739=CARTESIAN_POINT('Ctrl Pts',(94.5470514948584,-25.2593674400535,1.));
#26740=CARTESIAN_POINT('Ctrl Pts',(94.5538253850611,-25.2415788415781,1.));
#26741=CARTESIAN_POINT('Ctrl Pts',(94.5589792730445,-25.2280444556963,1.));
#26742=CARTESIAN_POINT('Ctrl Pts',(94.5640260783963,-25.2144657562887,0.999999999999999));
#26743=CARTESIAN_POINT('Ctrl Pts',(94.5689596301442,-25.2008574386567,0.999999999999999));
#26744=CARTESIAN_POINT('Ctrl Pts',(94.6006314836872,-25.1134963112103,0.999999999999999));
#26745=CARTESIAN_POINT('Ctrl Pts',(94.6276946264954,-25.0247742561595,0.999999999999998));
#26746=CARTESIAN_POINT('Ctrl Pts',(94.6498977731061,-24.9349146809329,0.999999999999998));
#26747=CARTESIAN_POINT('Ctrl Pts',(94.6549003686514,-24.914668401493,0.999999999999998));
#26748=CARTESIAN_POINT('Ctrl Pts',(94.6596560431607,-24.894364336279,1.));
#26749=CARTESIAN_POINT('Ctrl Pts',(94.6641615567933,-24.8740049843512,1.));
#26750=CARTESIAN_POINT('Ctrl Pts',(94.684507085955,-24.7820683435733,1.));
#26751=CARTESIAN_POINT('Ctrl Pts',(94.6997556148072,-24.6890040031268,1.));
#26752=CARTESIAN_POINT('Ctrl Pts',(94.7100170529218,-24.5952037047372,1.));
#26753=CARTESIAN_POINT('Ctrl Pts',(94.7207301965731,-24.4972743443535,1.));
#26754=CARTESIAN_POINT('Ctrl Pts',(94.7260075138323,-24.3985415672063,0.999999999999998));
#26755=CARTESIAN_POINT('Ctrl Pts',(94.7259165861328,-24.299465853035,0.999999999999998));
#26756=CARTESIAN_POINT('Ctrl Pts',(94.7258814692624,-24.2612021661271,0.999999999999998));
#26757=CARTESIAN_POINT('Ctrl Pts',(94.7250450624305,-24.2228875809902,0.999999999999998));
#26758=CARTESIAN_POINT('Ctrl Pts',(94.7234091242725,-24.1845498020178,0.999999999999997));
#26759=CARTESIAN_POINT('Ctrl Pts',(94.7228215216315,-24.1707794892095,0.999999999999997));
#26760=CARTESIAN_POINT('Ctrl Pts',(94.7221307767868,-24.1570079821605,1.));
#26761=CARTESIAN_POINT('Ctrl Pts',(94.7213378612436,-24.1432482331353,1.));
#26762=CARTESIAN_POINT('Ctrl Pts',(94.7159862604884,-24.0503799776195,1.));
#26763=CARTESIAN_POINT('Ctrl Pts',(94.7059789500127,-23.9578988174462,0.999999999999996));
#26764=CARTESIAN_POINT('Ctrl Pts',(94.6914389868646,-23.8661766503703,0.999999999999997));
#26765=CARTESIAN_POINT('Ctrl Pts',(94.6769360712931,-23.7746881898014,0.999999999999998));
#26766=CARTESIAN_POINT('Ctrl Pts',(94.6579231604244,-23.6839539151715,1.));
#26767=CARTESIAN_POINT('Ctrl Pts',(94.6344737838795,-23.5943600003469,1.));
#26768=CARTESIAN_POINT('Ctrl Pts',(94.6114257043808,-23.5062993362386,0.999999999999998));
#26769=CARTESIAN_POINT('Ctrl Pts',(94.5840912373833,-23.4193395518976,1.));
#26770=CARTESIAN_POINT('Ctrl Pts',(94.5524998666925,-23.3338765545241,1.));
#26771=CARTESIAN_POINT('Ctrl Pts',(94.5366373923581,-23.2909643739907,1.));
#26772=CARTESIAN_POINT('Ctrl Pts',(94.5197010774786,-23.2484300968532,1.));
#26773=CARTESIAN_POINT('Ctrl Pts',(94.5016912657434,-23.206327621631,1.));
#26774=CARTESIAN_POINT('Ctrl Pts',(94.4963919504663,-23.1939391362082,1.));
#26775=CARTESIAN_POINT('Ctrl Pts',(94.4909996770287,-23.1815880553872,1.));
#26776=CARTESIAN_POINT('Ctrl Pts',(94.485514419704,-23.1692758010802,1.));
#26777=CARTESIAN_POINT('Ctrl Pts',(94.4799210007597,-23.1567207663004,1.));
#26778=CARTESIAN_POINT('Ctrl Pts',(94.4742345748605,-23.1442143929032,1.));
#26779=CARTESIAN_POINT('Ctrl Pts',(94.4684564310145,-23.1317600158838,1.));
#26780=CARTESIAN_POINT('Ctrl Pts',(94.4309710580974,-23.0509629676511,1.));
#26781=CARTESIAN_POINT('Ctrl Pts',(94.3896159815805,-22.9723227780457,1.));
#26782=CARTESIAN_POINT('Ctrl Pts',(94.3444610246362,-22.8961871515012,0.999999999999999));
#26783=CARTESIAN_POINT('Ctrl Pts',(94.3000642491435,-22.8213298922449,0.999999999999999));
#26784=CARTESIAN_POINT('Ctrl Pts',(94.2519936725177,-22.7488931261332,1.));
#26785=CARTESIAN_POINT('Ctrl Pts',(94.2002794589025,-22.6792415177607,1.));
#26786=CARTESIAN_POINT('Ctrl Pts',(94.1501451854236,-22.61171786153,1.));
#26787=CARTESIAN_POINT('Ctrl Pts',(94.0965860671228,-22.5468113410791,0.999999999999999));
#26788=CARTESIAN_POINT('Ctrl Pts',(94.0396018953678,-22.4848944920469,0.999999999999999));
#26789=CARTESIAN_POINT('Ctrl Pts',(94.0184128484534,-22.4618712738701,0.999999999999999));
#26790=CARTESIAN_POINT('Ctrl Pts',(93.9967499855334,-22.439261866594,0.999999999999998));
#26791=CARTESIAN_POINT('Ctrl Pts',(93.9746124571306,-22.4170870902725,0.999999999999998));
#26792=CARTESIAN_POINT('Ctrl Pts',(93.9557856680546,-22.3982286238251,0.999999999999998));
#26793=CARTESIAN_POINT('Ctrl Pts',(93.9366155517544,-22.3796845329471,0.999999999999999));
#26794=CARTESIAN_POINT('Ctrl Pts',(93.9171118396844,-22.3614597340103,0.999999999999999));
#26795=CARTESIAN_POINT('Origin',(92.,-24.,12.2084234471775));
#26796=CARTESIAN_POINT('Ctrl Pts',(88.9232328435277,-23.9980626432726,9.70842344717746));
#26797=CARTESIAN_POINT('Ctrl Pts',(88.9222986726779,-23.8738980500463,9.70197366100994));
#26798=CARTESIAN_POINT('Ctrl Pts',(88.9853330132547,-22.7368858898031,9.64286281975954));
#26799=CARTESIAN_POINT('Ctrl Pts',(90.4009680446667,-20.744487174453,9.53109092342626));
#26800=CARTESIAN_POINT('Ctrl Pts',(93.8523951731074,-20.8820464105141,9.37310775817762));
#26801=CARTESIAN_POINT('Ctrl Pts',(95.6235721938174,-23.847285073477,9.215124592929));
#26802=CARTESIAN_POINT('Ctrl Pts',(94.1080771138749,-26.9512425629647,9.05714142768035));
#26803=CARTESIAN_POINT('Ctrl Pts',(90.680468686986,-27.3782238204297,8.89915826243172));
#26804=CARTESIAN_POINT('Ctrl Pts',(89.0391556852518,-25.4378982357328,8.78291893559742));
#26805=CARTESIAN_POINT('Ctrl Pts',(88.9237203439564,-24.2133137839327,8.719340663846));
#26806=CARTESIAN_POINT('Ctrl Pts',(88.925632185667,-24.0026790855389,8.70842344717745));
#26807=CARTESIAN_POINT('Ctrl Pts',(88.9297109890477,-24.0031050978172,9.79157655282255));
#26808=CARTESIAN_POINT('Ctrl Pts',(88.9347146650535,-23.3096207752369,9.75572892504928));
#26809=CARTESIAN_POINT('Ctrl Pts',(89.5077566649198,-21.5876413967006,9.66722024219312));
#26810=CARTESIAN_POINT('Ctrl Pts',(92.3539160472627,-20.3911616367203,9.52605050425409));
#26811=CARTESIAN_POINT('Ctrl Pts',(95.215603926767,-22.3229247027849,9.36806733900546));
#26812=CARTESIAN_POINT('Ctrl Pts',(95.1618223030446,-25.7771165220753,9.21008417375683));
#26813=CARTESIAN_POINT('Ctrl Pts',(92.2395757220273,-27.6187839878381,9.0521010085082));
#26814=CARTESIAN_POINT('Ctrl Pts',(89.4675381047452,-26.3468885879089,8.91259846819676));
#26815=CARTESIAN_POINT('Ctrl Pts',(88.9339207778366,-24.6595175431003,8.82575698296822));
#26816=CARTESIAN_POINT('Ctrl Pts',(88.9296146841086,-23.99786424691,8.79157655282255));
#26817=CARTESIAN_POINT('Ctrl Pts',(93.9134659966651,-22.3640127966251,10.));
#26818=CARTESIAN_POINT('Ctrl Pts',(94.4547800806522,-22.9971388327508,9.94733894491712));
#26819=CARTESIAN_POINT('Ctrl Pts',(94.8501256748086,-24.8326016501471,9.84201683475137));
#26820=CARTESIAN_POINT('Ctrl Pts',(92.8579877031057,-26.8458064948082,9.68403366950272));
#26821=CARTESIAN_POINT('Ctrl Pts',(90.0866997272543,-26.2718360144009,9.5260505042541));
#26822=CARTESIAN_POINT('Ctrl Pts',(89.0512847401284,-23.6401113487857,9.36806733900546));
#26823=CARTESIAN_POINT('Ctrl Pts',(90.6902349284037,-21.3334135225917,9.21008417375683));
#26824=CARTESIAN_POINT('Ctrl Pts',(93.5172945659013,-21.4460881205366,9.05210100850819));
#26825=CARTESIAN_POINT('Ctrl Pts',(94.9680634449115,-23.8749113949824,8.89411784325956));
#26826=CARTESIAN_POINT('Ctrl Pts',(93.7267233233056,-26.4173590864694,8.73613467801093));
#26827=CARTESIAN_POINT('Ctrl Pts',(90.9191735544127,-26.7670988996036,8.57815151276228));
#26828=CARTESIAN_POINT('Ctrl Pts',(89.0919764590838,-24.6070250632274,8.42016834751366));
#26829=CARTESIAN_POINT('Ctrl Pts',(89.9024529386512,-21.8963394365791,8.26218518226502));
#26830=CARTESIAN_POINT('Ctrl Pts',(92.6154776819786,-21.0937552116683,8.10420201701638));
#26831=CARTESIAN_POINT('Ctrl Pts',(94.7702424329595,-22.9272295704909,7.94621885176776));
#26832=CARTESIAN_POINT('Ctrl Pts',(94.4123030989785,-25.7337455944376,7.78823568651911));
#26833=CARTESIAN_POINT('Ctrl Pts',(91.8663223428291,-26.9676940765812,7.63025252127049));
#26834=CARTESIAN_POINT('Ctrl Pts',(89.441591869785,-25.509843281544,7.47226935602184));
#26835=CARTESIAN_POINT('Ctrl Pts',(89.3374248530143,-22.6825128295981,7.31428619077321));
#26836=CARTESIAN_POINT('Ctrl Pts',(91.648304394415,-21.0501883402777,7.15630302552458));
#26837=CARTESIAN_POINT('Ctrl Pts',(94.2781838441901,-22.0934436458725,6.99831986027595));
#26838=CARTESIAN_POINT('Ctrl Pts',(94.8416727928904,-24.8660106707762,6.84033669502731));
#26839=CARTESIAN_POINT('Ctrl Pts',(92.8276675236541,-26.8530764431805,6.68235352977868));
#26840=CARTESIAN_POINT('Ctrl Pts',(90.0629395615723,-26.2523045074983,6.52437036453004));
#26841=CARTESIAN_POINT('Ctrl Pts',(89.055191532594,-23.6086155038654,6.36638719928141));
#26842=CARTESIAN_POINT('Ctrl Pts',(90.7184852964603,-21.3199255988147,6.20840403403277));
#26843=CARTESIAN_POINT('Ctrl Pts',(93.5441566371434,-21.4621546514439,6.05042086878414));
#26844=CARTESIAN_POINT('Ctrl Pts',(94.9692252026282,-23.9062960577466,5.89243770353551));
#26845=CARTESIAN_POINT('Ctrl Pts',(93.7011051632761,-26.4354301377776,5.73445453828687));
#26846=CARTESIAN_POINT('Ctrl Pts',(90.8900246784809,-26.7555459564984,5.57647137303824));
#26847=CARTESIAN_POINT('Ctrl Pts',(89.0857296961368,-24.5762875399298,5.4184882077896));
#26848=CARTESIAN_POINT('Ctrl Pts',(89.9247773496848,-21.8743166547494,5.26050504254097));
#26849=CARTESIAN_POINT('Ctrl Pts',(92.6461227788815,-21.1004131178103,5.10252187729233));
#26850=CARTESIAN_POINT('Ctrl Pts',(94.781412794043,-22.9565338521763,4.9445387120437));
#26851=CARTESIAN_POINT('Ctrl Pts',(94.3938664694978,-25.7591139982761,4.78655554679506));
#26852=CARTESIAN_POINT('Ctrl Pts',(91.8350015491773,-26.9661177057641,4.62857238154643));
#26853=CARTESIAN_POINT('Ctrl Pts',(89.4257958558034,-25.4827514138513,4.4705892162978));
#26854=CARTESIAN_POINT('Ctrl Pts',(89.3514811837096,-22.6544789807379,4.31260605104916));
#26855=CARTESIAN_POINT('Ctrl Pts',(91.6794634788654,-21.0466400362912,4.15462288580053));
#26856=CARTESIAN_POINT('Ctrl Pts',(94.2981833367367,-22.1175993861324,3.99663972055189));
#26857=CARTESIAN_POINT('Ctrl Pts',(94.832372471477,-24.8959603376103,3.83865655530326));
#26858=CARTESIAN_POINT('Ctrl Pts',(92.7975030889959,-26.8616546930814,3.68067339005462));
#26859=CARTESIAN_POINT('Ctrl Pts',(90.0392712060535,-26.2317305445351,3.52269022480599));
#26860=CARTESIAN_POINT('Ctrl Pts',(89.059487218677,-23.5775506652917,3.36470705955735));
#26861=CARTESIAN_POINT('Ctrl Pts',(90.7468487806939,-21.3065466558477,3.20672389430872));
#26862=CARTESIAN_POINT('Ctrl Pts',(93.570861086046,-21.4785969587254,3.04874072906008));
#26863=CARTESIAN_POINT('Ctrl Pts',(94.9700491479981,-23.9376454809303,2.89075756381145));
#26864=CARTESIAN_POINT('Ctrl Pts',(93.6753004854887,-26.4532524972207,2.73277439856281));
#26865=CARTESIAN_POINT('Ctrl Pts',(90.86099868006,-26.7436740950583,2.57479123331418));
#26866=CARTESIAN_POINT('Ctrl Pts',(89.0798067232475,-24.545493049519,2.41680806806554));
#26867=CARTESIAN_POINT('Ctrl Pts',(89.9473363281977,-21.8525242277567,2.25882490281691));
#26868=CARTESIAN_POINT('Ctrl Pts',(92.6766884907985,-21.1074034480955,2.10084173756828));
#26869=CARTESIAN_POINT('Ctrl Pts',(94.7922885760843,-22.9859374299123,1.94285857231964));
#26870=CARTESIAN_POINT('Ctrl Pts',(94.3751314870431,-25.7843200921868,1.78487540707101));
#26871=CARTESIAN_POINT('Ctrl Pts',(91.8037637139842,-26.96414237307,1.62689224182237));
#26872=CARTESIAN_POINT('Ctrl Pts',(89.4101547923377,-25.4556338085585,1.46890907657374));
#26873=CARTESIAN_POINT('Ctrl Pts',(89.3661021422764,-22.6263102241946,1.3109259113251));
#26874=CARTESIAN_POINT('Ctrl Pts',(91.7101077338689,-21.0440028274616,1.15294274607647));
#26875=CARTESIAN_POINT('Ctrl Pts',(94.3190522551594,-22.14076517287,0.994959580827836));
#26876=CARTESIAN_POINT('Ctrl Pts',(94.8204142519502,-24.9282808397392,0.836976415579201));
#26877=CARTESIAN_POINT('Ctrl Pts',(93.4549268544596,-26.2169491679593,0.731654305413445));
#26878=CARTESIAN_POINT('Ctrl Pts',(92.6501999979751,-26.4320868020351,0.678993250330566));
#26879=CARTESIAN_POINT('Ctrl Pts',(94.0543315503421,-22.2435746787732,10.1070022498898));
#26880=CARTESIAN_POINT('Ctrl Pts',(94.6354960985062,-22.9233101920371,10.0543411948069));
#26881=CARTESIAN_POINT('Ctrl Pts',(95.0599462474923,-24.8938961244909,9.94901908464118));
#26882=CARTESIAN_POINT('Ctrl Pts',(92.9211510480811,-27.0553090980672,9.79103591939255));
#26883=CARTESIAN_POINT('Ctrl Pts',(89.9458463738419,-26.4390840546533,9.6330527541439));
#26884=CARTESIAN_POINT('Ctrl Pts',(88.8342061986536,-23.6136170634398,9.47506958889528));
#26885=CARTESIAN_POINT('Ctrl Pts',(90.5938126338247,-21.1371047398788,9.31708642364664));
#26886=CARTESIAN_POINT('Ctrl Pts',(93.6289947683033,-21.2580742171958,9.159103258398));
#26887=CARTESIAN_POINT('Ctrl Pts',(95.1865663612134,-23.8657026211472,9.00112009314937));
#26888=CARTESIAN_POINT('Ctrl Pts',(93.8538412534954,-26.5953202453012,8.84313692790073));
#26889=CARTESIAN_POINT('Ctrl Pts',(90.8396052652705,-26.9708072065457,8.6851537626521));
#26890=CARTESIAN_POINT('Ctrl Pts',(88.8778935608714,-24.6517130387526,8.52717059740347));
#26891=CARTESIAN_POINT('Ctrl Pts',(89.7480357038138,-21.7414721379016,8.36918743215483));
#26892=CARTESIAN_POINT('Ctrl Pts',(92.6607879224527,-20.8798032616766,8.21120426690619));
#26893=CARTESIAN_POINT('Ctrl Pts',(94.9741821605629,-22.848254349199,8.05322110165757));
#26894=CARTESIAN_POINT('Ctrl Pts',(94.5898920460865,-25.8613804902347,7.89523793640892));
#26895=CARTESIAN_POINT('Ctrl Pts',(91.85648126009,-27.1861698007228,7.7372547711603));
#26896=CARTESIAN_POINT('Ctrl Pts',(89.2532469614236,-25.6209949352399,7.57927160591165));
#26897=CARTESIAN_POINT('Ctrl Pts',(89.1414113764536,-22.5855220494931,7.42128844066304));
#26898=CARTESIAN_POINT('Ctrl Pts',(91.6224132647619,-20.8330290840307,7.26330527541438));
#26899=CARTESIAN_POINT('Ctrl Pts',(94.4458991990223,-21.9530867663101,7.10532211016576));
#26900=CARTESIAN_POINT('Ctrl Pts',(95.0508710812514,-24.929764650644,6.94733894491712));
#26901=CARTESIAN_POINT('Ctrl Pts',(92.8885987574378,-27.0631142455517,6.78935577966849));
#26902=CARTESIAN_POINT('Ctrl Pts',(89.9203370321098,-26.4181146771334,6.63137261441986));
#26903=CARTESIAN_POINT('Ctrl Pts',(88.8384006013953,-23.5798025571787,6.47338944917122));
#26904=CARTESIAN_POINT('Ctrl Pts',(90.6241427376827,-21.122623862031,6.31540628392259));
#26905=CARTESIAN_POINT('Ctrl Pts',(93.6578343717016,-21.2753235340925,6.15742311867394));
#26906=CARTESIAN_POINT('Ctrl Pts',(95.1878136452183,-23.8993977602433,5.99943995342532));
#26907=CARTESIAN_POINT('Ctrl Pts',(93.8263371355742,-26.6147216513962,5.84145678817668));
#26908=CARTESIAN_POINT('Ctrl Pts',(90.8083105071782,-26.9584037587908,5.68347362292805));
#26909=CARTESIAN_POINT('Ctrl Pts',(88.8711869236842,-24.6187126802411,5.52549045767941));
#26910=CARTESIAN_POINT('Ctrl Pts',(89.7720035935014,-21.7178280827588,5.36750729243077));
#26911=CARTESIAN_POINT('Ctrl Pts',(92.6936890503225,-20.8869513096014,5.20952412718214));
#26912=CARTESIAN_POINT('Ctrl Pts',(94.9861748613701,-22.8797159537069,5.05154096193351));
#26913=CARTESIAN_POINT('Ctrl Pts',(94.5700981486823,-25.8886164654117,4.89355779668487));
#26914=CARTESIAN_POINT('Ctrl Pts',(91.8228546920231,-27.1844773806274,4.73557463143624));
#26915=CARTESIAN_POINT('Ctrl Pts',(89.2362880763697,-25.5919086182341,4.5775914661876));
#26916=CARTESIAN_POINT('Ctrl Pts',(89.1565025062044,-22.5554244045433,4.41960830093897));
#26917=CARTESIAN_POINT('Ctrl Pts',(91.6558662189183,-20.8292195609755,4.26162513569033));
#26918=CARTESIAN_POINT('Ctrl Pts',(94.4673710143567,-21.9790208040324,4.1036419704417));
#26919=CARTESIAN_POINT('Ctrl Pts',(95.0408860887087,-24.9619191522692,3.94565880519306));
#26920=CARTESIAN_POINT('Ctrl Pts',(92.8562136772091,-27.0723240091163,3.78767563994443));
#26921=CARTESIAN_POINT('Ctrl Pts',(89.8949262594222,-26.3960261000149,3.6296924746958));
#26922=CARTESIAN_POINT('Ctrl Pts',(88.8430125273276,-23.5464507870927,3.47170930944716));
#26923=CARTESIAN_POINT('Ctrl Pts',(90.6545942851052,-21.1082599879431,3.31372614419853));
#26924=CARTESIAN_POINT('Ctrl Pts',(93.6865047489179,-21.2929762912711,3.1557429789499));
#26925=CARTESIAN_POINT('Ctrl Pts',(95.1886982478045,-23.9330550654913,2.99775981370126));
#26926=CARTESIAN_POINT('Ctrl Pts',(93.7986327688294,-26.6338560574266,2.83977664845263));
#26927=CARTESIAN_POINT('Ctrl Pts',(90.7771476725941,-26.9456579145687,2.68179348320399));
#26928=CARTESIAN_POINT('Ctrl Pts',(88.8648279133335,-24.585651160811,2.52381031795536));
#26929=CARTESIAN_POINT('Ctrl Pts',(89.7962233190588,-21.694431340717,2.36582715270672));
#26930=CARTESIAN_POINT('Ctrl Pts',(92.7265049490419,-20.8944562540725,2.20784398745809));
#26931=CARTESIAN_POINT('Ctrl Pts',(94.9978512968129,-22.9112841642428,2.04986082220945));
#26932=CARTESIAN_POINT('Ctrl Pts',(94.5499839341528,-25.9156781817275,1.89187765696082));
#26933=CARTESIAN_POINT('Ctrl Pts',(91.7893171896512,-27.1823566278765,1.73389449171218));
#26934=CARTESIAN_POINT('Ctrl Pts',(89.2194955489798,-25.5627946688775,1.57591132646355));
#26935=CARTESIAN_POINT('Ctrl Pts',(89.1721998306056,-22.5251819202756,1.41792816121491));
#26936=CARTESIAN_POINT('Ctrl Pts',(91.6887664429098,-20.8263882060871,1.25994499596628));
#26937=CARTESIAN_POINT('Ctrl Pts',(94.4897762609678,-22.0038920098267,1.10196183071765));
#26938=CARTESIAN_POINT('Ctrl Pts',(95.0280475288895,-24.9966190253592,0.943978665469011));
#26939=CARTESIAN_POINT('Ctrl Pts',(93.5620356702265,-26.3801565479508,0.838656555303256));
#26940=CARTESIAN_POINT('Ctrl Pts',(92.698066426161,-26.6111321859386,0.785995500220377));
#26941=CARTESIAN_POINT('Ctrl Pts',(94.1951971040191,-22.1231365609213,10.2140044997796));
#26942=CARTESIAN_POINT('Ctrl Pts',(94.8162121163602,-22.8494815513233,10.1613434446967));
#26943=CARTESIAN_POINT('Ctrl Pts',(95.269766820176,-24.9551905988348,10.056021334531));
#26944=CARTESIAN_POINT('Ctrl Pts',(92.9843143930565,-27.2648117013262,9.89803816928236));
#26945=CARTESIAN_POINT('Ctrl Pts',(89.8049930204297,-26.6063320949058,9.74005500403372));
#26946=CARTESIAN_POINT('Ctrl Pts',(88.6171276571787,-23.5871227780939,9.58207183878508));
#26947=CARTESIAN_POINT('Ctrl Pts',(90.4973903392457,-20.9407959571659,9.42408867353645));
#26948=CARTESIAN_POINT('Ctrl Pts',(93.7406949707054,-21.070060313855,9.26610550828781));
#26949=CARTESIAN_POINT('Ctrl Pts',(95.4050692775153,-23.8564938473121,9.10812234303918));
#26950=CARTESIAN_POINT('Ctrl Pts',(93.9809591836852,-26.7732814041329,8.95013917779054));
#26951=CARTESIAN_POINT('Ctrl Pts',(90.7600369761282,-27.1745155134877,8.79215601254191));
#26952=CARTESIAN_POINT('Ctrl Pts',(88.663810662659,-24.6964010142779,8.63417284729327));
#26953=CARTESIAN_POINT('Ctrl Pts',(89.5936184689763,-21.5866048392241,8.47618968204464));
#26954=CARTESIAN_POINT('Ctrl Pts',(92.7060981629268,-20.6658513116849,8.31820651679601));
#26955=CARTESIAN_POINT('Ctrl Pts',(95.1781218881664,-22.7692791279071,8.16022335154737));
#26956=CARTESIAN_POINT('Ctrl Pts',(94.7674809931943,-25.9890153860317,8.00224018629874));
#26957=CARTESIAN_POINT('Ctrl Pts',(91.8466401773509,-27.4046455248644,7.84425702105011));
#26958=CARTESIAN_POINT('Ctrl Pts',(89.0649020530621,-25.7321465889358,7.68627385580147));
#26959=CARTESIAN_POINT('Ctrl Pts',(88.9453978998932,-22.488531269388,7.52829069055284));
#26960=CARTESIAN_POINT('Ctrl Pts',(91.5965221351087,-20.6158698277837,7.37030752530419));
#26961=CARTESIAN_POINT('Ctrl Pts',(94.6136145538545,-21.8127298867477,7.21232436005558));
#26962=CARTESIAN_POINT('Ctrl Pts',(95.2600693696124,-24.9935186305119,7.05434119480693));
#26963=CARTESIAN_POINT('Ctrl Pts',(92.9495299912217,-27.2731520479229,6.8963580295583));
#26964=CARTESIAN_POINT('Ctrl Pts',(89.7777345026471,-26.5839248467685,6.73837486430966));
#26965=CARTESIAN_POINT('Ctrl Pts',(88.6216096701968,-23.5509896104921,6.58039169906103));
#26966=CARTESIAN_POINT('Ctrl Pts',(90.529800178905,-20.9253221252473,6.42240853381239));
#26967=CARTESIAN_POINT('Ctrl Pts',(93.77151210626,-21.088492416741,6.26442536856375));
#26968=CARTESIAN_POINT('Ctrl Pts',(95.4064020878083,-23.8924994627401,6.10644220331513));
#26969=CARTESIAN_POINT('Ctrl Pts',(93.9515691078723,-26.7940131650148,5.94845903806649));
#26970=CARTESIAN_POINT('Ctrl Pts',(90.7265963358753,-27.1612615610831,5.79047587281786));
#26971=CARTESIAN_POINT('Ctrl Pts',(88.6566441512317,-24.6611378205524,5.63249270756922));
#26972=CARTESIAN_POINT('Ctrl Pts',(89.6192298373179,-21.5613395107681,5.47450954232059));
#26973=CARTESIAN_POINT('Ctrl Pts',(92.7412553217636,-20.6734895013926,5.31652637707195));
#26974=CARTESIAN_POINT('Ctrl Pts',(95.1909369286972,-22.8028980552375,5.15854321182332));
#26975=CARTESIAN_POINT('Ctrl Pts',(94.7463298278668,-26.0181189325473,5.00056004657468));
#26976=CARTESIAN_POINT('Ctrl Pts',(91.8107078348689,-27.4028370554907,4.84257688132605));
#26977=CARTESIAN_POINT('Ctrl Pts',(89.0467802969359,-25.7010658226169,4.68459371607741));
#26978=CARTESIAN_POINT('Ctrl Pts',(88.9615238286993,-22.4563698283487,4.52661055082878));
#26979=CARTESIAN_POINT('Ctrl Pts',(91.6322689589712,-20.6117990856598,4.36862738558015));
#26980=CARTESIAN_POINT('Ctrl Pts',(94.6365586919768,-21.8404422219323,4.21064422033151));
#26981=CARTESIAN_POINT('Ctrl Pts',(95.2493997059401,-25.0278779669281,4.05266105508288));
#26982=CARTESIAN_POINT('Ctrl Pts',(92.9149242654226,-27.2829933251512,3.89467788983424));
#26983=CARTESIAN_POINT('Ctrl Pts',(89.7505813127906,-26.5603216554947,3.73669472458561));
#26984=CARTESIAN_POINT('Ctrl Pts',(88.6265378359784,-23.5153509088937,3.57871155933697));
#26985=CARTESIAN_POINT('Ctrl Pts',(90.5623397895163,-20.9099733200387,3.42072839408834));
#26986=CARTESIAN_POINT('Ctrl Pts',(93.8021484117901,-21.1073556238168,3.2627452288397));
#26987=CARTESIAN_POINT('Ctrl Pts',(95.4073473476108,-23.9284646500523,3.10476206359107));
#26988=CARTESIAN_POINT('Ctrl Pts',(93.9219650521703,-26.8144596176325,2.94677889834244));
#26989=CARTESIAN_POINT('Ctrl Pts',(90.693296665128,-27.1476417340791,2.7887957330938));
#26990=CARTESIAN_POINT('Ctrl Pts',(88.6498491034197,-24.6258092721029,2.63081256784516));
#26991=CARTESIAN_POINT('Ctrl Pts',(89.6451103099197,-21.5363384536773,2.47282940259654));
#26992=CARTESIAN_POINT('Ctrl Pts',(92.7763214072855,-20.6815090600495,2.3148462373479));
#26993=CARTESIAN_POINT('Ctrl Pts',(95.2034140175415,-22.8366308985733,2.15686307209927));
#26994=CARTESIAN_POINT('Ctrl Pts',(94.7248363812625,-26.0470362712681,1.99887990685063));
#26995=CARTESIAN_POINT('Ctrl Pts',(91.7748706653183,-27.4005708826831,1.840896741602));
#26996=CARTESIAN_POINT('Ctrl Pts',(89.0288363056218,-25.6699555291964,1.68291357635336));
#26997=CARTESIAN_POINT('Ctrl Pts',(88.9782975189349,-22.4240536163567,1.52493041110473));
#26998=CARTESIAN_POINT('Ctrl Pts',(91.6674251519505,-20.6087735847125,1.36694724585609));
#26999=CARTESIAN_POINT('Ctrl Pts',(94.6605002667765,-21.8670188467834,1.20896408060746));
#27000=CARTESIAN_POINT('Ctrl Pts',(95.2356808058288,-25.0649572109792,1.05098091535882));
#27001=CARTESIAN_POINT('Ctrl Pts',(93.6691444859934,-26.5433639279422,0.945658805193066));
#27002=CARTESIAN_POINT('Ctrl Pts',(92.7459328543469,-26.7901775698422,0.892997750110188));
#27003=CARTESIAN_POINT('Ctrl Pts',(94.3360626576961,-22.0026984430694,10.3210067496694));
#27004=CARTESIAN_POINT('Ctrl Pts',(94.9969281342143,-22.7756529106096,10.2683456945866));
#27005=CARTESIAN_POINT('Ctrl Pts',(95.4795873928596,-25.0164850731786,10.1630235844208));
#27006=CARTESIAN_POINT('Ctrl Pts',(93.0474777380319,-27.4743143045852,10.0050404191722));
#27007=CARTESIAN_POINT('Ctrl Pts',(89.6641396670172,-26.7735801351583,9.84705725392352));
#27008=CARTESIAN_POINT('Ctrl Pts',(88.4000491157039,-23.5606284927479,9.6890740886749));
#27009=CARTESIAN_POINT('Ctrl Pts',(90.4009680446667,-20.744487174453,9.53109092342626));
#27010=CARTESIAN_POINT('Ctrl Pts',(93.8523951731074,-20.8820464105141,9.37310775817762));
#27011=CARTESIAN_POINT('Ctrl Pts',(95.6235721938174,-23.847285073477,9.215124592929));
#27012=CARTESIAN_POINT('Ctrl Pts',(94.1080771138749,-26.9512425629647,9.05714142768035));
#27013=CARTESIAN_POINT('Ctrl Pts',(90.680468686986,-27.3782238204297,8.89915826243172));
#27014=CARTESIAN_POINT('Ctrl Pts',(88.4497277644466,-24.7410889898031,8.74117509718309));
#27015=CARTESIAN_POINT('Ctrl Pts',(89.4392012341389,-21.4317375405466,8.58319193193445));
#27016=CARTESIAN_POINT('Ctrl Pts',(92.7514084034007,-20.4518993616932,8.42520876668581));
#27017=CARTESIAN_POINT('Ctrl Pts',(95.38206161577,-22.6903039066152,8.26722560143718));
#27018=CARTESIAN_POINT('Ctrl Pts',(94.9450699403021,-26.1166502818288,8.10924243618855));
#27019=CARTESIAN_POINT('Ctrl Pts',(91.8367990946118,-27.6231212490059,7.95125927093992));
#27020=CARTESIAN_POINT('Ctrl Pts',(88.8765571447008,-25.8432982426317,7.79327610569128));
#27021=CARTESIAN_POINT('Ctrl Pts',(88.7493844233324,-22.3915404892829,7.63529294044265));
#27022=CARTESIAN_POINT('Ctrl Pts',(91.5706310054557,-20.3987105715367,7.47730977519401));
#27023=CARTESIAN_POINT('Ctrl Pts',(94.7813299086865,-21.6723730071853,7.31932660994538));
#27024=CARTESIAN_POINT('Ctrl Pts',(95.4692676579736,-25.0572726103797,7.16134344469675));
#27025=CARTESIAN_POINT('Ctrl Pts',(93.0104612250053,-27.483189850294,7.00336027944811));
#27026=CARTESIAN_POINT('Ctrl Pts',(89.6351319731846,-26.7497350164036,6.84537711419948));
#27027=CARTESIAN_POINT('Ctrl Pts',(88.4048187389981,-23.5221766638054,6.68739394895084));
#27028=CARTESIAN_POINT('Ctrl Pts',(90.4354576201273,-20.7280203884636,6.52941078370221));
#27029=CARTESIAN_POINT('Ctrl Pts',(93.8851898408184,-20.9016612993894,6.37142761845357));
#27030=CARTESIAN_POINT('Ctrl Pts',(95.6249905303983,-23.885601165237,6.21344445320494));
#27031=CARTESIAN_POINT('Ctrl Pts',(94.0768010801705,-26.9733046786334,6.0554612879563));
#27032=CARTESIAN_POINT('Ctrl Pts',(90.6448821645723,-27.3641193633755,5.89747812270767));
#27033=CARTESIAN_POINT('Ctrl Pts',(88.4421013787792,-24.7035629608637,5.73949495745903));
#27034=CARTESIAN_POINT('Ctrl Pts',(89.4664560811345,-21.4048509387775,5.5815117922104));
#27035=CARTESIAN_POINT('Ctrl Pts',(92.7888215932045,-20.4600276931837,5.42352862696176));
#27036=CARTESIAN_POINT('Ctrl Pts',(95.3956989960243,-22.7260801567682,5.26554546171313));
#27037=CARTESIAN_POINT('Ctrl Pts',(94.9225615070513,-26.1476213996829,5.10756229646449));
#27038=CARTESIAN_POINT('Ctrl Pts',(91.7985609777146,-27.6211967303539,4.94957913121586));
#27039=CARTESIAN_POINT('Ctrl Pts',(88.8572725175023,-25.8102230269998,4.79159596596722));
#27040=CARTESIAN_POINT('Ctrl Pts',(88.7665451511941,-22.3573152521541,4.6336128007186));
#27041=CARTESIAN_POINT('Ctrl Pts',(91.6086716990242,-20.394378610344,4.47562963546995));
#27042=CARTESIAN_POINT('Ctrl Pts',(94.8057463695968,-21.7018636398323,4.31764647022133));
#27043=CARTESIAN_POINT('Ctrl Pts',(95.4579133231718,-25.0938367815869,4.15966330497269));
#27044=CARTESIAN_POINT('Ctrl Pts',(92.9736348536358,-27.493662641186,4.00168013972405));
#27045=CARTESIAN_POINT('Ctrl Pts',(89.6062363661592,-26.7246172109746,3.84369697447542));
#27046=CARTESIAN_POINT('Ctrl Pts',(88.4100631446291,-23.4842510306947,3.68571380922679));
#27047=CARTESIAN_POINT('Ctrl Pts',(90.4700852939275,-20.7116866521342,3.52773064397815));
#27048=CARTESIAN_POINT('Ctrl Pts',(93.9177920746623,-20.9217349563625,3.36974747872952));
#27049=CARTESIAN_POINT('Ctrl Pts',(95.625996447417,-23.9238742346134,3.21176431348088));
#27050=CARTESIAN_POINT('Ctrl Pts',(94.0452973355112,-26.9950631778383,3.05378114823225));
#27051=CARTESIAN_POINT('Ctrl Pts',(90.6094456576621,-27.3496255535896,2.89579798298361));
#27052=CARTESIAN_POINT('Ctrl Pts',(88.4348702935058,-24.6659673833949,2.73781481773498));
#27053=CARTESIAN_POINT('Ctrl Pts',(89.4939973007808,-21.3782455666376,2.57983165248634));
#27054=CARTESIAN_POINT('Ctrl Pts',(92.8261378655289,-20.4685618660265,2.42184848723771));
#27055=CARTESIAN_POINT('Ctrl Pts',(95.4089767382702,-22.7619776329039,2.26386532198907));
#27056=CARTESIAN_POINT('Ctrl Pts',(94.899688828372,-26.1783943608088,2.10588215674044));
#27057=CARTESIAN_POINT('Ctrl Pts',(91.7604241409854,-27.6187851374898,1.9478989914918));
#27058=CARTESIAN_POINT('Ctrl Pts',(88.8381770622638,-25.7771163895153,1.78991582624317));
#27059=CARTESIAN_POINT('Ctrl Pts',(88.784395207264,-22.3229253124378,1.63193266099454));
#27060=CARTESIAN_POINT('Ctrl Pts',(91.6460838609914,-20.3911589633379,1.4739494957459));
#27061=CARTESIAN_POINT('Ctrl Pts',(94.8312242725849,-21.7301456837402,1.31596633049727));
#27062=CARTESIAN_POINT('Ctrl Pts',(95.4433140827682,-25.1332953965992,1.15798316524863));
#27063=CARTESIAN_POINT('Ctrl Pts',(93.7762533017603,-26.7065713079336,1.05266105508288));
#27064=CARTESIAN_POINT('Ctrl Pts',(92.7937992825328,-26.9692229537457,0.999999999999999));
#27065=CARTESIAN_POINT('Ctrl Pts',(93.9134659966651,-22.3640127966251,10.));
#27066=CARTESIAN_POINT('Ctrl Pts',(93.9750770578955,-22.4219120654398,10.));
#27067=CARTESIAN_POINT('Ctrl Pts',(94.0333190151648,-22.4829618973501,10.));
#27068=CARTESIAN_POINT('Ctrl Pts',(94.0881941987852,-22.5467775157033,10.));
#27069=CARTESIAN_POINT('Ctrl Pts',(94.1445220900365,-22.6122825213101,10.));
#27070=CARTESIAN_POINT('Ctrl Pts',(94.19730302831,-22.6807021204397,10.));
#27071=CARTESIAN_POINT('Ctrl Pts',(94.246514026676,-22.7516687130522,10.));
#27072=CARTESIAN_POINT('Ctrl Pts',(94.2970865251706,-22.8245987087286,10.));
#27073=CARTESIAN_POINT('Ctrl Pts',(94.3438893496014,-22.9002191359243,10.));
#27074=CARTESIAN_POINT('Ctrl Pts',(94.3868634537135,-22.9781740458772,10.));
#27075=CARTESIAN_POINT('Ctrl Pts',(94.4057549128497,-23.0124431022373,10.));
#27076=CARTESIAN_POINT('Ctrl Pts',(94.4239059912867,-23.0471637926691,10.));
#27077=CARTESIAN_POINT('Ctrl Pts',(94.4413092551545,-23.0823079492044,10.));
#27078=CARTESIAN_POINT('Ctrl Pts',(94.4512342776001,-23.1023505426566,10.));
#27079=CARTESIAN_POINT('Ctrl Pts',(94.4609160539065,-23.1225308841615,10.));
#27080=CARTESIAN_POINT('Ctrl Pts',(94.4703529715552,-23.1428438969986,10.));
#27081=CARTESIAN_POINT('Ctrl Pts',(94.4788699915235,-23.1611768254387,10.));
#27082=CARTESIAN_POINT('Ctrl Pts',(94.4871899465833,-23.1796235690021,10.));
#27083=CARTESIAN_POINT('Ctrl Pts',(94.4952979566468,-23.1981485647195,10.));
#27084=CARTESIAN_POINT('Ctrl Pts',(94.5318626759043,-23.2816907979364,10.));
#27085=CARTESIAN_POINT('Ctrl Pts',(94.5641670779769,-23.366916527663,10.));
#27086=CARTESIAN_POINT('Ctrl Pts',(94.5921860624412,-23.4534270379695,10.));
#27087=CARTESIAN_POINT('Ctrl Pts',(94.6206677373038,-23.5413661361863,10.));
#27088=CARTESIAN_POINT('Ctrl Pts',(94.6447217851998,-23.6306335527319,10.));
#27089=CARTESIAN_POINT('Ctrl Pts',(94.664282765984,-23.7208476135917,10.));
#27090=CARTESIAN_POINT('Ctrl Pts',(94.6832631734611,-23.8083841054565,10.));
#27091=CARTESIAN_POINT('Ctrl Pts',(94.6980134264571,-23.8968127993399,10.));
#27092=CARTESIAN_POINT('Ctrl Pts',(94.7084329206264,-23.9858069094092,10.));
#27093=CARTESIAN_POINT('Ctrl Pts',(94.7127922670595,-24.0230405936937,10.));
#27094=CARTESIAN_POINT('Ctrl Pts',(94.7163930212393,-24.0603734428421,10.));
#27095=CARTESIAN_POINT('Ctrl Pts',(94.7192254940158,-24.0977821388602,10.));
#27096=CARTESIAN_POINT('Ctrl Pts',(94.7209960695383,-24.121166272346,10.));
#27097=CARTESIAN_POINT('Ctrl Pts',(94.7224664121845,-24.1445800482853,10.));
#27098=CARTESIAN_POINT('Ctrl Pts',(94.7236338650185,-24.168017803389,10.));
#27099=CARTESIAN_POINT('Ctrl Pts',(94.7243181282436,-24.1817550554887,10.));
#27100=CARTESIAN_POINT('Ctrl Pts',(94.724898065248,-24.1954959766469,10.));
#27101=CARTESIAN_POINT('Ctrl Pts',(94.7253731538336,-24.2092311923572,10.));
#27102=CARTESIAN_POINT('Ctrl Pts',(94.7287309598134,-24.306308223558,10.));
#27103=CARTESIAN_POINT('Ctrl Pts',(94.726861580852,-24.4032207088614,10.));
#27104=CARTESIAN_POINT('Ctrl Pts',(94.7197002220053,-24.4995463878866,10.));
#27105=CARTESIAN_POINT('Ctrl Pts',(94.7125388631585,-24.5958720669118,10.));
#27106=CARTESIAN_POINT('Ctrl Pts',(94.7000859592916,-24.6916119941747,10.));
#27107=CARTESIAN_POINT('Ctrl Pts',(94.6822238228945,-24.7863628481204,10.));
#27108=CARTESIAN_POINT('Ctrl Pts',(94.6651462975085,-24.8769516823807,10.));
#27109=CARTESIAN_POINT('Ctrl Pts',(94.6431244275635,-24.9666373988193,10.));
#27110=CARTESIAN_POINT('Ctrl Pts',(94.6164329081479,-25.0551806589533,10.));
#27111=CARTESIAN_POINT('Ctrl Pts',(94.6074980340553,-25.0848201436421,10.));
#27112=CARTESIAN_POINT('Ctrl Pts',(94.5980394679057,-25.1143315742024,10.));
#27113=CARTESIAN_POINT('Ctrl Pts',(94.5880662379456,-25.14370579416,10.));
#27114=CARTESIAN_POINT('Ctrl Pts',(94.5815849548301,-25.1627951600529,10.));
#27115=CARTESIAN_POINT('Ctrl Pts',(94.5748863019078,-25.1818265755599,10.));
#27116=CARTESIAN_POINT('Ctrl Pts',(94.5679726206488,-25.2007974925995,10.));
#27117=CARTESIAN_POINT('Ctrl Pts',(94.5613831132945,-25.2188788869637,10.));
#27118=CARTESIAN_POINT('Ctrl Pts',(94.5545965181257,-25.2369095329808,10.));
#27119=CARTESIAN_POINT('Ctrl Pts',(94.5476256545372,-25.2548600743819,10.));
#27120=CARTESIAN_POINT('Ctrl Pts',(94.5137821755734,-25.3420097887006,10.));
#27121=CARTESIAN_POINT('Ctrl Pts',(94.4755603548741,-25.4273852003437,10.));
#27122=CARTESIAN_POINT('Ctrl Pts',(94.4332913755525,-25.5107526954609,10.));
#27123=CARTESIAN_POINT('Ctrl Pts',(94.3894531453979,-25.5972152383712,10.));
#27124=CARTESIAN_POINT('Ctrl Pts',(94.3412615513892,-25.6815187325337,10.));
#27125=CARTESIAN_POINT('Ctrl Pts',(94.2890300742868,-25.7633995606624,10.));
#27126=CARTESIAN_POINT('Ctrl Pts',(94.2362101788303,-25.8462028245481,10.));
#27127=CARTESIAN_POINT('Ctrl Pts',(94.1792584551776,-25.9265293491613,10.));
#27128=CARTESIAN_POINT('Ctrl Pts',(94.1184473133391,-26.0040916615067,10.));
#27129=CARTESIAN_POINT('Ctrl Pts',(94.0767848210946,-26.0572305952426,10.));
#27130=CARTESIAN_POINT('Ctrl Pts',(94.0333097148272,-26.1090717583023,10.));
#27131=CARTESIAN_POINT('Ctrl Pts',(93.9880973825635,-26.159515663108,10.));
#27132=CARTESIAN_POINT('Ctrl Pts',(93.9759903694326,-26.1730235930748,10.));
#27133=CARTESIAN_POINT('Ctrl Pts',(93.9637574535261,-26.1864325457838,10.));
#27134=CARTESIAN_POINT('Ctrl Pts',(93.9514137007096,-26.199726113673,10.));
#27135=CARTESIAN_POINT('Ctrl Pts',(93.8827528892985,-26.273670170346,10.));
#27136=CARTESIAN_POINT('Ctrl Pts',(93.8105781862797,-26.3441463401416,10.));
#27137=CARTESIAN_POINT('Ctrl Pts',(93.7352000515009,-26.4108648135309,10.));
#27138=CARTESIAN_POINT('Ctrl Pts',(93.6722951821929,-26.4665429868008,10.));
#27139=CARTESIAN_POINT('Ctrl Pts',(93.6071582639901,-26.5196041737296,10.));
#27140=CARTESIAN_POINT('Ctrl Pts',(93.5399460670852,-26.5698661697182,10.));
#27141=CARTESIAN_POINT('Ctrl Pts',(93.5180638151575,-26.5862299505385,10.));
#27142=CARTESIAN_POINT('Ctrl Pts',(93.4959614387476,-26.6022969068259,10.));
#27143=CARTESIAN_POINT('Ctrl Pts',(93.473643921931,-26.6180603652787,10.));
#27144=CARTESIAN_POINT('Ctrl Pts',(93.4508750768599,-26.6341426089371,10.));
#27145=CARTESIAN_POINT('Ctrl Pts',(93.4278768876333,-26.6499123832023,10.));
#27146=CARTESIAN_POINT('Ctrl Pts',(93.4046837833618,-26.6653433745001,10.));
#27147=CARTESIAN_POINT('Ctrl Pts',(93.3197384868702,-26.7218597474537,10.));
#27148=CARTESIAN_POINT('Ctrl Pts',(93.2321269166639,-26.7738756911564,10.));
#27149=CARTESIAN_POINT('Ctrl Pts',(93.1421393365345,-26.8210831412052,10.));
#27150=CARTESIAN_POINT('Ctrl Pts',(93.0588657411436,-26.8647684374332,10.));
#27151=CARTESIAN_POINT('Ctrl Pts',(92.9735566410059,-26.9043362525348,10.));
#27152=CARTESIAN_POINT('Ctrl Pts',(92.8864146397764,-26.9395136119409,10.));
#27153=CARTESIAN_POINT('Ctrl Pts',(92.8563906944762,-26.9516336355772,10.));
#27154=CARTESIAN_POINT('Ctrl Pts',(92.8261489679874,-26.9632321934336,10.));
#27155=CARTESIAN_POINT('Ctrl Pts',(92.7957018439802,-26.9743128659187,10.));
#27156=CARTESIAN_POINT('Ctrl Pts',(89.4817891743669,-24.002194435609,8.38741669750802));
#27157=CARTESIAN_POINT('Ctrl Pts',(89.4802231872165,-24.1747250532131,8.39833391417657));
#27158=CARTESIAN_POINT('Ctrl Pts',(89.4964591581217,-24.3469627518866,8.40925113084511));
#27159=CARTESIAN_POINT('Ctrl Pts',(89.5315887215665,-24.5152564315154,8.42016834751366));
#27160=CARTESIAN_POINT('Ctrl Pts',(89.7010421575268,-25.3270496753528,8.47282940259653));
#27161=CARTESIAN_POINT('Ctrl Pts',(90.3101078559698,-26.0470742874782,8.52549045767941));
#27162=CARTESIAN_POINT('Ctrl Pts',(91.0825656666734,-26.3487966246852,8.57815151276229));
#27163=CARTESIAN_POINT('Ctrl Pts',(91.855023477377,-26.6505189618922,8.63081256784516));
#27164=CARTESIAN_POINT('Ctrl Pts',(92.7908734003413,-26.5339390241808,8.68347362292804));
#27165=CARTESIAN_POINT('Ctrl Pts',(93.4656883820911,-26.0519077734106,8.73613467801092));
#27166=CARTESIAN_POINT('Ctrl Pts',(94.1405033638409,-25.5698765226404,8.7887957330938));
#27167=CARTESIAN_POINT('Ctrl Pts',(94.5542834043762,-24.7223939588114,8.84145678817668));
#27168=CARTESIAN_POINT('Ctrl Pts',(94.5193786114755,-23.8938487978226,8.89411784325956));
#27169=CARTESIAN_POINT('Ctrl Pts',(94.4844738185748,-23.0653036368338,8.94677889834244));
#27170=CARTESIAN_POINT('Ctrl Pts',(94.000884192238,-22.2556958786852,8.99943995342531));
#27171=CARTESIAN_POINT('Ctrl Pts',(93.2879127728201,-21.8321128999534,9.05210100850819));
#27172=CARTESIAN_POINT('Ctrl Pts',(92.5749413534021,-21.4085299212216,9.10476206359107));
#27173=CARTESIAN_POINT('Ctrl Pts',(91.6325881409029,-21.3709717219067,9.15742311867395));
#27174=CARTESIAN_POINT('Ctrl Pts',(90.8882531699407,-21.7366422599482,9.21008417375683));
#27175=CARTESIAN_POINT('Ctrl Pts',(90.1439181989786,-22.1023127979897,9.2627452288397));
#27176=CARTESIAN_POINT('Ctrl Pts',(89.5976014695535,-22.8712120733877,9.31540628392258));
#27177=CARTESIAN_POINT('Ctrl Pts',(89.4970122693619,-23.6942824886892,9.36806733900546));
#27178=CARTESIAN_POINT('Ctrl Pts',(89.4846923712707,-23.7950899672168,9.37451712517298));
#27179=CARTESIAN_POINT('Ctrl Pts',(89.4790586980532,-23.8967100507537,9.3809669113405));
#27180=CARTESIAN_POINT('Ctrl Pts',(89.4798238762261,-23.9984131135314,9.38741669750802));
#27181=CARTESIAN_POINT('Ctrl Pts',(91.2062007174671,-26.9692229537457,10.));
#27182=CARTESIAN_POINT('Ctrl Pts',(90.2237466982397,-26.7065713079336,9.94733894491712));
#27183=CARTESIAN_POINT('Ctrl Pts',(88.5566846367919,-25.1333040393726,9.84201683475137));
#27184=CARTESIAN_POINT('Ctrl Pts',(89.1687768340778,-21.7301430813076,9.68403366950273));
#27185=CARTESIAN_POINT('Ctrl Pts',(92.3539160472627,-20.3911616367203,9.52605050425409));
#27186=CARTESIAN_POINT('Ctrl Pts',(95.215603926767,-22.3229247027849,9.36806733900546));
#27187=CARTESIAN_POINT('Ctrl Pts',(95.1618223030446,-25.7771165220753,9.21008417375683));
#27188=CARTESIAN_POINT('Ctrl Pts',(92.2395757220273,-27.6187839878381,9.0521010085082));
#27189=CARTESIAN_POINT('Ctrl Pts',(89.1003119065523,-26.1783940085773,8.89411784325955));
#27190=CARTESIAN_POINT('Ctrl Pts',(88.5910240312662,-22.7619778387773,8.73613467801093));
#27191=CARTESIAN_POINT('Ctrl Pts',(91.1738623478633,-20.4685627419331,8.57815151276229));
#27192=CARTESIAN_POINT('Ctrl Pts',(94.5060020988175,-21.3782461595948,8.42016834751366));
#27193=CARTESIAN_POINT('Ctrl Pts',(95.5651288739418,-24.665967239189,8.26218518226502));
#27194=CARTESIAN_POINT('Ctrl Pts',(93.3905540118639,-27.3496247591347,8.10420201701638));
#27195=CARTESIAN_POINT('Ctrl Pts',(89.9547031474507,-26.9950624766613,7.94621885176775));
#27196=CARTESIAN_POINT('Ctrl Pts',(88.3740044045685,-23.923874250773,7.78823568651912));
#27197=CARTESIAN_POINT('Ctrl Pts',(90.0822083770022,-20.9217356813897,7.63025252127048));
#27198=CARTESIAN_POINT('Ctrl Pts',(93.5299143458989,-20.7116874252053,7.47226935602185));
#27199=CARTESIAN_POINT('Ctrl Pts',(95.5899360110292,-23.4842511522573,7.31428619077322));
#27200=CARTESIAN_POINT('Ctrl Pts',(94.3937630706594,-26.7246165699189,7.15630302552457));
#27201=CARTESIAN_POINT('Ctrl Pts',(91.0263653754403,-27.4936618194068,6.99831986027595));
#27202=CARTESIAN_POINT('Ctrl Pts',(88.5420874902395,-25.0938365242431,6.84033669502731));
#27203=CARTESIAN_POINT('Ctrl Pts',(89.194254290432,-21.7018641804574,6.68235352977868));
#27204=CARTESIAN_POINT('Ctrl Pts',(92.3913282089151,-20.3943794585145,6.52437036453004));
#27205=CARTESIAN_POINT('Ctrl Pts',(95.2334540881775,-22.3573156385801,6.36638719928141));
#27206=CARTESIAN_POINT('Ctrl Pts',(95.1427267432077,-25.8102226011645,6.20840403403277));
#27207=CARTESIAN_POINT('Ctrl Pts',(92.2014389749,-27.6211958785123,6.05042086878414));
#27208=CARTESIAN_POINT('Ctrl Pts',(89.0774391804456,-26.1476208944803,5.89243770353551));
#27209=CARTESIAN_POINT('Ctrl Pts',(88.604301802773,-22.7260804564427,5.73445453828687));
#27210=CARTESIAN_POINT('Ctrl Pts',(91.2111785923562,-20.4600285259192,5.57647137303824));
#27211=CARTESIAN_POINT('Ctrl Pts',(94.53354332288,-21.4048515492551,5.4184882077896));
#27212=CARTESIAN_POINT('Ctrl Pts',(95.5578977842681,-24.7035627953589,5.26050504254097));
#27213=CARTESIAN_POINT('Ctrl Pts',(93.3551175166525,-27.3641185720073,5.10252187729233));
#27214=CARTESIAN_POINT('Ctrl Pts',(89.9231994083719,-26.9733039791991,4.9445387120437));
#27215=CARTESIAN_POINT('Ctrl Pts',(88.3750103223367,-23.8856011921486,4.78655554679506));
#27216=CARTESIAN_POINT('Ctrl Pts',(90.1148106026499,-20.9016620282348,4.62857238154643));
#27217=CARTESIAN_POINT('Ctrl Pts',(93.5645420118329,-20.7280211581598,4.4705892162978));
#27218=CARTESIAN_POINT('Ctrl Pts',(95.595180415279,-23.5221767762025,4.31260605104916));
#27219=CARTESIAN_POINT('Ctrl Pts',(94.3648674705089,-26.7497343695717,4.15462288580053));
#27220=CARTESIAN_POINT('Ctrl Pts',(90.9895390126931,-27.4831890308961,3.99663972055189));
#27221=CARTESIAN_POINT('Ctrl Pts',(88.5307331581303,-25.0572723617073,3.83865655530326));
#27222=CARTESIAN_POINT('Ctrl Pts',(89.2186707455856,-21.6723735546569,3.68067339005462));
#27223=CARTESIAN_POINT('Ctrl Pts',(92.429368893546,-20.3987114188412,3.52269022480599));
#27224=CARTESIAN_POINT('Ctrl Pts',(95.2506148119859,-22.3915408673733,3.36470705955735));
#27225=CARTESIAN_POINT('Ctrl Pts',(95.1234421205799,-25.8432978095596,3.20672389430872));
#27226=CARTESIAN_POINT('Ctrl Pts',(92.1632008669202,-27.6231203956681,3.04874072906009));
#27227=CARTESIAN_POINT('Ctrl Pts',(89.0549307526673,-26.1166497859116,2.89075756381145));
#27228=CARTESIAN_POINT('Ctrl Pts',(88.6179391794157,-22.6903042108869,2.73277439856282));
#27229=CARTESIAN_POINT('Ctrl Pts',(91.2485917742672,-20.451900203599,2.57479123331418));
#27230=CARTESIAN_POINT('Ctrl Pts',(94.5607981614372,-21.4317381309793,2.41680806806555));
#27231=CARTESIAN_POINT('Ctrl Pts',(95.5502714048858,-24.7410888412383,2.25882490281692));
#27232=CARTESIAN_POINT('Ctrl Pts',(93.3195309927209,-27.3782229777192,2.10084173756828));
#27233=CARTESIAN_POINT('Ctrl Pts',(89.8919234036862,-26.9512419574066,1.94285857231965));
#27234=CARTESIAN_POINT('Ctrl Pts',(88.3764286113539,-23.8472849474598,1.78487540707101));
#27235=CARTESIAN_POINT('Ctrl Pts',(90.1476053652115,-20.8820474355396,1.62689224182238));
#27236=CARTESIAN_POINT('Ctrl Pts',(93.5990313571954,-20.7444874247256,1.46890907657374));
#27237=CARTESIAN_POINT('Ctrl Pts',(95.5999505159819,-23.5606294856849,1.31092591132511));
#27238=CARTESIAN_POINT('Ctrl Pts',(94.33585874306,-26.7735779839873,1.15294274607647));
#27239=CARTESIAN_POINT('Ctrl Pts',(90.9525246480968,-27.4743158223952,0.994959580827838));
#27240=CARTESIAN_POINT('Ctrl Pts',(88.5204066563018,-25.0164786759465,0.836976415579204));
#27241=CARTESIAN_POINT('Ctrl Pts',(89.0030718657857,-22.7756529106096,0.731654305413447));
#27242=CARTESIAN_POINT('Ctrl Pts',(89.6639373423039,-22.0026984430693,0.678993250330568));
#27243=CARTESIAN_POINT('Ctrl Pts',(91.254067145653,-26.7901775698421,10.1070022498898));
#27244=CARTESIAN_POINT('Ctrl Pts',(90.3308555140066,-26.5433639279422,10.0543411948069));
#27245=CARTESIAN_POINT('Ctrl Pts',(88.7643179909425,-25.0649653325897,9.94901908464118));
#27246=CARTESIAN_POINT('Ctrl Pts',(89.3395007731539,-21.8670164012787,9.79103591939254));
#27247=CARTESIAN_POINT('Ctrl Pts',(92.332574761836,-20.6087760968887,9.63305275414391));
#27248=CARTESIAN_POINT('Ctrl Pts',(95.0217016673144,-22.4240530434662,9.47506958889527));
#27249=CARTESIAN_POINT('Ctrl Pts',(94.9711630979589,-25.669955653763,9.31708642364664));
#27250=CARTESIAN_POINT('Ctrl Pts',(92.2251292059548,-27.400569802356,9.159103258398));
#27251=CARTESIAN_POINT('Ctrl Pts',(89.2751643093457,-26.0470359402764,9.00112009314937));
#27252=CARTESIAN_POINT('Ctrl Pts',(88.7965867055915,-22.8366310920326,8.84313692790073));
#27253=CARTESIAN_POINT('Ctrl Pts',(91.2236787932393,-20.6815098831386,8.6851537626521));
#27254=CARTESIAN_POINT('Ctrl Pts',(94.354889125883,-21.536339010879,8.52717059740346));
#27255=CARTESIAN_POINT('Ctrl Pts',(95.3501501142311,-24.6258091365927,8.36918743215484));
#27256=CARTESIAN_POINT('Ctrl Pts',(93.3067030243257,-27.1476409875303,8.21120426690619));
#27257=CARTESIAN_POINT('Ctrl Pts',(90.0780354016687,-26.8144589587366,8.05322110165756));
#27258=CARTESIAN_POINT('Ctrl Pts',(88.5926534529997,-23.9284646652375,7.89523793640893));
#27259=CARTESIAN_POINT('Ctrl Pts',(90.1978520126387,-21.1073563051245,7.7372547711603));
#27260=CARTESIAN_POINT('Ctrl Pts',(93.4376598720287,-20.9099740464933,7.57927160591166));
#27261=CARTESIAN_POINT('Ctrl Pts',(95.3734613705941,-23.515351023126,7.42128844066303));
#27262=CARTESIAN_POINT('Ctrl Pts',(94.249418157988,-26.560321053095,7.26330527541439));
#27263=CARTESIAN_POINT('Ctrl Pts',(91.0850759498403,-27.2829925529256,7.10532211016575));
#27264=CARTESIAN_POINT('Ctrl Pts',(88.750601058422,-25.0278777251021,6.94733894491712));
#27265=CARTESIAN_POINT('Ctrl Pts',(89.363441928252,-21.8404427299575,6.78935577966849));
#27266=CARTESIAN_POINT('Ctrl Pts',(92.3677309545194,-20.6117998826853,6.63137261441986));
#27267=CARTESIAN_POINT('Ctrl Pts',(95.0384754565385,-22.456370191473,6.47338944917121));
#27268=CARTESIAN_POINT('Ctrl Pts',(94.9532190083536,-25.7010654224598,6.31540628392259));
#27269=CARTESIAN_POINT('Ctrl Pts',(92.189292120603,-27.4028362550155,6.15742311867395));
#27270=CARTESIAN_POINT('Ctrl Pts',(89.2536708181738,-26.0181184578087,5.99943995342532));
#27271=CARTESIAN_POINT('Ctrl Pts',(88.8090638219323,-22.8028983368416,5.84145678817668));
#27272=CARTESIAN_POINT('Ctrl Pts',(91.2587448526078,-20.6734902839138,5.68347362292805));
#27273=CARTESIAN_POINT('Ctrl Pts',(94.3807696026347,-21.5613400844336,5.52549045767941));
#27274=CARTESIAN_POINT('Ctrl Pts',(95.3433550622842,-24.6611376650276,5.36750729243078));
#27275=CARTESIAN_POINT('Ctrl Pts',(93.273403364572,-27.1612608174348,5.20952412718215));
#27276=CARTESIAN_POINT('Ctrl Pts',(90.0484313512107,-26.7940125077567,5.05154096193351));
#27277=CARTESIAN_POINT('Ctrl Pts',(88.5935987135065,-23.892499488029,4.89355779668487));
#27278=CARTESIAN_POINT('Ctrl Pts',(90.2284883104669,-21.0884931016366,4.73557463143624));
#27279=CARTESIAN_POINT('Ctrl Pts',(93.4701994752482,-20.9253228485305,4.57759146618761));
#27280=CARTESIAN_POINT('Ctrl Pts',(95.3783895350779,-23.5509897161116,4.41960830093897));
#27281=CARTESIAN_POINT('Ctrl Pts',(94.2222649745917,-26.5839242389408,4.26162513569034));
#27282=CARTESIAN_POINT('Ctrl Pts',(91.0504702321437,-27.273151277935,4.1036419704417));
#27283=CARTESIAN_POINT('Ctrl Pts',(88.73993139728,-24.9935183968346,3.94565880519307));
#27284=CARTESIAN_POINT('Ctrl Pts',(89.3863860609648,-21.8127304012065,3.78767563994443));
#27285=CARTESIAN_POINT('Ctrl Pts',(92.4034777699831,-20.6158706239954,3.6296924746958));
#27286=CARTESIAN_POINT('Ctrl Pts',(95.0546013815359,-22.4885316246793,3.47170930944716));
#27287=CARTESIAN_POINT('Ctrl Pts',(94.9350972565224,-25.7321461819781,3.31372614419853));
#27288=CARTESIAN_POINT('Ctrl Pts',(92.1533597865007,-27.4046447229832,3.1557429789499));
#27289=CARTESIAN_POINT('Ctrl Pts',(89.2325196579888,-25.9890149200186,2.99775981370126));
#27290=CARTESIAN_POINT('Ctrl Pts',(88.8218788590692,-22.7692794138311,2.83977664845263));
#27291=CARTESIAN_POINT('Ctrl Pts',(91.2939020040278,-20.6658521028235,2.681793483204));
#27292=CARTESIAN_POINT('Ctrl Pts',(94.4063809630467,-21.5866053940535,2.52381031795536));
#27293=CARTESIAN_POINT('Ctrl Pts',(95.336188556763,-24.6964008746715,2.36582715270673));
#27294=CARTESIAN_POINT('Ctrl Pts',(93.2399627228925,-27.174514721593,2.20784398745809));
#27295=CARTESIAN_POINT('Ctrl Pts',(90.0190413026668,-26.7732808350902,2.04986082220945));
#27296=CARTESIAN_POINT('Ctrl Pts',(88.5949314791037,-23.8564937288939,1.89187765696082));
#27297=CARTESIAN_POINT('Ctrl Pts',(90.2593055351526,-21.070061277071,1.73389449171219));
#27298=CARTESIAN_POINT('Ctrl Pts',(93.5026090986844,-20.9407961923469,1.57591132646355));
#27299=CARTESIAN_POINT('Ctrl Pts',(95.3828719967165,-23.5871237111563,1.41792816121492));
#27300=CARTESIAN_POINT('Ctrl Pts',(94.1950054855208,-26.6063300734514,1.25994499596628));
#27301=CARTESIAN_POINT('Ctrl Pts',(91.0156878491876,-27.2648131276116,1.10196183071765));
#27302=CARTESIAN_POINT('Ctrl Pts',(88.7302275878235,-24.9551845873584,0.943978665469013));
#27303=CARTESIAN_POINT('Ctrl Pts',(89.1837878836397,-22.8494815513233,0.838656555303258));
#27304=CARTESIAN_POINT('Ctrl Pts',(89.8048028959809,-22.1231365609212,0.785995500220379));
#27305=CARTESIAN_POINT('Ctrl Pts',(91.301933573839,-26.6111321859386,10.2140044997796));
#27306=CARTESIAN_POINT('Ctrl Pts',(90.4379643297735,-26.3801565479507,10.1613434446967));
#27307=CARTESIAN_POINT('Ctrl Pts',(88.9719513450928,-24.9966266258069,10.056021334531));
#27308=CARTESIAN_POINT('Ctrl Pts',(89.5102247122303,-22.0038897212497,9.89803816928235));
#27309=CARTESIAN_POINT('Ctrl Pts',(92.3112334764091,-20.8263905570572,9.74005500403372));
#27310=CARTESIAN_POINT('Ctrl Pts',(94.8277994078618,-22.5251813841475,9.58207183878509));
#27311=CARTESIAN_POINT('Ctrl Pts',(94.7805038928732,-25.5627947854507,9.42408867353645));
#27312=CARTESIAN_POINT('Ctrl Pts',(92.2106826898821,-27.1823556168738,9.26610550828782));
#27313=CARTESIAN_POINT('Ctrl Pts',(89.4500167121391,-25.9156778719754,9.10812234303918));
#27314=CARTESIAN_POINT('Ctrl Pts',(89.0021493799168,-22.9112843452878,8.95013917779054));
#27315=CARTESIAN_POINT('Ctrl Pts',(91.2734952386149,-20.8944570243441,8.79215601254192));
#27316=CARTESIAN_POINT('Ctrl Pts',(94.2037761529487,-21.6944318621631,8.63417284729327));
#27317=CARTESIAN_POINT('Ctrl Pts',(95.1351713545205,-24.5856510339964,8.47618968204465));
#27318=CARTESIAN_POINT('Ctrl Pts',(93.2228520367874,-26.9456572159258,8.31820651679601));
#27319=CARTESIAN_POINT('Ctrl Pts',(90.2013676558868,-26.6338554408121,8.16022335154738));
#27320=CARTESIAN_POINT('Ctrl Pts',(88.8113025014309,-23.933055079702,8.00224018629874));
#27321=CARTESIAN_POINT('Ctrl Pts',(90.3134956482753,-21.2929769288594,7.84425702105011));
#27322=CARTESIAN_POINT('Ctrl Pts',(93.3454053981585,-21.1082606677813,7.68627385580147));
#27323=CARTESIAN_POINT('Ctrl Pts',(95.156986730159,-23.5464508939947,7.52829069055284));
#27324=CARTESIAN_POINT('Ctrl Pts',(94.1050732453165,-26.3960255362711,7.37030752530419));
#27325=CARTESIAN_POINT('Ctrl Pts',(91.1437865242403,-27.0723232864443,7.21232436005558));
#27326=CARTESIAN_POINT('Ctrl Pts',(88.9591146266045,-24.9619189259611,7.05434119480693));
#27327=CARTESIAN_POINT('Ctrl Pts',(89.5326295660721,-21.9790212794576,6.8963580295583));
#27328=CARTESIAN_POINT('Ctrl Pts',(92.3441337001234,-20.8292203068559,6.73837486430967));
#27329=CARTESIAN_POINT('Ctrl Pts',(94.8434968248997,-22.555424744366,6.58039169906103));
#27330=CARTESIAN_POINT('Ctrl Pts',(94.7637112734992,-25.591908243755,6.4224085338124));
#27331=CARTESIAN_POINT('Ctrl Pts',(92.1771452663062,-27.1844766315186,6.26442536856375));
#27332=CARTESIAN_POINT('Ctrl Pts',(89.4299024559019,-25.888616021137,6.10644220331513));
#27333=CARTESIAN_POINT('Ctrl Pts',(89.0138258410916,-22.8797162172404,5.94845903806648));
#27334=CARTESIAN_POINT('Ctrl Pts',(91.3063111128593,-20.8869520419083,5.79047587281787));
#27335=CARTESIAN_POINT('Ctrl Pts',(94.2279958823895,-21.7178286196122,5.63249270756922));
#27336=CARTESIAN_POINT('Ctrl Pts',(95.1288123403003,-24.6187125346963,5.47450954232059));
#27337=CARTESIAN_POINT('Ctrl Pts',(93.1916892124914,-26.9584030628623,5.31652637707196));
#27338=CARTESIAN_POINT('Ctrl Pts',(90.1736632940495,-26.6147210363142,5.15854321182332));
#27339=CARTESIAN_POINT('Ctrl Pts',(88.8121871046762,-23.8993977839094,5.00056004657468));
#27340=CARTESIAN_POINT('Ctrl Pts',(90.342166018284,-21.2753241750384,4.84257688132606));
#27341=CARTESIAN_POINT('Ctrl Pts',(93.3758569386635,-21.1226245389013,4.68459371607742));
#27342=CARTESIAN_POINT('Ctrl Pts',(95.1615986548766,-23.5798026560206,4.52661055082878));
#27343=CARTESIAN_POINT('Ctrl Pts',(94.0796624786748,-26.41811410831,4.36862738558015));
#27344=CARTESIAN_POINT('Ctrl Pts',(91.1114014515939,-27.0631135249739,4.21064422033152));
#27345=CARTESIAN_POINT('Ctrl Pts',(88.9491296364298,-24.9297644319618,4.05266105508287));
#27346=CARTESIAN_POINT('Ctrl Pts',(89.5541013763441,-21.9530872477561,3.89467788983425));
#27347=CARTESIAN_POINT('Ctrl Pts',(92.3775866464202,-20.8330298291496,3.73669472458561));
#27348=CARTESIAN_POINT('Ctrl Pts',(94.858587951086,-22.5855223819854,3.57871155933698));
#27349=CARTESIAN_POINT('Ctrl Pts',(94.7467523924648,-25.6209945543966,3.42072839408834));
#27350=CARTESIAN_POINT('Ctrl Pts',(92.1435187060813,-27.1861690502982,3.26274522883971));
#27351=CARTESIAN_POINT('Ctrl Pts',(89.4101085633103,-25.8613800541255,3.10476206359107));
#27352=CARTESIAN_POINT('Ctrl Pts',(89.0258185387226,-22.8482546167753,2.94677889834244));
#27353=CARTESIAN_POINT('Ctrl Pts',(91.3392122337884,-20.8798040020479,2.78879573309381));
#27354=CARTESIAN_POINT('Ctrl Pts',(94.2519637646563,-21.7414726571277,2.63081256784517));
#27355=CARTESIAN_POINT('Ctrl Pts',(95.1221057086401,-24.6517129081048,2.47282940259654));
#27356=CARTESIAN_POINT('Ctrl Pts',(93.1603944530641,-26.9708064654667,2.3148462373479));
#27357=CARTESIAN_POINT('Ctrl Pts',(90.1461592016474,-26.5953197127739,2.15686307209927));
#27358=CARTESIAN_POINT('Ctrl Pts',(88.8134343468535,-23.8657025103278,1.99887990685063));
#27359=CARTESIAN_POINT('Ctrl Pts',(90.3710057050937,-21.2580751186024,1.840896741602));
#27360=CARTESIAN_POINT('Ctrl Pts',(93.4061868401735,-21.1371049599683,1.68291357635336));
#27361=CARTESIAN_POINT('Ctrl Pts',(95.1657934774511,-23.6136179366278,1.52493041110473));
#27362=CARTESIAN_POINT('Ctrl Pts',(94.0541522279815,-26.4390821629154,1.3669472458561));
#27363=CARTESIAN_POINT('Ctrl Pts',(91.0788510502784,-27.0553104328281,1.20896408060746));
#27364=CARTESIAN_POINT('Ctrl Pts',(88.9400485193453,-24.8938904987703,1.05098091535883));
#27365=CARTESIAN_POINT('Ctrl Pts',(89.3645039014938,-22.9233101920371,0.945658805193069));
#27366=CARTESIAN_POINT('Ctrl Pts',(89.9456684496579,-22.2435746787732,0.89299775011019));
#27367=CARTESIAN_POINT('Ctrl Pts',(91.3498000020249,-26.4320868020351,10.3210067496694));
#27368=CARTESIAN_POINT('Ctrl Pts',(90.5450731455404,-26.2169491679593,10.2683456945866));
#27369=CARTESIAN_POINT('Ctrl Pts',(89.1795846992432,-24.9282879190241,10.1630235844208));
#27370=CARTESIAN_POINT('Ctrl Pts',(89.6809486513065,-22.1407630412207,10.0050404191722));
#27371=CARTESIAN_POINT('Ctrl Pts',(92.2898921909823,-21.0440050172257,9.84705725392353));
#27372=CARTESIAN_POINT('Ctrl Pts',(94.6338971484091,-22.6263097248287,9.68907408867489));
#27373=CARTESIAN_POINT('Ctrl Pts',(94.5898446877876,-25.4556339171384,9.53109092342626));
#27374=CARTESIAN_POINT('Ctrl Pts',(92.1962361738095,-26.9641414313917,9.37310775817763));
#27375=CARTESIAN_POINT('Ctrl Pts',(89.6248691149327,-25.7843198036745,9.21512459292898));
#27376=CARTESIAN_POINT('Ctrl Pts',(89.207712054242,-22.985937598543,9.05714142768036));
#27377=CARTESIAN_POINT('Ctrl Pts',(91.3233116839909,-21.1074041655496,8.89915826243172));
#27378=CARTESIAN_POINT('Ctrl Pts',(94.052663180014,-21.8525247134472,8.74117509718308));
#27379=CARTESIAN_POINT('Ctrl Pts',(94.9201925948099,-24.5454929314001,8.58319193193446));
#27380=CARTESIAN_POINT('Ctrl Pts',(93.1390010492492,-26.7436734443214,8.42520876668581));
#27381=CARTESIAN_POINT('Ctrl Pts',(90.3246999101047,-26.4532519228875,8.26722560143719));
#27382=CARTESIAN_POINT('Ctrl Pts',(89.0299515498622,-23.9376454941666,8.10924243618855));
#27383=CARTESIAN_POINT('Ctrl Pts',(90.4291392839118,-21.4785975525943,7.95125927093992));
#27384=CARTESIAN_POINT('Ctrl Pts',(93.2531509242885,-21.3065472890693,7.79327610569128));
#27385=CARTESIAN_POINT('Ctrl Pts',(94.9405120897237,-23.5775507648634,7.63529294044265));
#27386=CARTESIAN_POINT('Ctrl Pts',(93.9607283326452,-26.2317300194472,7.47730977519401));
#27387=CARTESIAN_POINT('Ctrl Pts',(91.2024970986403,-26.8616540199631,7.31932660994538));
#27388=CARTESIAN_POINT('Ctrl Pts',(89.167628194787,-24.8959601268202,7.16134344469675));
#27389=CARTESIAN_POINT('Ctrl Pts',(89.7018172038921,-22.1175998289577,7.00336027944811));
#27390=CARTESIAN_POINT('Ctrl Pts',(92.3205364457276,-21.0466407310267,6.84537711419948));
#27391=CARTESIAN_POINT('Ctrl Pts',(94.6485181932608,-22.6544792972589,6.68739394895083));
#27392=CARTESIAN_POINT('Ctrl Pts',(94.574203538645,-25.4827510650502,6.52941078370221));
#27393=CARTESIAN_POINT('Ctrl Pts',(92.1649984120093,-26.9661170080217,6.37142761845357));
#27394=CARTESIAN_POINT('Ctrl Pts',(89.6061340936301,-25.7591135844653,6.21344445320494));
#27395=CARTESIAN_POINT('Ctrl Pts',(89.2185878602508,-22.9565340976394,6.0554612879563));
#27396=CARTESIAN_POINT('Ctrl Pts',(91.353877373111,-21.1004137999029,5.89747812270767));
#27397=CARTESIAN_POINT('Ctrl Pts',(94.0752221621442,-21.8743171547908,5.73949495745903));
#27398=CARTESIAN_POINT('Ctrl Pts',(94.9142696183164,-24.576287404365,5.5815117922104));
#27399=CARTESIAN_POINT('Ctrl Pts',(93.1099750604108,-26.7555453082897,5.42352862696177));
#27400=CARTESIAN_POINT('Ctrl Pts',(90.2988952368883,-26.4354295648718,5.26554546171313));
#27401=CARTESIAN_POINT('Ctrl Pts',(89.0307754958461,-23.9062960797898,5.10756229646449));
#27402=CARTESIAN_POINT('Ctrl Pts',(90.4558437261009,-21.4621552484402,4.94957913121587));
#27403=CARTESIAN_POINT('Ctrl Pts',(93.2815144020789,-21.319926229272,4.79159596596723));
#27404=CARTESIAN_POINT('Ctrl Pts',(94.9448077746754,-23.6086155959297,4.6336128007186));
#27405=CARTESIAN_POINT('Ctrl Pts',(93.9370599827578,-26.2523039776791,4.47562963546996));
#27406=CARTESIAN_POINT('Ctrl Pts',(91.1723326710444,-26.8530757720127,4.31764647022133));
#27407=CARTESIAN_POINT('Ctrl Pts',(89.1583278755794,-24.8660104670891,4.15966330497269));
#27408=CARTESIAN_POINT('Ctrl Pts',(89.7218166917233,-22.0934440943058,4.00168013972406));
#27409=CARTESIAN_POINT('Ctrl Pts',(92.3516955228573,-21.0501890343038,3.84369697447542));
#27410=CARTESIAN_POINT('Ctrl Pts',(94.6625745206359,-22.6825131392915,3.68571380922679));
#27411=CARTESIAN_POINT('Ctrl Pts',(94.5584075284074,-25.5098429268151,3.52773064397815));
#27412=CARTESIAN_POINT('Ctrl Pts',(92.1336776256617,-26.9676933776133,3.36974747872952));
#27413=CARTESIAN_POINT('Ctrl Pts',(89.5876974686318,-25.7337451882325,3.21176431348088));
#27414=CARTESIAN_POINT('Ctrl Pts',(89.2297582183761,-22.9272298197195,3.05378114823225));
#27415=CARTESIAN_POINT('Ctrl Pts',(91.384522463549,-21.0937559012723,2.89579798298361));
#27416=CARTESIAN_POINT('Ctrl Pts',(94.0975465662658,-21.8963399202019,2.73781481773498));
#27417=CARTESIAN_POINT('Ctrl Pts',(94.9080228605173,-24.6070249415381,2.57983165248635));
#27418=CARTESIAN_POINT('Ctrl Pts',(93.0808261832357,-26.7670982093405,2.42184848723771));
#27419=CARTESIAN_POINT('Ctrl Pts',(90.273277100628,-26.4173585904575,2.26386532198908));
#27420=CARTESIAN_POINT('Ctrl Pts',(89.0319372146034,-23.8749112917619,2.10588215674044));
#27421=CARTESIAN_POINT('Ctrl Pts',(90.4827058750349,-21.4460889601337,1.94789899149181));
#27422=CARTESIAN_POINT('Ctrl Pts',(93.3097645816624,-21.3334137275896,1.78991582624317));
#27423=CARTESIAN_POINT('Ctrl Pts',(94.9487149581859,-23.6401121620991,1.63193266099454));
#27424=CARTESIAN_POINT('Ctrl Pts',(93.9132989704421,-26.2718342523794,1.47394949574591));
#27425=CARTESIAN_POINT('Ctrl Pts',(91.1420142513693,-26.8458077380446,1.31596633049727));
#27426=CARTESIAN_POINT('Ctrl Pts',(89.149869450867,-24.8325964101823,1.15798316524864));
#27427=CARTESIAN_POINT('Ctrl Pts',(89.5452199193478,-22.9971388327508,1.05266105508288));
#27428=CARTESIAN_POINT('Ctrl Pts',(90.0865340033349,-22.3640127966251,1.));
#27429=CARTESIAN_POINT('Ctrl Pts',(89.4850512338518,-23.9982506073194,9.11258330249198));
#27430=CARTESIAN_POINT('Ctrl Pts',(89.4831441979475,-23.7052247997765,9.09410267755477));
#27431=CARTESIAN_POINT('Ctrl Pts',(89.5304975843651,-23.4127948855722,9.07562205261757));
#27432=CARTESIAN_POINT('Ctrl Pts',(89.6298381693152,-23.1392457272327,9.05714142768036));
#27433=CARTESIAN_POINT('Ctrl Pts',(89.9129119308249,-22.3597597875452,9.00448037259748));
#27434=CARTESIAN_POINT('Ctrl Pts',(90.6181118074079,-21.7335819765474,8.9518193175146));
#27435=CARTESIAN_POINT('Ctrl Pts',(91.4256036617033,-21.5446798290314,8.89915826243172));
#27436=CARTESIAN_POINT('Ctrl Pts',(92.2330955159986,-21.3557776815155,8.84649720734885));
#27437=CARTESIAN_POINT('Ctrl Pts',(93.1428793480063,-21.6041511974813,8.79383615226596));
#27438=CARTESIAN_POINT('Ctrl Pts',(93.7423594998095,-22.1771659917897,8.74117509718309));
#27439=CARTESIAN_POINT('Ctrl Pts',(94.3418396516127,-22.7501807860982,8.68851404210021));
#27440=CARTESIAN_POINT('Ctrl Pts',(94.6310161232113,-23.6478368587491,8.63585298701733));
#27441=CARTESIAN_POINT('Ctrl Pts',(94.4787391014172,-24.4630283138948,8.58319193193445));
#27442=CARTESIAN_POINT('Ctrl Pts',(94.326462079623,-25.2782197690405,8.53053087685158));
#27443=CARTESIAN_POINT('Ctrl Pts',(93.7327315644362,-26.0109466066809,8.4778698217687));
#27444=CARTESIAN_POINT('Ctrl Pts',(92.9668161169853,-26.3289064385955,8.42520876668582));
#27445=CARTESIAN_POINT('Ctrl Pts',(92.2009006695344,-26.6468662705101,8.37254771160294));
#27446=CARTESIAN_POINT('Ctrl Pts',(91.2628002898196,-26.5500590966988,8.31988665652006));
#27447=CARTESIAN_POINT('Ctrl Pts',(90.5779587065884,-26.082387771673,8.26722560143718));
#27448=CARTESIAN_POINT('Ctrl Pts',(89.907599452313,-25.624606281228,8.21567816845545));
#27449=CARTESIAN_POINT('Ctrl Pts',(89.4799009347916,-24.8114801021923,8.16413073547372));
#27450=CARTESIAN_POINT('Ctrl Pts',(89.4784371162896,-23.999680408535,8.11258330249198));
#27451=CARTESIAN_POINT('Ctrl Pts',(91.2062007174671,-26.9692229537457,10.));
#27452=CARTESIAN_POINT('Ctrl Pts',(91.1131474716668,-26.9351836607658,10.));
#27453=CARTESIAN_POINT('Ctrl Pts',(91.0221595031901,-26.8963760597068,10.));
#27454=CARTESIAN_POINT('Ctrl Pts',(90.9334453118182,-26.8531283773235,10.));
#27455=CARTESIAN_POINT('Ctrl Pts',(90.8427654821472,-26.8089224570357,10.));
#27456=CARTESIAN_POINT('Ctrl Pts',(90.7544606379728,-26.7600769016029,10.));
#27457=CARTESIAN_POINT('Ctrl Pts',(90.668782366846,-26.7068967029855,10.));
#27458=CARTESIAN_POINT('Ctrl Pts',(90.5863298883847,-26.6557187424198,10.));
#27459=CARTESIAN_POINT('Ctrl Pts',(90.5063096394357,-26.6005255181573,10.));
#27460=CARTESIAN_POINT('Ctrl Pts',(90.4289788439406,-26.5415587834304,10.));
#27461=CARTESIAN_POINT('Ctrl Pts',(90.3613143978823,-26.4899628905444,10.));
#27462=CARTESIAN_POINT('Ctrl Pts',(90.2957093551107,-26.435477205689,10.));
#27463=CARTESIAN_POINT('Ctrl Pts',(90.2323606826138,-26.3782509736031,10.));
#27464=CARTESIAN_POINT('Ctrl Pts',(90.2182619575677,-26.3655148438658,10.));
#27465=CARTESIAN_POINT('Ctrl Pts',(90.2042723901541,-26.3526402704889,10.));
#27466=CARTESIAN_POINT('Ctrl Pts',(90.190413624506,-26.339647326439,10.));
#27467=CARTESIAN_POINT('Ctrl Pts',(90.117982895404,-26.2717416821266,10.));
#27468=CARTESIAN_POINT('Ctrl Pts',(90.0490178395273,-26.2005142871037,10.));
#27469=CARTESIAN_POINT('Ctrl Pts',(89.9837584040089,-26.1262557408025,10.));
#27470=CARTESIAN_POINT('Ctrl Pts',(89.9188586588048,-26.0524064851986,10.));
#27471=CARTESIAN_POINT('Ctrl Pts',(89.8576233116514,-25.9755586030621,10.));
#27472=CARTESIAN_POINT('Ctrl Pts',(89.8003319724653,-25.8959711475448,10.));
#27473=CARTESIAN_POINT('Ctrl Pts',(89.7451391407445,-25.8192988773226,10.));
#27474=CARTESIAN_POINT('Ctrl Pts',(89.6936065132557,-25.7400833150341,10.));
#27475=CARTESIAN_POINT('Ctrl Pts',(89.6460290163529,-25.6585424655959,10.));
#27476=CARTESIAN_POINT('Ctrl Pts',(89.626040255569,-25.6242846622301,10.));
#27477=CARTESIAN_POINT('Ctrl Pts',(89.6067501857345,-25.5896163159409,10.));
#27478=CARTESIAN_POINT('Ctrl Pts',(89.5881832814499,-25.5545532938095,10.));
#27479=CARTESIAN_POINT('Ctrl Pts',(89.5751467282293,-25.529934167913,10.));
#27480=CARTESIAN_POINT('Ctrl Pts',(89.5624667280368,-25.505120464169,10.));
#27481=CARTESIAN_POINT('Ctrl Pts',(89.5501522393051,-25.4801176691506,10.));
#27482=CARTESIAN_POINT('Ctrl Pts',(89.5423997338152,-25.4643773237844,10.));
#27483=CARTESIAN_POINT('Ctrl Pts',(89.5347912129438,-25.4485599130764,10.));
#27484=CARTESIAN_POINT('Ctrl Pts',(89.5273385775824,-25.4326879328603,10.));
#27485=CARTESIAN_POINT('Ctrl Pts',(89.4852180064675,-25.3429831721955,10.));
#27486=CARTESIAN_POINT('Ctrl Pts',(89.4479996497494,-25.2513937089187,10.));
#27487=CARTESIAN_POINT('Ctrl Pts',(89.4159751546784,-25.1581920045764,10.));
#27488=CARTESIAN_POINT('Ctrl Pts',(89.3861126932969,-25.0712825219929,10.));
#27489=CARTESIAN_POINT('Ctrl Pts',(89.3607666485969,-24.9829703487333,10.));
#27490=CARTESIAN_POINT('Ctrl Pts',(89.3402240440734,-24.8934677198076,10.));
#27491=CARTESIAN_POINT('Ctrl Pts',(89.3387367653631,-24.8869877549932,10.));
#27492=CARTESIAN_POINT('Ctrl Pts',(89.337274687697,-24.8805015489785,10.));
#27493=CARTESIAN_POINT('Ctrl Pts',(89.335837930805,-24.874009181989,10.));
#27494=CARTESIAN_POINT('Ctrl Pts',(89.315252334091,-24.7809877047218,10.));
#27495=CARTESIAN_POINT('Ctrl Pts',(89.2998605243042,-24.6867004764278,10.));
#27496=CARTESIAN_POINT('Ctrl Pts',(89.2895854935825,-24.5915555250827,10.));
#27497=CARTESIAN_POINT('Ctrl Pts',(89.2837678665547,-24.5376853367106,10.));
#27498=CARTESIAN_POINT('Ctrl Pts',(89.279591470324,-24.4835403753464,10.));
#27499=CARTESIAN_POINT('Ctrl Pts',(89.2770492198354,-24.4291973958018,10.));
#27500=CARTESIAN_POINT('Ctrl Pts',(89.2764018813574,-24.4153599309944,10.));
#27501=CARTESIAN_POINT('Ctrl Pts',(89.2758606481526,-24.4015110330491,10.));
#27502=CARTESIAN_POINT('Ctrl Pts',(89.2754255840287,-24.3876642045987,10.));
#27503=CARTESIAN_POINT('Ctrl Pts',(89.2724967852974,-24.2944490407395,10.));
#27504=CARTESIAN_POINT('Ctrl Pts',(89.2743673782132,-24.2011765909983,10.));
#27505=CARTESIAN_POINT('Ctrl Pts',(89.2809024940859,-24.1082221294119,10.));
#27506=CARTESIAN_POINT('Ctrl Pts',(89.287448047592,-24.0151192045669,10.));
#27507=CARTESIAN_POINT('Ctrl Pts',(89.2986734147484,-23.9223343048006,10.));
#27508=CARTESIAN_POINT('Ctrl Pts',(89.3144939864412,-23.8302566591467,10.));
#27509=CARTESIAN_POINT('Ctrl Pts',(89.3300873891373,-23.7395011646005,10.));
#27510=CARTESIAN_POINT('Ctrl Pts',(89.3501454394382,-23.649431915389,10.));
#27511=CARTESIAN_POINT('Ctrl Pts',(89.3746301066029,-23.5604468626945,10.));
#27512=CARTESIAN_POINT('Ctrl Pts',(89.3838721758798,-23.5268582492132,10.));
#27513=CARTESIAN_POINT('Ctrl Pts',(89.3937453511447,-23.4934244350543,10.));
#27514=CARTESIAN_POINT('Ctrl Pts',(89.4042490107015,-23.4601681503182,10.));
#27515=CARTESIAN_POINT('Ctrl Pts',(89.4119449034304,-23.4358017094118,10.));
#27516=CARTESIAN_POINT('Ctrl Pts',(89.4199792749368,-23.4115305873094,10.));
#27517=CARTESIAN_POINT('Ctrl Pts',(89.4283521276576,-23.3873640207246,10.));
#27518=CARTESIAN_POINT('Ctrl Pts',(89.4335196879868,-23.3724488902498,10.));
#27519=CARTESIAN_POINT('Ctrl Pts',(89.4388131892276,-23.3575822733592,10.));
#27520=CARTESIAN_POINT('Ctrl Pts',(89.4442314440759,-23.3427682606429,10.));
#27521=CARTESIAN_POINT('Ctrl Pts',(89.4759375039964,-23.2560809437852,10.));
#27522=CARTESIAN_POINT('Ctrl Pts',(89.511920335114,-23.1711677991127,10.));
#27523=CARTESIAN_POINT('Ctrl Pts',(89.5521196351583,-23.0884296536704,10.));
#27524=CARTESIAN_POINT('Ctrl Pts',(89.5822691101916,-23.0263760445887,10.));
#27525=CARTESIAN_POINT('Ctrl Pts',(89.6147913381275,-22.9655463574365,10.));
#27526=CARTESIAN_POINT('Ctrl Pts',(89.6496759688728,-22.9061246870224,10.));
#27527=CARTESIAN_POINT('Ctrl Pts',(89.6654548106757,-22.8792473740884,10.));
#27528=CARTESIAN_POINT('Ctrl Pts',(89.6817171385687,-22.8526583245227,10.));
#27529=CARTESIAN_POINT('Ctrl Pts',(89.6984627751052,-22.8263756432691,10.));
#27530=CARTESIAN_POINT('Ctrl Pts',(89.7075848157606,-22.8120583799984,10.));
#27531=CARTESIAN_POINT('Ctrl Pts',(89.7168450962946,-22.7978401889566,10.));
#27532=CARTESIAN_POINT('Ctrl Pts',(89.726242936913,-22.7837240829482,10.));
#27533=CARTESIAN_POINT('Ctrl Pts',(89.7738179917087,-22.7122635693982,10.));
#27534=CARTESIAN_POINT('Ctrl Pts',(89.8249182481167,-22.6434123197201,10.));
#27535=CARTESIAN_POINT('Ctrl Pts',(89.8795126484078,-22.577523824193,10.));
#27536=CARTESIAN_POINT('Ctrl Pts',(89.9256431731806,-22.5218501496231,10.));
#27537=CARTESIAN_POINT('Ctrl Pts',(89.974269092162,-22.4682921528781,10.));
#27538=CARTESIAN_POINT('Ctrl Pts',(90.0253879613002,-22.4170872144436,10.));
#27539=CARTESIAN_POINT('Ctrl Pts',(90.0442197521512,-22.3982237163382,10.));
#27540=CARTESIAN_POINT('Ctrl Pts',(90.0633900127449,-22.3796798067826,10.));
#27541=CARTESIAN_POINT('Ctrl Pts',(90.0828885913555,-22.3614597865289,10.));
#27542=CARTESIAN_POINT('Origin',(92.,-24.,5.));
#27543=CARTESIAN_POINT('Origin',(-24.,-92.,1.));
#27544=CARTESIAN_POINT('Ctrl Pts',(-25.913465996665,-90.364012796625,0.999999999999996));
#27545=CARTESIAN_POINT('Ctrl Pts',(-25.9756062673146,-90.4224093923451,
0.999999999999996));
#27546=CARTESIAN_POINT('Ctrl Pts',(-26.034371236743,-90.4840596836494,0.999999999999993));
#27547=CARTESIAN_POINT('Ctrl Pts',(-26.089748867249,-90.5485872413642,0.999999999999997));
#27548=CARTESIAN_POINT('Ctrl Pts',(-26.1464812232126,-90.6146933629207,
1.));
#27549=CARTESIAN_POINT('Ctrl Pts',(-26.1996589497415,-90.6838197394388,
1.));
#27550=CARTESIAN_POINT('Ctrl Pts',(-26.2492402162037,-90.7556079093069,
1.));
#27551=CARTESIAN_POINT('Ctrl Pts',(-26.2621838799929,-90.77434889761,1.));
#27552=CARTESIAN_POINT('Ctrl Pts',(-26.2748822665281,-90.7932715095309,
1.));
#27553=CARTESIAN_POINT('Ctrl Pts',(-26.287334255627,-90.8123698011315,1.));
#27554=CARTESIAN_POINT('Ctrl Pts',(-26.29749533292,-90.8279543969398,1.));
#27555=CARTESIAN_POINT('Ctrl Pts',(-26.3074927699566,-90.8436568716418,
1.));
#27556=CARTESIAN_POINT('Ctrl Pts',(-26.3173171311148,-90.8594594346009,
1.));
#27557=CARTESIAN_POINT('Ctrl Pts',(-26.3647643834219,-90.9357787168166,
1.));
#27558=CARTESIAN_POINT('Ctrl Pts',(-26.4082280607616,-91.014505223999,1.00000000000001));
#27559=CARTESIAN_POINT('Ctrl Pts',(-26.4476734128481,-91.0952464686478,
1.00000000000001));
#27560=CARTESIAN_POINT('Ctrl Pts',(-26.479514252443,-91.1604219299776,1.00000000000001));
#27561=CARTESIAN_POINT('Ctrl Pts',(-26.5087362738458,-91.2269112715432,
1.));
#27562=CARTESIAN_POINT('Ctrl Pts',(-26.5353040214271,-91.2945258795828,
1.));
#27563=CARTESIAN_POINT('Ctrl Pts',(-26.5460285866473,-91.3218197731108,
1.));
#27564=CARTESIAN_POINT('Ctrl Pts',(-26.5563204553652,-91.3492971819707,
1.));
#27565=CARTESIAN_POINT('Ctrl Pts',(-26.5661765051131,-91.3769462663626,
1.));
#27566=CARTESIAN_POINT('Ctrl Pts',(-26.5713946913052,-91.391584795397,1.));
#27567=CARTESIAN_POINT('Ctrl Pts',(-26.5764901577044,-91.4062701187452,
1.00000000000001));
#27568=CARTESIAN_POINT('Ctrl Pts',(-26.5814586838643,-91.4209886610266,
1.00000000000001));
#27569=CARTESIAN_POINT('Ctrl Pts',(-26.6109727393212,-91.5084197943558,
1.00000000000001));
#27570=CARTESIAN_POINT('Ctrl Pts',(-26.6360505229659,-91.5971308115395,
1.));
#27571=CARTESIAN_POINT('Ctrl Pts',(-26.6566592692921,-91.6867240182697,
1.));
#27572=CARTESIAN_POINT('Ctrl Pts',(-26.6775869543672,-91.7777037598634,
1.));
#27573=CARTESIAN_POINT('Ctrl Pts',(-26.6939067073515,-91.8695940137173,
1.00000000000001));
#27574=CARTESIAN_POINT('Ctrl Pts',(-26.7055423733552,-91.9620114717871,
1.00000000000001));
#27575=CARTESIAN_POINT('Ctrl Pts',(-26.7170868810523,-92.0537048957565,
1.00000000000001));
#27576=CARTESIAN_POINT('Ctrl Pts',(-26.724020751965,-92.1459182254205,1.));
#27577=CARTESIAN_POINT('Ctrl Pts',(-26.7262226527309,-92.2382962505423,
1.));
#27578=CARTESIAN_POINT('Ctrl Pts',(-26.7273178683138,-92.2842446666544,
1.));
#27579=CARTESIAN_POINT('Ctrl Pts',(-26.7272416203271,-92.3302340409407,
1.));
#27580=CARTESIAN_POINT('Ctrl Pts',(-26.7259741877374,-92.3762213556111,
1.));
#27581=CARTESIAN_POINT('Ctrl Pts',(-26.7255574259114,-92.3913430728443,
1.));
#27582=CARTESIAN_POINT('Ctrl Pts',(-26.7250117562314,-92.4064664174684,
1.00000000000001));
#27583=CARTESIAN_POINT('Ctrl Pts',(-26.7243366619654,-92.4215840384697,
1.00000000000001));
#27584=CARTESIAN_POINT('Ctrl Pts',(-26.7200628111856,-92.5172898673486,
1.00000000000001));
#27585=CARTESIAN_POINT('Ctrl Pts',(-26.7106219303704,-92.6124285203872,
1.));
#27586=CARTESIAN_POINT('Ctrl Pts',(-26.6959498489085,-92.7066016678489,
1.));
#27587=CARTESIAN_POINT('Ctrl Pts',(-26.6917951398295,-92.7332687792454,
1.));
#27588=CARTESIAN_POINT('Ctrl Pts',(-26.6872206693378,-92.7598586005847,
1.00000000000001));
#27589=CARTESIAN_POINT('Ctrl Pts',(-26.682224266105,-92.7863623464052,1.));
#27590=CARTESIAN_POINT('Ctrl Pts',(-26.6652593323816,-92.8763539404211,
1.));
#27591=CARTESIAN_POINT('Ctrl Pts',(-26.6434341104625,-92.9653530573532,
1.));
#27592=CARTESIAN_POINT('Ctrl Pts',(-26.617051236812,-93.0531274604727,1.));
#27593=CARTESIAN_POINT('Ctrl Pts',(-26.5900718918307,-93.1428862916619,
1.));
#27594=CARTESIAN_POINT('Ctrl Pts',(-26.5583262747371,-93.2313651060399,
1.));
#27595=CARTESIAN_POINT('Ctrl Pts',(-26.5220837746486,-93.3183118483727,
1.));
#27596=CARTESIAN_POINT('Ctrl Pts',(-26.5094168709692,-93.3487000944288,
1.));
#27597=CARTESIAN_POINT('Ctrl Pts',(-26.496200198248,-93.3789011100651,1.00000000000001));
#27598=CARTESIAN_POINT('Ctrl Pts',(-26.4824438244401,-93.4089037784374,
1.00000000000001));
#27599=CARTESIAN_POINT('Ctrl Pts',(-26.4754968109029,-93.424055223596,1.00000000000001));
#27600=CARTESIAN_POINT('Ctrl Pts',(-26.4684121470773,-93.4391560808108,
1.00000000000001));
#27601=CARTESIAN_POINT('Ctrl Pts',(-26.4611910622915,-93.4542048926094,
1.00000000000001));
#27602=CARTESIAN_POINT('Ctrl Pts',(-26.4551808929969,-93.4667301446008,
1.00000000000001));
#27603=CARTESIAN_POINT('Ctrl Pts',(-26.4490780639285,-93.479215407299,1.00000000000001));
#27604=CARTESIAN_POINT('Ctrl Pts',(-26.4428871735715,-93.4916526560001,
1.00000000000001));
#27605=CARTESIAN_POINT('Ctrl Pts',(-26.3999238163837,-93.5779643054661,
1.00000000000001));
#27606=CARTESIAN_POINT('Ctrl Pts',(-26.3526734208407,-93.6620692716443,
0.999999999999998));
#27607=CARTESIAN_POINT('Ctrl Pts',(-26.3014780532023,-93.7437174767272,
0.999999999999999));
#27608=CARTESIAN_POINT('Ctrl Pts',(-26.2492778937103,-93.8269681598294,
1.));
#27609=CARTESIAN_POINT('Ctrl Pts',(-26.1929760723445,-93.9076654736707,
1.));
#27610=CARTESIAN_POINT('Ctrl Pts',(-26.1328802773408,-93.9855370025748,
1.));
#27611=CARTESIAN_POINT('Ctrl Pts',(-26.0723164767454,-94.0640149684343,
1.));
#27612=CARTESIAN_POINT('Ctrl Pts',(-26.0078989173972,-94.1396238025829,
1.));
#27613=CARTESIAN_POINT('Ctrl Pts',(-25.9398933828955,-94.2120650883093,
1.));
#27614=CARTESIAN_POINT('Ctrl Pts',(-25.9029668417263,-94.2514002121243,
1.));
#27615=CARTESIAN_POINT('Ctrl Pts',(-25.8649816080713,-94.2898009986756,
1.));
#27616=CARTESIAN_POINT('Ctrl Pts',(-25.8259749927721,-94.3272159154238,
1.));
#27617=CARTESIAN_POINT('Ctrl Pts',(-25.8138410599859,-94.3388547126263,
1.));
#27618=CARTESIAN_POINT('Ctrl Pts',(-25.8016082666696,-94.3503980875446,
1.));
#27619=CARTESIAN_POINT('Ctrl Pts',(-25.7892776711008,-94.3618444242613,
1.));
#27620=CARTESIAN_POINT('Ctrl Pts',(-25.7779940533511,-94.3723188646422,
1.));
#27621=CARTESIAN_POINT('Ctrl Pts',(-25.7666342742199,-94.382706679586,0.999999999999998));
#27622=CARTESIAN_POINT('Ctrl Pts',(-25.7552037476042,-94.3930030340632,
0.999999999999998));
#27623=CARTESIAN_POINT('Ctrl Pts',(-25.6793946851099,-94.4612900873433,
0.999999999999999));
#27624=CARTESIAN_POINT('Ctrl Pts',(-25.6004193338813,-94.5256101174112,
1.));
#27625=CARTESIAN_POINT('Ctrl Pts',(-25.5186038566385,-94.585680500128,1.));
#27626=CARTESIAN_POINT('Ctrl Pts',(-25.4367174576773,-94.6458029548355,
1.));
#27627=CARTESIAN_POINT('Ctrl Pts',(-25.351985429782,-94.7016692285508,1.));
#27628=CARTESIAN_POINT('Ctrl Pts',(-25.2646898214108,-94.7529697581317,
1.));
#27629=CARTESIAN_POINT('Ctrl Pts',(-25.1791579833755,-94.8032337825095,
0.999999999999999));
#27630=CARTESIAN_POINT('Ctrl Pts',(-25.0911644460643,-94.8491153707221,
1.));
#27631=CARTESIAN_POINT('Ctrl Pts',(-25.0009407551715,-94.8902872128736,
1.00000000000001));
#27632=CARTESIAN_POINT('Ctrl Pts',(-24.9631517387227,-94.9075315020941,
1.00000000000001));
#27633=CARTESIAN_POINT('Ctrl Pts',(-24.9249711429332,-94.923949087781,1.));
#27634=CARTESIAN_POINT('Ctrl Pts',(-24.8864145873395,-94.9395135460182,
1.));
#27635=CARTESIAN_POINT('Ctrl Pts',(-24.8564008951788,-94.9516294326939,
1.));
#27636=CARTESIAN_POINT('Ctrl Pts',(-24.8261593691065,-94.9632283272653,
1.));
#27637=CARTESIAN_POINT('Ctrl Pts',(-24.7957017813267,-94.9743128096467,
1.));
#27638=CARTESIAN_POINT('Ctrl Pts',(-23.2062007174672,-94.9692229537457,
0.999999999999999));
#27639=CARTESIAN_POINT('Ctrl Pts',(-23.1113643951015,-94.9345314033933,
0.999999999999999));
#27640=CARTESIAN_POINT('Ctrl Pts',(-23.0185713035646,-94.8948494397886,
0.999999999999999));
#27641=CARTESIAN_POINT('Ctrl Pts',(-22.9280623762531,-94.8504973089186,
1.));
#27642=CARTESIAN_POINT('Ctrl Pts',(-22.8362819518079,-94.8055221057291,
1.));
#27643=CARTESIAN_POINT('Ctrl Pts',(-22.7468496512481,-94.7557438960029,
1.));
#27644=CARTESIAN_POINT('Ctrl Pts',(-22.6600507311628,-94.7014559325677,
1.));
#27645=CARTESIAN_POINT('Ctrl Pts',(-22.6355419727356,-94.6861270485212,
1.));
#27646=CARTESIAN_POINT('Ctrl Pts',(-22.6112434098515,-94.67043839863,1.));
#27647=CARTESIAN_POINT('Ctrl Pts',(-22.587162060266,-94.6543961292366,1.));
#27648=CARTESIAN_POINT('Ctrl Pts',(-22.5678313680127,-94.641518604595,1.));
#27649=CARTESIAN_POINT('Ctrl Pts',(-22.5486385356581,-94.6284115926912,
1.));
#27650=CARTESIAN_POINT('Ctrl Pts',(-22.5296064818783,-94.6150920387402,
1.));
#27651=CARTESIAN_POINT('Ctrl Pts',(-22.4468988465926,-94.5572092257188,
1.));
#27652=CARTESIAN_POINT('Ctrl Pts',(-22.3671460458253,-94.4952646292979,
1.));
#27653=CARTESIAN_POINT('Ctrl Pts',(-22.2906144353731,-94.4295554855911,
1.));
#27654=CARTESIAN_POINT('Ctrl Pts',(-22.2316015869558,-94.3788877456299,
1.));
#27655=CARTESIAN_POINT('Ctrl Pts',(-22.174504633498,-94.3259807640076,1.));
#27656=CARTESIAN_POINT('Ctrl Pts',(-22.1194632793834,-94.270959034197,1.));
#27657=CARTESIAN_POINT('Ctrl Pts',(-22.0901431561929,-94.2416493647283,
1.));
#27658=CARTESIAN_POINT('Ctrl Pts',(-22.0614066098028,-94.2117394621323,
1.));
#27659=CARTESIAN_POINT('Ctrl Pts',(-22.0332767871003,-94.181247310107,1.));
#27660=CARTESIAN_POINT('Ctrl Pts',(-22.0236428018515,-94.1708042672935,
1.));
#27661=CARTESIAN_POINT('Ctrl Pts',(-22.014080781236,-94.1602937100153,1.));
#27662=CARTESIAN_POINT('Ctrl Pts',(-22.0045982120006,-94.1497238888402,
1.));
#27663=CARTESIAN_POINT('Ctrl Pts',(-21.9388057221636,-94.0763877670595,
1.));
#27664=CARTESIAN_POINT('Ctrl Pts',(-21.8767454820535,-94.0001052969862,
0.999999999999998));
#27665=CARTESIAN_POINT('Ctrl Pts',(-21.8186612829854,-93.9211548960136,
0.999999999999999));
#27666=CARTESIAN_POINT('Ctrl Pts',(-21.7610834895644,-93.8428928221512,
0.999999999999999));
#27667=CARTESIAN_POINT('Ctrl Pts',(-21.7074122723325,-93.7620083511859,
0.999999999999998));
#27668=CARTESIAN_POINT('Ctrl Pts',(-21.6579309059598,-93.6787502765599,
0.999999999999997));
#27669=CARTESIAN_POINT('Ctrl Pts',(-21.609882526023,-93.5979033659812,0.999999999999997));
#27670=CARTESIAN_POINT('Ctrl Pts',(-21.5657846284247,-93.5148176409593,
1.));
#27671=CARTESIAN_POINT('Ctrl Pts',(-21.5259443770376,-93.4297105806012,
1.));
#27672=CARTESIAN_POINT('Ctrl Pts',(-21.5051331098544,-93.3852533869181,
1.));
#27673=CARTESIAN_POINT('Ctrl Pts',(-21.4854844375003,-93.3402445256234,
1.));
#27674=CARTESIAN_POINT('Ctrl Pts',(-21.4670478470219,-93.2947147599259,
1.));
#27675=CARTESIAN_POINT('Ctrl Pts',(-21.4599071766554,-93.2770806399357,
1.));
#27676=CARTESIAN_POINT('Ctrl Pts',(-21.452948372869,-93.259368380918,1.));
#27677=CARTESIAN_POINT('Ctrl Pts',(-21.4461744794312,-93.2415797793335,
1.));
#27678=CARTESIAN_POINT('Ctrl Pts',(-21.44102059279,-93.2280454010747,1.));
#27679=CARTESIAN_POINT('Ctrl Pts',(-21.4359737887531,-93.2144667091695,
1.));
#27680=CARTESIAN_POINT('Ctrl Pts',(-21.4310402382862,-93.2008583988899,
1.));
#27681=CARTESIAN_POINT('Ctrl Pts',(-21.3993683884323,-93.1134973061374,
1.));
#27682=CARTESIAN_POINT('Ctrl Pts',(-21.3723052492582,-93.0247752793144,
1.00000000000001));
#27683=CARTESIAN_POINT('Ctrl Pts',(-21.3501021064032,-92.9349157240161,
1.));
#27684=CARTESIAN_POINT('Ctrl Pts',(-21.3450995091274,-92.9146694386377,
1.));
#27685=CARTESIAN_POINT('Ctrl Pts',(-21.3403438331481,-92.8943653670041,
1.));
#27686=CARTESIAN_POINT('Ctrl Pts',(-21.3358383183128,-92.8740060081578,
1.));
#27687=CARTESIAN_POINT('Ctrl Pts',(-21.3154927915296,-92.7820693714265,
1.));
#27688=CARTESIAN_POINT('Ctrl Pts',(-21.300244266593,-92.6890050257244,1.));
#27689=CARTESIAN_POINT('Ctrl Pts',(-21.2899828336258,-92.5952047143721,
1.));
#27690=CARTESIAN_POINT('Ctrl Pts',(-21.2792696952259,-92.4972753393334,
1.));
#27691=CARTESIAN_POINT('Ctrl Pts',(-21.2739923846859,-92.3985425391084,
1.));
#27692=CARTESIAN_POINT('Ctrl Pts',(-21.2740833202269,-92.2994667952251,
1.));
#27693=CARTESIAN_POINT('Ctrl Pts',(-21.2741184401282,-92.2612030942814,
1.));
#27694=CARTESIAN_POINT('Ctrl Pts',(-21.2749548502656,-92.2228884941123,
0.999999999999998));
#27695=CARTESIAN_POINT('Ctrl Pts',(-21.2765907919834,-92.1845506992199,
0.999999999999998));
#27696=CARTESIAN_POINT('Ctrl Pts',(-21.2771783957654,-92.1707803839174,
0.999999999999998));
#27697=CARTESIAN_POINT('Ctrl Pts',(-21.2778691417354,-92.1570088742633,
1.));
#27698=CARTESIAN_POINT('Ctrl Pts',(-21.2786620583866,-92.1432491225241,
1.));
#27699=CARTESIAN_POINT('Ctrl Pts',(-21.2840136676365,-92.050380831051,1.));
#27700=CARTESIAN_POINT('Ctrl Pts',(-21.2940209875981,-91.9578996301337,
1.));
#27701=CARTESIAN_POINT('Ctrl Pts',(-21.3085609609126,-91.8661774191351,
1.));
#27702=CARTESIAN_POINT('Ctrl Pts',(-21.3230638860674,-91.7746889182712,
1.));
#27703=CARTESIAN_POINT('Ctrl Pts',(-21.3420768068504,-91.6839546001225,
0.999999999999999));
#27704=CARTESIAN_POINT('Ctrl Pts',(-21.3655261933471,-91.5943606400854,
1.));
#27705=CARTESIAN_POINT('Ctrl Pts',(-21.3885742799942,-91.506299941598,1.));
#27706=CARTESIAN_POINT('Ctrl Pts',(-21.4159087531981,-91.4193401209881,
0.999999999999999));
#27707=CARTESIAN_POINT('Ctrl Pts',(-21.4475001288737,-91.3338770867914,
0.999999999999999));
#27708=CARTESIAN_POINT('Ctrl Pts',(-21.463362608245,-91.2909648809136,0.999999999999999));
#27709=CARTESIAN_POINT('Ctrl Pts',(-21.480298928196,-91.248430578413,1.));
#27710=CARTESIAN_POINT('Ctrl Pts',(-21.498308744999,-91.2063280780076,1.));
#27711=CARTESIAN_POINT('Ctrl Pts',(-21.5036080596924,-91.1939395900253,
1.));
#27712=CARTESIAN_POINT('Ctrl Pts',(-21.5090003324731,-91.1815885066313,
0.999999999999998));
#27713=CARTESIAN_POINT('Ctrl Pts',(-21.5144855890668,-91.169276249741,0.999999999999998));
#27714=CARTESIAN_POINT('Ctrl Pts',(-21.5200790128479,-91.156721199797,0.999999999999998));
#27715=CARTESIAN_POINT('Ctrl Pts',(-21.5257654437118,-91.1442148112825,
0.999999999999997));
#27716=CARTESIAN_POINT('Ctrl Pts',(-21.5315435926219,-91.1317604192609,
0.999999999999997));
#27717=CARTESIAN_POINT('Ctrl Pts',(-21.5690289713544,-91.0509633319802,
0.999999999999998));
#27718=CARTESIAN_POINT('Ctrl Pts',(-21.6103840526462,-90.9723231042384,
0.999999999999998));
#27719=CARTESIAN_POINT('Ctrl Pts',(-21.6555390130635,-90.8961874418052,
0.999999999999998));
#27720=CARTESIAN_POINT('Ctrl Pts',(-21.6999357871794,-90.8213301553416,
0.999999999999998));
#27721=CARTESIAN_POINT('Ctrl Pts',(-21.7480063603779,-90.7488933636716,
0.999999999999999));
#27722=CARTESIAN_POINT('Ctrl Pts',(-21.7997205682537,-90.6792417325679,
0.999999999999999));
#27723=CARTESIAN_POINT('Ctrl Pts',(-21.8498548287834,-90.6117180642475,
1.));
#27724=CARTESIAN_POINT('Ctrl Pts',(-21.9034139309536,-90.5468115335925,
1.));
#27725=CARTESIAN_POINT('Ctrl Pts',(-21.9603980831221,-90.4848946771838,
1.));
#27726=CARTESIAN_POINT('Ctrl Pts',(-21.98158716959,-90.4618714053732,1.));
#27727=CARTESIAN_POINT('Ctrl Pts',(-22.0032500736797,-90.4392619466834,
1.));
#27728=CARTESIAN_POINT('Ctrl Pts',(-22.0253876448586,-90.417087121357,1.));
#27729=CARTESIAN_POINT('Ctrl Pts',(-22.0442144350809,-90.3982286485253,
1.));
#27730=CARTESIAN_POINT('Ctrl Pts',(-22.0633845524044,-90.3796845518288,
0.999999999999999));
#27731=CARTESIAN_POINT('Ctrl Pts',(-22.0828882653786,-90.3614597476137,
0.999999999999999));
#27732=CARTESIAN_POINT('Origin',(-24.,-92.,12.2084234471775));
#27733=CARTESIAN_POINT('Ctrl Pts',(-27.0767669904684,-91.998062685181,9.70842344717746));
#27734=CARTESIAN_POINT('Ctrl Pts',(-27.0777011675186,-91.8738981078455,
9.70197366100994));
#27735=CARTESIAN_POINT('Ctrl Pts',(-27.0146668802256,-90.7368860788636,
9.64286281975954));
#27736=CARTESIAN_POINT('Ctrl Pts',(-25.5990318095031,-88.7444872358932,
9.53109092342626));
#27737=CARTESIAN_POINT('Ctrl Pts',(-22.1476049582095,-88.8820466605266,
9.37310775817762));
#27738=CARTESIAN_POINT('Ctrl Pts',(-20.3764280027803,-91.847285042836,9.21512459292899));
#27739=CARTESIAN_POINT('Ctrl Pts',(-21.8919230124438,-94.9512424150719,
9.05714142768036));
#27740=CARTESIAN_POINT('Ctrl Pts',(-25.3195312348388,-95.3782236147545,
8.89915826243172));
#27741=CARTESIAN_POINT('Ctrl Pts',(-26.9608441448919,-93.4378981546875,
8.78291893559742));
#27742=CARTESIAN_POINT('Ctrl Pts',(-27.0762794797313,-92.213313773738,8.719340663846));
#27743=CARTESIAN_POINT('Ctrl Pts',(-27.0743676381347,-92.0026790873961,
8.70842344717746));
#27744=CARTESIAN_POINT('Ctrl Pts',(-27.0702887490762,-92.0031018432153,
9.79157655282255));
#27745=CARTESIAN_POINT('Ctrl Pts',(-27.0652853033504,-91.3096184359041,
9.75572892504928));
#27746=CARTESIAN_POINT('Ctrl Pts',(-26.4922441588307,-89.5876431146109,
9.66722024219313));
#27747=CARTESIAN_POINT('Ctrl Pts',(-23.6460838755241,-88.3911593875009,
9.52605050425409));
#27748=CARTESIAN_POINT('Ctrl Pts',(-20.7843953448966,-90.3229252160129,
9.36806733900547));
#27749=CARTESIAN_POINT('Ctrl Pts',(-20.8381771631847,-93.7771164103054,
9.21008417375682));
#27750=CARTESIAN_POINT('Ctrl Pts',(-23.7604241627304,-95.6187849549087,
9.05210100850819));
#27751=CARTESIAN_POINT('Ctrl Pts',(-26.5324624275929,-94.346888962543,8.91259846819677));
#27752=CARTESIAN_POINT('Ctrl Pts',(-27.0660798384141,-92.6595176403423,
8.82575698296822));
#27753=CARTESIAN_POINT('Ctrl Pts',(-27.0703859251749,-91.9978642356407,
8.79157655282255));
#27754=CARTESIAN_POINT('Ctrl Pts',(-22.0865340033349,-90.364012796625,10.));
#27755=CARTESIAN_POINT('Ctrl Pts',(-21.5452199193478,-90.9971388327508,
9.94733894491712));
#27756=CARTESIAN_POINT('Ctrl Pts',(-21.1498731367063,-92.8326003723509,
9.84201683475137));
#27757=CARTESIAN_POINT('Ctrl Pts',(-23.1420127726733,-94.8458067969654,
9.68403366950273));
#27758=CARTESIAN_POINT('Ctrl Pts',(-25.9132999553889,-94.2718355849706,
9.5260505042541));
#27759=CARTESIAN_POINT('Ctrl Pts',(-26.948715185934,-91.6401115468636,9.36806733900547));
#27760=CARTESIAN_POINT('Ctrl Pts',(-25.3097649521471,-89.3334135729173,
9.21008417375683));
#27761=CARTESIAN_POINT('Ctrl Pts',(-22.4827055416601,-89.4460883253215,
9.05210100850819));
#27762=CARTESIAN_POINT('Ctrl Pts',(-21.0319367161215,-91.8749113698844,
8.89411784325956));
#27763=CARTESIAN_POINT('Ctrl Pts',(-22.2732767801618,-94.4173589653306,
8.73613467801093));
#27764=CARTESIAN_POINT('Ctrl Pts',(-25.0808263815541,-94.7670987311353,
8.57815151276229));
#27765=CARTESIAN_POINT('Ctrl Pts',(-26.9080233748187,-92.6070250335036,
8.42016834751366));
#27766=CARTESIAN_POINT('Ctrl Pts',(-26.0975469404961,-89.8963395546467,
8.26218518226502));
#27767=CARTESIAN_POINT('Ctrl Pts',(-23.384522353545,-89.0937553800026,8.10420201701639));
#27768=CARTESIAN_POINT('Ctrl Pts',(-21.2297577260391,-90.9272296313332,
7.94621885176776));
#27769=CARTESIAN_POINT('Ctrl Pts',(-21.5876970395809,-93.733745495277,7.78823568651912));
#27770=CARTESIAN_POINT('Ctrl Pts',(-24.1336776494793,-94.9676939059565,
7.63025252127048));
#27771=CARTESIAN_POINT('Ctrl Pts',(-26.5584079833072,-93.5098431949504,
7.47226935602185));
#27772=CARTESIAN_POINT('Ctrl Pts',(-26.662574994087,-90.6825129051978,7.31428619077321));
#27773=CARTESIAN_POINT('Ctrl Pts',(-24.3516955853902,-89.0501885096969,
7.15630302552458));
#27774=CARTESIAN_POINT('Ctrl Pts',(-21.7218162866321,-90.0934437553397,
6.99831986027595));
#27775=CARTESIAN_POINT('Ctrl Pts',(-21.1583273702903,-92.8660106210542,
6.84033669502731));
#27776=CARTESIAN_POINT('Ctrl Pts',(-23.1723325238739,-94.8530762793412,
6.68235352977868));
#27777=CARTESIAN_POINT('Ctrl Pts',(-25.9370603271938,-94.2523043781638,
6.52437036453004));
#27778=CARTESIAN_POINT('Ctrl Pts',(-26.944808298303,-91.6086155263393,6.36638719928141));
#27779=CARTESIAN_POINT('Ctrl Pts',(-25.2815146299499,-89.3199257527161,
6.20840403403277));
#27780=CARTESIAN_POINT('Ctrl Pts',(-22.4558434515285,-89.4621547971772,
6.05042086878414));
#27781=CARTESIAN_POINT('Ctrl Pts',(-21.0307749678768,-91.9062960631275,
5.8924377035355));
#27782=CARTESIAN_POINT('Ctrl Pts',(-22.2988949344083,-94.4354299979253,
5.73445453828687));
#27783=CARTESIAN_POINT('Ctrl Pts',(-25.1099752577798,-94.7555457982637,
5.57647137303824));
#27784=CARTESIAN_POINT('Ctrl Pts',(-26.9142701365138,-92.576287506837,5.4184882077896));
#27785=CARTESIAN_POINT('Ctrl Pts',(-26.0752225311475,-89.8743167768149,
5.26050504254097));
#27786=CARTESIAN_POINT('Ctrl Pts',(-23.3538772582214,-89.1004132843165,
5.10252187729234));
#27787=CARTESIAN_POINT('Ctrl Pts',(-21.2185873656771,-90.9565339120964,
4.94453871204369));
#27788=CARTESIAN_POINT('Ctrl Pts',(-21.6061336679678,-93.7591138972605,
4.78655554679507));
#27789=CARTESIAN_POINT('Ctrl Pts',(-24.1649984413479,-94.9661175354377,
4.62857238154642));
#27790=CARTESIAN_POINT('Ctrl Pts',(-26.574203996375,-93.4827513287052,4.4705892162978));
#27791=CARTESIAN_POINT('Ctrl Pts',(-26.6485186642022,-90.6544790580041,
4.31260605104916));
#27792=CARTESIAN_POINT('Ctrl Pts',(-24.3205365027268,-89.0466402058835,
4.15462288580052));
#27793=CARTESIAN_POINT('Ctrl Pts',(-21.7018167952366,-90.1175994942308,
3.99663972055189));
#27794=CARTESIAN_POINT('Ctrl Pts',(-21.1676276911652,-92.8959602861542,
3.83865655530326));
#27795=CARTESIAN_POINT('Ctrl Pts',(-23.2024969568081,-94.8616545287659,
3.68067339005462));
#27796=CARTESIAN_POINT('Ctrl Pts',(-25.9607286813379,-94.2317304163557,
3.52269022480599));
#27797=CARTESIAN_POINT('Ctrl Pts',(-26.9405126124961,-91.5775506895979,
3.36470705955735));
#27798=CARTESIAN_POINT('Ctrl Pts',(-25.2531511472893,-89.3065468104243,
3.20672389430872));
#27799=CARTESIAN_POINT('Ctrl Pts',(-22.4291390042644,-89.4785971036944,
3.04874072906008));
#27800=CARTESIAN_POINT('Ctrl Pts',(-21.0299510223576,-91.937645484163,2.89075756381145));
#27801=CARTESIAN_POINT('Ctrl Pts',(-22.3246996110788,-94.453252357017,2.73277439856282));
#27802=CARTESIAN_POINT('Ctrl Pts',(-25.1390012538636,-94.7436739362117,
2.57479123331418));
#27803=CARTESIAN_POINT('Ctrl Pts',(-26.9201931102794,-92.5454930206752,
2.41680806806555));
#27804=CARTESIAN_POINT('Ctrl Pts',(-26.0526635517577,-89.8525243463365,
2.25882490281691));
#27805=CARTESIAN_POINT('Ctrl Pts',(-23.3233115518592,-89.1074036232017,
2.10084173756828));
#27806=CARTESIAN_POINT('Ctrl Pts',(-21.2077115778015,-90.9859374711348,
1.94285857231964));
#27807=CARTESIAN_POINT('Ctrl Pts',(-21.624868659881,-93.7843200216542,1.78487540707101));
#27808=CARTESIAN_POINT('Ctrl Pts',(-24.1962362586587,-94.964142143379,1.62689224182237));
#27809=CARTESIAN_POINT('Ctrl Pts',(-26.5898450807175,-93.4556338347463,
1.46890907657374));
#27810=CARTESIAN_POINT('Ctrl Pts',(-26.6338976845917,-90.6263101028394,
1.3109259113251));
#27811=CARTESIAN_POINT('Ctrl Pts',(-24.2898922478439,-89.0440033611201,
1.15294274607647));
#27812=CARTESIAN_POINT('Ctrl Pts',(-21.6809479657765,-90.1407646543606,
0.994959580827837));
#27813=CARTESIAN_POINT('Ctrl Pts',(-21.1795854924137,-92.928282565981,0.836976415579201));
#27814=CARTESIAN_POINT('Ctrl Pts',(-22.5450731455404,-94.2169491679593,
0.731654305413445));
#27815=CARTESIAN_POINT('Ctrl Pts',(-23.3498000020249,-94.4320868020351,
0.678993250330566));
#27816=CARTESIAN_POINT('Ctrl Pts',(-21.9456684496579,-90.2435746787731,
10.1070022498898));
#27817=CARTESIAN_POINT('Ctrl Pts',(-21.3645039014938,-90.9233101920371,
10.0543411948069));
#27818=CARTESIAN_POINT('Ctrl Pts',(-20.9400524765287,-92.8938947526259,
9.94901908464118));
#27819=CARTESIAN_POINT('Ctrl Pts',(-23.0788494627237,-95.0553094224687,
9.79103591939254));
#27820=CARTESIAN_POINT('Ctrl Pts',(-26.0541532854381,-94.4390835936093,
9.63305275414391));
#27821=CARTESIAN_POINT('Ctrl Pts',(-27.1657937219656,-91.6136172760999,
9.47506958889528));
#27822=CARTESIAN_POINT('Ctrl Pts',(-25.4061872379324,-89.1371047939092,
9.31708642364664));
#27823=CARTESIAN_POINT('Ctrl Pts',(-22.3710053471766,-89.2580744370565,
9.159103258398));
#27824=CARTESIAN_POINT('Ctrl Pts',(-20.8134338116745,-91.8657025942017,
9.00112009314937));
#27825=CARTESIAN_POINT('Ctrl Pts',(-22.1461588575891,-94.5953201152443,
8.84313692790073));
#27826=CARTESIAN_POINT('Ctrl Pts',(-25.1603946659823,-94.9708070256751,
8.68515376265211));
#27827=CARTESIAN_POINT('Ctrl Pts',(-27.1221062608033,-92.6517130068406,
8.52717059740346));
#27828=CARTESIAN_POINT('Ctrl Pts',(-26.2519641664366,-89.741472264661,8.36918743215484));
#27829=CARTESIAN_POINT('Ctrl Pts',(-23.3392121156861,-88.8798034424032,
8.21120426690619));
#27830=CARTESIAN_POINT('Ctrl Pts',(-21.0258180101408,-90.8482544145204,
8.05322110165756));
#27831=CARTESIAN_POINT('Ctrl Pts',(-21.4101081026736,-93.861380383774,7.89523793640894));
#27832=CARTESIAN_POINT('Ctrl Pts',(-24.1435187316522,-95.186169617537,7.73725477116029));
#27833=CARTESIAN_POINT('Ctrl Pts',(-26.7467528808536,-93.6209948422715,
7.57927160591167));
#27834=CARTESIAN_POINT('Ctrl Pts',(-26.8585884593915,-90.5855221306583,
7.42128844066302));
#27835=CARTESIAN_POINT('Ctrl Pts',(-24.3775867135566,-88.8330292659221,
7.26330527541439));
#27836=CARTESIAN_POINT('Ctrl Pts',(-21.5541009414308,-89.9530868838363,
7.10532211016575));
#27837=CARTESIAN_POINT('Ctrl Pts',(-20.9491290939422,-92.9297645972614,
6.94733894491712));
#27838=CARTESIAN_POINT('Ctrl Pts',(-23.111401293589,-95.0631140696508,6.78935577966849));
#27839=CARTESIAN_POINT('Ctrl Pts',(-26.0796628484675,-94.4181145382775,
6.63137261441986));
#27840=CARTESIAN_POINT('Ctrl Pts',(-27.1615992170526,-91.579802581307,6.47338944917121));
#27841=CARTESIAN_POINT('Ctrl Pts',(-25.37585718331,-89.1226240272624,6.31540628392259));
#27842=CARTESIAN_POINT('Ctrl Pts',(-22.342165723498,-89.2753236905542,6.15742311867395));
#27843=CARTESIAN_POINT('Ctrl Pts',(-20.812186537839,-91.8993977660205,5.99943995342531));
#27844=CARTESIAN_POINT('Ctrl Pts',(-22.1736629693016,-94.6147215012481,
5.84145678817668));
#27845=CARTESIAN_POINT('Ctrl Pts',(-25.1916894243902,-94.9584035889072,
5.68347362292805));
#27846=CARTESIAN_POINT('Ctrl Pts',(-27.1288128966464,-92.618712644712,5.52549045767941));
#27847=CARTESIAN_POINT('Ctrl Pts',(-26.227996278558,-89.7178282138104,5.36750729243077));
#27848=CARTESIAN_POINT('Ctrl Pts',(-23.3063109895119,-88.8869514883655,
5.20952412718215));
#27849=CARTESIAN_POINT('Ctrl Pts',(-21.0138253101083,-90.8797160180383,
5.05154096193351));
#27850=CARTESIAN_POINT('Ctrl Pts',(-21.4299019989033,-93.8886163569595,
4.89355779668488));
#27851=CARTESIAN_POINT('Ctrl Pts',(-24.1771452978046,-95.1844771977619,
4.73557463143624));
#27852=CARTESIAN_POINT('Ctrl Pts',(-26.7637117649264,-93.5919085268197,
4.5775914661876));
#27853=CARTESIAN_POINT('Ctrl Pts',(-26.8434973305109,-90.5554244874977,
4.41960830093897));
#27854=CARTESIAN_POINT('Ctrl Pts',(-24.3441337613188,-88.8292197430528,
4.26162513569033));
#27855=CARTESIAN_POINT('Ctrl Pts',(-21.5326291273322,-89.9790209200889,
4.10364197044171));
#27856=CARTESIAN_POINT('Ctrl Pts',(-20.9591140859071,-92.9619190970249,
3.94565880519306));
#27857=CARTESIAN_POINT('Ctrl Pts',(-23.1437863719668,-95.0723238327043,
3.78767563994443));
#27858=CARTESIAN_POINT('Ctrl Pts',(-26.1050736196794,-94.3960259623991,
3.6296924746958));
#27859=CARTESIAN_POINT('Ctrl Pts',(-27.1569872914167,-91.5464508131884,
3.47170930944716));
#27860=CARTESIAN_POINT('Ctrl Pts',(-25.3454056375763,-89.1082601538994,
3.31372614419853));
#27861=CARTESIAN_POINT('Ctrl Pts',(-22.3134953480408,-89.2929764469124,
3.15574297894989));
#27862=CARTESIAN_POINT('Ctrl Pts',(-20.8113019350926,-91.9330550689619,
2.99775981370126));
#27863=CARTESIAN_POINT('Ctrl Pts',(-22.2013673348471,-94.6338559069014,
2.83977664845262));
#27864=CARTESIAN_POINT('Ctrl Pts',(-25.2228522564652,-94.9456577440281,
2.68179348320399));
#27865=CARTESIAN_POINT('Ctrl Pts',(-27.1351719079378,-92.5856511298438,
2.52381031795535));
#27866=CARTESIAN_POINT('Ctrl Pts',(-26.2037765520592,-89.6944314680265,
2.36582715270672));
#27867=CARTESIAN_POINT('Ctrl Pts',(-23.2734950967561,-88.8944564420696,
2.20784398745809));
#27868=CARTESIAN_POINT('Ctrl Pts',(-21.0021488684016,-90.9112842085001,
2.04986082220945));
#27869=CARTESIAN_POINT('Ctrl Pts',(-21.4500162235876,-93.9156781060024,
1.89187765696082));
#27870=CARTESIAN_POINT('Ctrl Pts',(-24.2106827809777,-95.1823563812763,
1.73389449171218));
#27871=CARTESIAN_POINT('Ctrl Pts',(-26.78050431473,-93.562794696993,1.57591132646355));
#27872=CARTESIAN_POINT('Ctrl Pts',(-26.827799983517,-90.5251817899866,1.41792816121491));
#27873=CARTESIAN_POINT('Ctrl Pts',(-24.3112335374568,-88.8263887790323,
1.25994499596628));
#27874=CARTESIAN_POINT('Ctrl Pts',(-21.5102239762329,-90.0038914531458,
1.10196183071765));
#27875=CARTESIAN_POINT('Ctrl Pts',(-20.9719521966549,-92.9966208786834,
0.943978665469012));
#27876=CARTESIAN_POINT('Ctrl Pts',(-22.4379643297735,-94.3801565479507,
0.838656555303256));
#27877=CARTESIAN_POINT('Ctrl Pts',(-23.301933573839,-94.6111321859386,0.785995500220377));
#27878=CARTESIAN_POINT('Ctrl Pts',(-21.8048028959809,-90.1231365609213,
10.2140044997796));
#27879=CARTESIAN_POINT('Ctrl Pts',(-21.1837878836397,-90.8494815513233,
10.1613434446967));
#27880=CARTESIAN_POINT('Ctrl Pts',(-20.730231816351,-92.9551891329009,10.056021334531));
#27881=CARTESIAN_POINT('Ctrl Pts',(-23.0156861527743,-95.2648120479719,
9.89803816928236));
#27882=CARTESIAN_POINT('Ctrl Pts',(-26.1950066154872,-94.606331602248,9.74005500403371));
#27883=CARTESIAN_POINT('Ctrl Pts',(-27.3828722579974,-91.5871230053361,
9.58207183878509));
#27884=CARTESIAN_POINT('Ctrl Pts',(-25.5026095237177,-88.9407960149012,
9.42408867353644));
#27885=CARTESIAN_POINT('Ctrl Pts',(-22.2593051526931,-89.0700605487915,
9.26610550828782));
#27886=CARTESIAN_POINT('Ctrl Pts',(-20.5949309072274,-91.8564938185189,
9.10812234303918));
#27887=CARTESIAN_POINT('Ctrl Pts',(-22.0190409350165,-94.7732812651581,
8.95013917779055));
#27888=CARTESIAN_POINT('Ctrl Pts',(-25.2399629504105,-95.1745153202148,
8.79215601254192));
#27889=CARTESIAN_POINT('Ctrl Pts',(-27.336189146788,-92.6964009801777,8.63417284729328));
#27890=CARTESIAN_POINT('Ctrl Pts',(-26.4063813923771,-89.5866049746754,
8.47618968204465));
#27891=CARTESIAN_POINT('Ctrl Pts',(-23.2939018778273,-88.6658515048039,
8.31820651679601));
#27892=CARTESIAN_POINT('Ctrl Pts',(-20.8218782942425,-90.7692791977077,
8.16022335154738));
#27893=CARTESIAN_POINT('Ctrl Pts',(-21.2325191657662,-93.9890152722711,
8.00224018629874));
#27894=CARTESIAN_POINT('Ctrl Pts',(-24.153359813825,-95.4046453291174,7.8442570210501));
#27895=CARTESIAN_POINT('Ctrl Pts',(-26.9350977783999,-93.7321464895926,
7.68627385580147));
#27896=CARTESIAN_POINT('Ctrl Pts',(-27.0546019246961,-90.4885313561186,
7.52829069055284));
#27897=CARTESIAN_POINT('Ctrl Pts',(-24.403477841723,-88.6158700221475,7.3703075253042));
#27898=CARTESIAN_POINT('Ctrl Pts',(-21.3863855962296,-89.8127300123325,
7.21232436005556));
#27899=CARTESIAN_POINT('Ctrl Pts',(-20.7399308175942,-92.9935185734688,
7.05434119480694));
#27900=CARTESIAN_POINT('Ctrl Pts',(-23.0504700633042,-95.2731518599606,
6.89635802955829));
#27901=CARTESIAN_POINT('Ctrl Pts',(-26.2222653697413,-94.5839246983912,
6.73837486430967));
#27902=CARTESIAN_POINT('Ctrl Pts',(-27.3783901358023,-91.550989636275,6.58039169906103));
#27903=CARTESIAN_POINT('Ctrl Pts',(-25.4701997366701,-88.9253223018084,
6.4224085338124));
#27904=CARTESIAN_POINT('Ctrl Pts',(-22.2284879954675,-89.0884925839314,
6.26442536856376));
#27905=CARTESIAN_POINT('Ctrl Pts',(-20.5935981078012,-91.8924994689134,
6.10644220331513));
#27906=CARTESIAN_POINT('Ctrl Pts',(-22.0484310041947,-94.794013004571,5.94845903806649));
#27907=CARTESIAN_POINT('Ctrl Pts',(-25.2734035910007,-95.1612613795506,
5.79047587281786));
#27908=CARTESIAN_POINT('Ctrl Pts',(-27.343355656779,-92.6611377825871,5.63249270756922));
#27909=CARTESIAN_POINT('Ctrl Pts',(-26.3807700259685,-89.561339650806,5.47450954232059));
#27910=CARTESIAN_POINT('Ctrl Pts',(-23.2587447208024,-88.6734896924145,
5.31652637707195));
#27911=CARTESIAN_POINT('Ctrl Pts',(-20.8090632545395,-90.80289812398,5.15854321182332));
#27912=CARTESIAN_POINT('Ctrl Pts',(-21.2536703298387,-94.0181188166586,
5.00056004657469));
#27913=CARTESIAN_POINT('Ctrl Pts',(-24.1892921542613,-95.4028368600861,
4.84257688132605));
#27914=CARTESIAN_POINT('Ctrl Pts',(-26.9532195334778,-93.7010657249343,
4.68459371607742));
#27915=CARTESIAN_POINT('Ctrl Pts',(-27.0384759968196,-90.4563699169912,
4.52661055082878));
#27916=CARTESIAN_POINT('Ctrl Pts',(-24.3677310199108,-88.6117992802222,
4.36862738558014));
#27917=CARTESIAN_POINT('Ctrl Pts',(-21.3634414594277,-89.8404423459467,
4.21064422033152));
#27918=CARTESIAN_POINT('Ctrl Pts',(-20.7506004806489,-93.0278779078959,
4.05266105508288));
#27919=CARTESIAN_POINT('Ctrl Pts',(-23.0850757871254,-95.2829931366425,
3.89467788983424));
#27920=CARTESIAN_POINT('Ctrl Pts',(-26.2494185580208,-94.5603215084427,
3.73669472458561));
#27921=CARTESIAN_POINT('Ctrl Pts',(-27.3734619703373,-91.5153509367788,
3.57871155933698));
#27922=CARTESIAN_POINT('Ctrl Pts',(-25.4376601278634,-88.9099734973746,
3.42072839408834));
#27923=CARTESIAN_POINT('Ctrl Pts',(-22.1978516918172,-89.1073557901304,
3.26274522883971));
#27924=CARTESIAN_POINT('Ctrl Pts',(-20.5926528478276,-91.9284646537611,
3.10476206359107));
#27925=CARTESIAN_POINT('Ctrl Pts',(-22.0780350586153,-94.8144594567856,
2.94677889834244));
#27926=CARTESIAN_POINT('Ctrl Pts',(-25.3067032590667,-95.1476415518446,
2.7887957330938));
#27927=CARTESIAN_POINT('Ctrl Pts',(-27.3501507055963,-92.6258092390124,
2.63081256784517));
#27928=CARTESIAN_POINT('Ctrl Pts',(-26.3548895523608,-89.5363385897163,
2.47282940259653));
#27929=CARTESIAN_POINT('Ctrl Pts',(-23.223678641653,-88.6815092609377,2.3148462373479));
#27930=CARTESIAN_POINT('Ctrl Pts',(-20.7965861590018,-90.8366309458652,
2.15686307209926));
#27931=CARTESIAN_POINT('Ctrl Pts',(-21.2751637872942,-94.0470361903508,
1.99887990685063));
#27932=CARTESIAN_POINT('Ctrl Pts',(-24.2251293032967,-95.4005706191734,
1.84089674160199));
#27933=CARTESIAN_POINT('Ctrl Pts',(-26.9711635487424,-93.6699555592399,
1.68291357635336));
#27934=CARTESIAN_POINT('Ctrl Pts',(-27.0217022824422,-90.4240534771338,
1.52493041110472));
#27935=CARTESIAN_POINT('Ctrl Pts',(-24.3325748270696,-88.6087741969446,
1.36694724585609));
#27936=CARTESIAN_POINT('Ctrl Pts',(-21.3394999866892,-89.8670182519309,
1.20896408060746));
#27937=CARTESIAN_POINT('Ctrl Pts',(-20.7643189008962,-93.0649591913859,
1.05098091535882));
#27938=CARTESIAN_POINT('Ctrl Pts',(-22.3308555140066,-94.5433639279422,
0.945658805193066));
#27939=CARTESIAN_POINT('Ctrl Pts',(-23.2540671456531,-94.7901775698421,
0.892997750110188));
#27940=CARTESIAN_POINT('Ctrl Pts',(-21.6639373423038,-90.0026984430693,
10.3210067496694));
#27941=CARTESIAN_POINT('Ctrl Pts',(-21.0030718657857,-90.7756529106096,
10.2683456945866));
#27942=CARTESIAN_POINT('Ctrl Pts',(-20.5204111561734,-93.0164835131759,
10.1630235844208));
#27943=CARTESIAN_POINT('Ctrl Pts',(-22.9525228428248,-95.474314673475,10.0050404191722));
#27944=CARTESIAN_POINT('Ctrl Pts',(-26.3358599455363,-94.7735796108867,
9.84705725392353));
#27945=CARTESIAN_POINT('Ctrl Pts',(-27.5999507940291,-91.5606287345722,
9.6890740886749));
#27946=CARTESIAN_POINT('Ctrl Pts',(-25.5990318095031,-88.7444872358932,
9.53109092342626));
#27947=CARTESIAN_POINT('Ctrl Pts',(-22.1476049582095,-88.8820466605266,
9.37310775817762));
#27948=CARTESIAN_POINT('Ctrl Pts',(-20.3764280027803,-91.847285042836,9.21512459292899));
#27949=CARTESIAN_POINT('Ctrl Pts',(-21.8919230124438,-94.9512424150719,
9.05714142768036));
#27950=CARTESIAN_POINT('Ctrl Pts',(-25.3195312348388,-95.3782236147545,
8.89915826243172));
#27951=CARTESIAN_POINT('Ctrl Pts',(-27.5502720327727,-92.7410889535148,
8.74117509718309));
#27952=CARTESIAN_POINT('Ctrl Pts',(-26.5607986183176,-89.4317376846897,
8.58319193193445));
#27953=CARTESIAN_POINT('Ctrl Pts',(-23.2485916399684,-88.4518995672047,
8.42520876668582));
#27954=CARTESIAN_POINT('Ctrl Pts',(-20.6179385783441,-90.6903039808948,
8.26722560143718));
#27955=CARTESIAN_POINT('Ctrl Pts',(-21.0549302288588,-94.116650160768,8.10924243618856));
#27956=CARTESIAN_POINT('Ctrl Pts',(-24.1632008959979,-95.6231210406981,
7.95125927093991));
#27957=CARTESIAN_POINT('Ctrl Pts',(-27.1234426759463,-93.8432981369136,
7.79327610569129));
#27958=CARTESIAN_POINT('Ctrl Pts',(-27.2506153900006,-90.391540581579,7.63529294044264));
#27959=CARTESIAN_POINT('Ctrl Pts',(-24.4293689698895,-88.3987107783728,
7.47730977519402));
#27960=CARTESIAN_POINT('Ctrl Pts',(-21.2186702510283,-89.672373140829,7.31932660994537));
#27961=CARTESIAN_POINT('Ctrl Pts',(-20.5307325412461,-93.057272549676,7.16134344469675));
#27962=CARTESIAN_POINT('Ctrl Pts',(-22.9895388330194,-95.4831896502703,
7.0033602794481));
#27963=CARTESIAN_POINT('Ctrl Pts',(-26.364867891015,-94.7497348585049,6.84537711419948));
#27964=CARTESIAN_POINT('Ctrl Pts',(-27.5951810545518,-91.5221766912428,
6.68739394895083));
#27965=CARTESIAN_POINT('Ctrl Pts',(-25.5645422900302,-88.7280205763547,
6.52941078370221));
#27966=CARTESIAN_POINT('Ctrl Pts',(-22.114810267437,-88.9016614773084,6.37142761845357));
#27967=CARTESIAN_POINT('Ctrl Pts',(-20.3750096777634,-91.8856011718064,
6.21344445320494));
#27968=CARTESIAN_POINT('Ctrl Pts',(-21.923199039088,-94.9733045078939,6.0554612879563));
#27969=CARTESIAN_POINT('Ctrl Pts',(-25.3551177576112,-95.3641191701941,
5.89747812270767));
#27970=CARTESIAN_POINT('Ctrl Pts',(-27.5578984169117,-92.7035629204621,
5.73949495745903));
#27971=CARTESIAN_POINT('Ctrl Pts',(-26.533543773379,-89.4048510878016,5.5815117922104));
#27972=CARTESIAN_POINT('Ctrl Pts',(-23.2111784520928,-88.4600278964635,
5.42352862696177));
#27973=CARTESIAN_POINT('Ctrl Pts',(-20.6043011989706,-90.7260802299217,
5.26554546171313));
#27974=CARTESIAN_POINT('Ctrl Pts',(-21.0774386607742,-94.1476212763577,
5.1075622964645));
#27975=CARTESIAN_POINT('Ctrl Pts',(-24.2014390107181,-95.6211965224102,
4.94957913121586));
#27976=CARTESIAN_POINT('Ctrl Pts',(-27.1427273020292,-93.8102229230488,
4.79159596596723));
#27977=CARTESIAN_POINT('Ctrl Pts',(-27.2334546631283,-90.3573153464849,
4.63361280071859));
#27978=CARTESIAN_POINT('Ctrl Pts',(-24.3913282785028,-88.3943788173915,
4.47562963546995));
#27979=CARTESIAN_POINT('Ctrl Pts',(-21.1942537915233,-89.7018637718047,
4.31764647022133));
#27980=CARTESIAN_POINT('Ctrl Pts',(-20.5420868753907,-93.0938367187666,
4.15966330497269));
#27981=CARTESIAN_POINT('Ctrl Pts',(-23.026365202284,-95.4936624405808,4.00168013972406));
#27982=CARTESIAN_POINT('Ctrl Pts',(-26.3937634963623,-94.7246170544863,
3.84369697447542));
#27983=CARTESIAN_POINT('Ctrl Pts',(-27.5899366492579,-91.4842510603691,
3.68571380922678));
#27984=CARTESIAN_POINT('Ctrl Pts',(-25.5299146181504,-88.7116868408497,
3.52773064397815));
#27985=CARTESIAN_POINT('Ctrl Pts',(-22.0822080355935,-88.9217351333484,
3.36974747872952));
#27986=CARTESIAN_POINT('Ctrl Pts',(-20.3740037605626,-91.92387423856,3.21176431348088));
#27987=CARTESIAN_POINT('Ctrl Pts',(-21.9547027823836,-94.99506300667,3.05378114823225));
#27988=CARTESIAN_POINT('Ctrl Pts',(-25.3905542616683,-95.349625359661,2.89579798298362));
#27989=CARTESIAN_POINT('Ctrl Pts',(-27.5651295032547,-92.6659673481809,
2.73781481773498));
#27990=CARTESIAN_POINT('Ctrl Pts',(-26.5060025526623,-89.3782457114063,
2.57983165248635));
#27991=CARTESIAN_POINT('Ctrl Pts',(-23.1738621865499,-88.4685620798055,
2.42184848723771));
#27992=CARTESIAN_POINT('Ctrl Pts',(-20.5910234496019,-90.7619776832305,
2.26386532198907));
#27993=CARTESIAN_POINT('Ctrl Pts',(-21.1003113510007,-94.1783942746989,
2.10588215674044));
#27994=CARTESIAN_POINT('Ctrl Pts',(-24.2395758256157,-95.6187848570707,
1.94789899149181));
#27995=CARTESIAN_POINT('Ctrl Pts',(-27.1618227827549,-93.7771164214867,
1.78991582624317));
#27996=CARTESIAN_POINT('Ctrl Pts',(-27.2156045813675,-90.3229251642809,
1.63193266099454));
#27997=CARTESIAN_POINT('Ctrl Pts',(-24.3539161166825,-88.3911596148569,
1.4739494957459));
#27998=CARTESIAN_POINT('Ctrl Pts',(-21.1687759971456,-89.7301450507159,
1.31596633049727));
#27999=CARTESIAN_POINT('Ctrl Pts',(-20.5566856051374,-93.1332975040884,
1.15798316524863));
#28000=CARTESIAN_POINT('Ctrl Pts',(-22.2237466982397,-94.7065713079336,
1.05266105508288));
#28001=CARTESIAN_POINT('Ctrl Pts',(-23.2062007174672,-94.9692229537457,
0.999999999999999));
#28002=CARTESIAN_POINT('Ctrl Pts',(-22.0865340033349,-90.364012796625,10.));
#28003=CARTESIAN_POINT('Ctrl Pts',(-22.0249229041794,-90.42191210108,10.));
#28004=CARTESIAN_POINT('Ctrl Pts',(-21.9666809070895,-90.4829619660093,
10.));
#28005=CARTESIAN_POINT('Ctrl Pts',(-21.9118056829835,-90.5467776153496,
10.));
#28006=CARTESIAN_POINT('Ctrl Pts',(-21.8554777542738,-90.612282647997,10.));
#28007=CARTESIAN_POINT('Ctrl Pts',(-21.8026967773226,-90.6807022716027,
10.));
#28008=CARTESIAN_POINT('Ctrl Pts',(-21.7534857403585,-90.751668886859,10.));
#28009=CARTESIAN_POINT('Ctrl Pts',(-21.7029132366757,-90.8245988560858,
10.));
#28010=CARTESIAN_POINT('Ctrl Pts',(-21.6561104020018,-90.9002192512322,
10.));
#28011=CARTESIAN_POINT('Ctrl Pts',(-21.6131362838788,-90.9781741250521,
10.));
#28012=CARTESIAN_POINT('Ctrl Pts',(-21.5942448480483,-91.0124431120789,
10.));
#28013=CARTESIAN_POINT('Ctrl Pts',(-21.5760937898788,-91.0471637309784,
10.));
#28014=CARTESIAN_POINT('Ctrl Pts',(-21.5586905433102,-91.0823078140376,
10.));
#28015=CARTESIAN_POINT('Ctrl Pts',(-21.5487655216201,-91.1023503839837,
10.));
#28016=CARTESIAN_POINT('Ctrl Pts',(-21.5390837455501,-91.122530701603,10.));
#28017=CARTESIAN_POINT('Ctrl Pts',(-21.5296468276344,-91.1428436902072,
10.));
#28018=CARTESIAN_POINT('Ctrl Pts',(-21.5211298019169,-91.1611766086332,
10.));
#28019=CARTESIAN_POINT('Ctrl Pts',(-21.5128098409547,-91.1796233420343,
10.));
#28020=CARTESIAN_POINT('Ctrl Pts',(-21.5047018248584,-91.1981483274791,
10.));
#28021=CARTESIAN_POINT('Ctrl Pts',(-21.468137058809,-91.281690559118,10.));
#28022=CARTESIAN_POINT('Ctrl Pts',(-21.435832611822,-91.3669162867985,10.));
#28023=CARTESIAN_POINT('Ctrl Pts',(-21.4078135856883,-91.4534267955088,
10.));
#28024=CARTESIAN_POINT('Ctrl Pts',(-21.3793318743036,-91.5413658740861,
10.));
#28025=CARTESIAN_POINT('Ctrl Pts',(-21.3552777914222,-91.6306332709131,
10.));
#28026=CARTESIAN_POINT('Ctrl Pts',(-21.3357167785958,-91.7208473131702,
10.));
#28027=CARTESIAN_POINT('Ctrl Pts',(-21.3167363466558,-91.8083837564149,
10.));
#28028=CARTESIAN_POINT('Ctrl Pts',(-21.3019860690135,-91.8968124021051,
10.));
#28029=CARTESIAN_POINT('Ctrl Pts',(-21.2915665512102,-91.9858064658359,
10.));
#28030=CARTESIAN_POINT('Ctrl Pts',(-21.2872071979573,-92.0230401045266,
10.));
#28031=CARTESIAN_POINT('Ctrl Pts',(-21.2836064360671,-92.0603729082663,
10.));
#28032=CARTESIAN_POINT('Ctrl Pts',(-21.2807739547557,-92.0977815592145,
10.));
#28033=CARTESIAN_POINT('Ctrl Pts',(-21.2790033727376,-92.1211656798516,
10.));
#28034=CARTESIAN_POINT('Ctrl Pts',(-21.2775330236673,-92.1445794431136,
10.));
#28035=CARTESIAN_POINT('Ctrl Pts',(-21.2763655645011,-92.1680171857376,
10.));
#28036=CARTESIAN_POINT('Ctrl Pts',(-21.2756812972385,-92.1817544370702,
10.));
#28037=CARTESIAN_POINT('Ctrl Pts',(-21.2751013563293,-92.1954953575252,
10.));
#28038=CARTESIAN_POINT('Ctrl Pts',(-21.2746262639777,-92.2092305726123,
10.));
#28039=CARTESIAN_POINT('Ctrl Pts',(-21.2712684324437,-92.3063075686709,
10.));
#28040=CARTESIAN_POINT('Ctrl Pts',(-21.2731377894438,-92.4032200227796,
10.));
#28041=CARTESIAN_POINT('Ctrl Pts',(-21.2802991313829,-92.4995456761415,
10.));
#28042=CARTESIAN_POINT('Ctrl Pts',(-21.2874604733219,-92.5958713295034,
10.));
#28043=CARTESIAN_POINT('Ctrl Pts',(-21.2999133653317,-92.6916112366308,
10.));
#28044=CARTESIAN_POINT('Ctrl Pts',(-21.3177754963829,-92.7863620775548,
10.));
#28045=CARTESIAN_POINT('Ctrl Pts',(-21.3348530128177,-92.8769508789951,
10.));
#28046=CARTESIAN_POINT('Ctrl Pts',(-21.3568748775386,-92.9666365695189,
10.));
#28047=CARTESIAN_POINT('Ctrl Pts',(-21.3835663946288,-93.0551798098071,
10.));
#28048=CARTESIAN_POINT('Ctrl Pts',(-21.3925012626256,-93.0848192702138,
10.));
#28049=CARTESIAN_POINT('Ctrl Pts',(-21.4019598223812,-93.1143306773249,
10.));
#28050=CARTESIAN_POINT('Ctrl Pts',(-21.4119330456339,-93.1437048746533,
10.));
#28051=CARTESIAN_POINT('Ctrl Pts',(-21.4184142793756,-93.1627940932574,
10.));
#28052=CARTESIAN_POINT('Ctrl Pts',(-21.4251128797724,-93.1818253626268,
10.));
#28053=CARTESIAN_POINT('Ctrl Pts',(-21.4320265053981,-93.2007961347298,
10.));
#28054=CARTESIAN_POINT('Ctrl Pts',(-21.4386160833976,-93.2188777302993,
10.));
#28055=CARTESIAN_POINT('Ctrl Pts',(-21.4454027538013,-93.2369085767537,
10.));
#28056=CARTESIAN_POINT('Ctrl Pts',(-21.4523736968937,-93.2548593171236,
10.));
#28057=CARTESIAN_POINT('Ctrl Pts',(-21.4862171782416,-93.3420090096165,
10.));
#28058=CARTESIAN_POINT('Ctrl Pts',(-21.5244390025882,-93.4273844054068,
10.));
#28059=CARTESIAN_POINT('Ctrl Pts',(-21.566707986091,-93.5107518898265,10.));
#28060=CARTESIAN_POINT('Ctrl Pts',(-21.6105462295651,-93.5972144393595,
10.));
#28061=CARTESIAN_POINT('Ctrl Pts',(-21.658737839251,-93.6815179448056,10.));
#28062=CARTESIAN_POINT('Ctrl Pts',(-21.7109693333793,-93.7633987878851,
10.));
#28063=CARTESIAN_POINT('Ctrl Pts',(-21.7637892526044,-93.8462020771595,
10.));
#28064=CARTESIAN_POINT('Ctrl Pts',(-21.8207410024304,-93.9265286302991,
10.));
#28065=CARTESIAN_POINT('Ctrl Pts',(-21.8815521717217,-94.0040909732374,
10.));
#28066=CARTESIAN_POINT('Ctrl Pts',(-21.9232146414969,-94.0572298752848,
10.));
#28067=CARTESIAN_POINT('Ctrl Pts',(-21.9666897223061,-94.1090710101977,
10.));
#28068=CARTESIAN_POINT('Ctrl Pts',(-22.0119020259848,-94.1595148903617,
10.));
#28069=CARTESIAN_POINT('Ctrl Pts',(-22.0240091589624,-94.1730229559845,
10.));
#28070=CARTESIAN_POINT('Ctrl Pts',(-22.0362421971848,-94.1864320425615,
10.));
#28071=CARTESIAN_POINT('Ctrl Pts',(-22.0485860744409,-94.1997257421532,
10.));
#28072=CARTESIAN_POINT('Ctrl Pts',(-22.1172469211216,-94.2736698239476,
10.));
#28073=CARTESIAN_POINT('Ctrl Pts',(-22.1894216591264,-94.3441460198121,
10.));
#28074=CARTESIAN_POINT('Ctrl Pts',(-22.2647998275067,-94.4108645190983,
10.));
#28075=CARTESIAN_POINT('Ctrl Pts',(-22.3277047217446,-94.4665427112258,
10.));
#28076=CARTESIAN_POINT('Ctrl Pts',(-22.3928416636934,-94.5196039171525,
10.));
#28077=CARTESIAN_POINT('Ctrl Pts',(-22.4600538825451,-94.5698659316683,
10.));
#28078=CARTESIAN_POINT('Ctrl Pts',(-22.4819361594785,-94.5862297318769,
10.));
#28079=CARTESIAN_POINT('Ctrl Pts',(-22.5040385610628,-94.6022967070182,
10.));
#28080=CARTESIAN_POINT('Ctrl Pts',(-22.5263561031885,-94.6180601837531,
10.));
#28081=CARTESIAN_POINT('Ctrl Pts',(-22.5491249077463,-94.6341423992097,
10.));
#28082=CARTESIAN_POINT('Ctrl Pts',(-22.5721230552632,-94.6499121464985,
10.));
#28083=CARTESIAN_POINT('Ctrl Pts',(-22.5953161167533,-94.6653431121406,
10.));
#28084=CARTESIAN_POINT('Ctrl Pts',(-22.6802614455734,-94.7218595168873,
10.));
#28085=CARTESIAN_POINT('Ctrl Pts',(-22.7678730455798,-94.7738754900138,
10.));
#28086=CARTESIAN_POINT('Ctrl Pts',(-22.8578606517821,-94.8210829659429,
10.));
#28087=CARTESIAN_POINT('Ctrl Pts',(-22.9411342809957,-94.8647682912064,
10.));
#28088=CARTESIAN_POINT('Ctrl Pts',(-23.0264434122392,-94.9043361313526,
10.));
#28089=CARTESIAN_POINT('Ctrl Pts',(-23.1135854408295,-94.9395135107766,
10.));
#28090=CARTESIAN_POINT('Ctrl Pts',(-23.1436093918511,-94.9516335398141,
10.));
#28091=CARTESIAN_POINT('Ctrl Pts',(-23.173851123563,-94.9632321026033,10.));
#28092=CARTESIAN_POINT('Ctrl Pts',(-23.2042982523172,-94.9743127795766,
10.));
#28093=CARTESIAN_POINT('Ctrl Pts',(-26.5182106813093,-92.0021944371302,
8.38741669750803));
#28094=CARTESIAN_POINT('Ctrl Pts',(-26.5197766683662,-92.1747250448626,
8.39833391417657));
#28095=CARTESIAN_POINT('Ctrl Pts',(-26.5035406983691,-92.3469627335709,
8.40925113084512));
#28096=CARTESIAN_POINT('Ctrl Pts',(-26.4684111368875,-92.5152564032994,
8.42016834751366));
#28097=CARTESIAN_POINT('Ctrl Pts',(-26.2989577103971,-93.3270495993809,
8.47282940259654));
#28098=CARTESIAN_POINT('Ctrl Pts',(-25.6898920459756,-94.0470741652581,
8.52549045767941));
#28099=CARTESIAN_POINT('Ctrl Pts',(-24.9174342801995,-94.3487964872293,
8.57815151276229));
#28100=CARTESIAN_POINT('Ctrl Pts',(-24.1449765144233,-94.6505188092004,
8.63081256784517));
#28101=CARTESIAN_POINT('Ctrl Pts',(-23.2091266472925,-94.5339388872655,
8.68347362292804));
#28102=CARTESIAN_POINT('Ctrl Pts',(-22.5343117030538,-94.0519076603904,
8.73613467801092));
#28103=CARTESIAN_POINT('Ctrl Pts',(-21.859496758815,-93.5698764335152,8.7887957330938));
#28104=CARTESIAN_POINT('Ctrl Pts',(-21.4457167374683,-92.7223939016998,
8.84145678817668));
#28105=CARTESIAN_POINT('Ctrl Pts',(-21.4806215310513,-91.8938487950316,
8.89411784325956));
#28106=CARTESIAN_POINT('Ctrl Pts',(-21.5155263246344,-91.0653036883635,
8.94677889834244));
#28107=CARTESIAN_POINT('Ctrl Pts',(-21.9991159331473,-90.2556960068425,
8.99943995342531));
#28108=CARTESIAN_POINT('Ctrl Pts',(-22.7120873058182,-89.8321130406813,
9.05210100850819));
#28109=CARTESIAN_POINT('Ctrl Pts',(-23.4250586784891,-89.4085300745201,
9.10476206359107));
#28110=CARTESIAN_POINT('Ctrl Pts',(-24.3674118153181,-89.3709718237187,
9.15742311867395));
#28111=CARTESIAN_POINT('Ctrl Pts',(-25.1117467560304,-89.7366423606423,
9.21008417375683));
#28112=CARTESIAN_POINT('Ctrl Pts',(-25.8560816967427,-90.102312897566,9.2627452288397));
#28113=CARTESIAN_POINT('Ctrl Pts',(-26.4023984413383,-90.8712122222148,
9.31540628392258));
#28114=CARTESIAN_POINT('Ctrl Pts',(-26.5029876085453,-91.6942825575571,
9.36806733900546));
#28115=CARTESIAN_POINT('Ctrl Pts',(-26.5153075025967,-91.7950900262914,
9.37451712517298));
#28116=CARTESIAN_POINT('Ctrl Pts',(-26.5209411710519,-91.8967100980969,
9.3809669113405));
#28117=CARTESIAN_POINT('Ctrl Pts',(-26.5201759878003,-91.9984131478585,
9.38741669750802));
#28118=CARTESIAN_POINT('Ctrl Pts',(-24.7937992825329,-94.9692229537457,
10.));
#28119=CARTESIAN_POINT('Ctrl Pts',(-25.7762533017603,-94.7065713079336,
9.94733894491712));
#28120=CARTESIAN_POINT('Ctrl Pts',(-27.4433142859563,-93.1332967687399,
9.84201683475136));
#28121=CARTESIAN_POINT('Ctrl Pts',(-26.8312240969782,-89.7301452717062,
9.68403366950274));
#28122=CARTESIAN_POINT('Ctrl Pts',(-23.6460838755241,-88.3911593875009,
9.52605050425409));
#28123=CARTESIAN_POINT('Ctrl Pts',(-20.7843953448966,-90.3229252160129,
9.36806733900547));
#28124=CARTESIAN_POINT('Ctrl Pts',(-20.8381771631847,-93.7771164103054,
9.21008417375682));
#28125=CARTESIAN_POINT('Ctrl Pts',(-23.7604241627304,-95.6187849549087,
9.05210100850819));
#28126=CARTESIAN_POINT('Ctrl Pts',(-26.8996887115742,-94.1783943047284,
8.89411784325956));
#28127=CARTESIAN_POINT('Ctrl Pts',(-27.4089766159342,-90.7619776656796,
8.73613467801092));
#28128=CARTESIAN_POINT('Ctrl Pts',(-24.8261378316183,-88.4685620052275,
8.57815151276229));
#28129=CARTESIAN_POINT('Ctrl Pts',(-21.493997396212,-89.3782456609066,8.42016834751366));
#28130=CARTESIAN_POINT('Ctrl Pts',(-20.4348704258473,-92.6659673604641,
8.26218518226503));
#28131=CARTESIAN_POINT('Ctrl Pts',(-22.6094457101907,-95.3496254273119,
8.10420201701638));
#28132=CARTESIAN_POINT('Ctrl Pts',(-26.0452972587431,-94.9950630663803,
7.94621885176775));
#28133=CARTESIAN_POINT('Ctrl Pts',(-27.6259963119893,-91.9238742371833,
7.78823568651911));
#28134=CARTESIAN_POINT('Ctrl Pts',(-25.9177920028682,-88.9217350716083,
7.63025252127049));
#28135=CARTESIAN_POINT('Ctrl Pts',(-22.4700853511787,-88.7116867750179,
7.47226935602185));
#28136=CARTESIAN_POINT('Ctrl Pts',(-20.4100632788413,-91.4842510500175,
7.31428619077321));
#28137=CARTESIAN_POINT('Ctrl Pts',(-21.6062364556795,-94.7246171090759,
7.15630302552459));
#28138=CARTESIAN_POINT('Ctrl Pts',(-24.9736348172233,-95.4936625105602,
6.99831986027594));
#28139=CARTESIAN_POINT('Ctrl Pts',(-27.4579131938761,-93.0938367406809,
6.84033669502731));
#28140=CARTESIAN_POINT('Ctrl Pts',(-26.8057462646821,-89.7018637257671,
6.68235352977867));
#28141=CARTESIAN_POINT('Ctrl Pts',(-23.6086717136575,-88.3943787451648,
6.52437036453005));
#28142=CARTESIAN_POINT('Ctrl Pts',(-20.7665452720997,-90.3573153135784,
6.36638719928141));
#28143=CARTESIAN_POINT('Ctrl Pts',(-20.8572726350159,-93.8102229593112,
6.20840403403277));
#28144=CARTESIAN_POINT('Ctrl Pts',(-23.7985609852469,-95.6211965949497,
6.05042086878414));
#28145=CARTESIAN_POINT('Ctrl Pts',(-26.9225613977704,-94.1476213193784,
5.8924377035355));
#28146=CARTESIAN_POINT('Ctrl Pts',(-27.3956988690517,-90.7260802044029,
5.73445453828687));
#28147=CARTESIAN_POINT('Ctrl Pts',(-24.7888215637087,-88.4600278255509,
5.57647137303823));
#28148=CARTESIAN_POINT('Ctrl Pts',(-21.4664561758692,-89.404851035816,5.41848820778961));
#28149=CARTESIAN_POINT('Ctrl Pts',(-20.4421015118168,-92.7035629345559,
5.26050504254096));
#28150=CARTESIAN_POINT('Ctrl Pts',(-22.6448822152433,-95.3641192375839,
5.10252187729233));
#28151=CARTESIAN_POINT('Ctrl Pts',(-26.0768010025144,-94.9733045674548,
4.94453871204369));
#28152=CARTESIAN_POINT('Ctrl Pts',(-27.6249903948521,-91.8856011695148,
4.78655554679506));
#28153=CARTESIAN_POINT('Ctrl Pts',(-25.8851897703268,-88.9016614152428,
4.62857238154642));
#28154=CARTESIAN_POINT('Ctrl Pts',(-22.435457678629,-88.7280205108105,4.4705892162978));
#28155=CARTESIAN_POINT('Ctrl Pts',(-20.4048188734298,-91.5221766816716,
4.31260605104916));
#28156=CARTESIAN_POINT('Ctrl Pts',(-21.6351320616123,-94.7497349135865,
4.15462288580052));
#28157=CARTESIAN_POINT('Ctrl Pts',(-25.0104611872221,-95.4831897200468,
3.99663972055189));
#28158=CARTESIAN_POINT('Ctrl Pts',(-27.46926752825,-93.0572725708519,3.83865655530325));
#28159=CARTESIAN_POINT('Ctrl Pts',(-26.7813298046868,-89.6723730942085,
3.68067339005462));
#28160=CARTESIAN_POINT('Ctrl Pts',(-23.5706310215098,-88.3987107062197,
3.52269022480598));
#28161=CARTESIAN_POINT('Ctrl Pts',(-20.7493845448822,-90.3915405493825,
3.36470705955735));
#28162=CARTESIAN_POINT('Ctrl Pts',(-20.876557261488,-93.8432981737925,3.20672389430871));
#28163=CARTESIAN_POINT('Ctrl Pts',(-23.8367991007265,-95.6231211133646,
3.04874072906008));
#28164=CARTESIAN_POINT('Ctrl Pts',(-26.9450698301516,-94.1166502029988,
2.89075756381144));
#28165=CARTESIAN_POINT('Ctrl Pts',(-27.3820614893708,-90.6903039549832,
2.73277439856281));
#28166=CARTESIAN_POINT('Ctrl Pts',(-24.7514083751606,-88.4518994955133,
2.57479123331418));
#28167=CARTESIAN_POINT('Ctrl Pts',(-21.4392013302128,-89.4317376344075,
2.41680806806554));
#28168=CARTESIAN_POINT('Ctrl Pts',(-20.4497278964894,-92.7410889661721,
2.25882490281691));
#28169=CARTESIAN_POINT('Ctrl Pts',(-22.6804687378898,-95.3782236865055,
2.10084173756827));
#28170=CARTESIAN_POINT('Ctrl Pts',(-26.1080770316232,-94.9512424666579,
1.94285857231964));
#28171=CARTESIAN_POINT('Ctrl Pts',(-27.6235720657977,-91.8472850535337,
1.78487540707101));
#28172=CARTESIAN_POINT('Ctrl Pts',(-25.852395087606,-88.8820465732967,1.62689224182237));
#28173=CARTESIAN_POINT('Ctrl Pts',(-22.4009681396119,-88.7444872144855,
1.46890907657374));
#28174=CARTESIAN_POINT('Ctrl Pts',(-20.4000491745082,-91.5606286501729,
1.3109259113251));
#28175=CARTESIAN_POINT('Ctrl Pts',(-21.6641399192573,-94.7735797938367,
1.15294274607647));
#28176=CARTESIAN_POINT('Ctrl Pts',(-25.0474773599211,-95.4743145446722,
0.994959580827833));
#28177=CARTESIAN_POINT('Ctrl Pts',(-27.4795883375449,-93.0164840574888,
0.836976415579199));
#28178=CARTESIAN_POINT('Ctrl Pts',(-26.9969281342143,-90.7756529106095,
0.731654305413442));
#28179=CARTESIAN_POINT('Ctrl Pts',(-26.3360626576961,-90.0026984430693,
0.678993250330564));
#28180=CARTESIAN_POINT('Ctrl Pts',(-24.745932854347,-94.7901775698421,10.1070022498898));
#28181=CARTESIAN_POINT('Ctrl Pts',(-25.6691444859934,-94.5433639279422,
10.0543411948069));
#28182=CARTESIAN_POINT('Ctrl Pts',(-27.2356809967647,-93.0649585003793,
9.94901908464118));
#28183=CARTESIAN_POINT('Ctrl Pts',(-26.6605001017588,-89.8670184595953,
9.79103591939254));
#28184=CARTESIAN_POINT('Ctrl Pts',(-23.6674251656069,-88.6087739832982,
9.6330527541439));
#28185=CARTESIAN_POINT('Ctrl Pts',(-20.9782976482682,-90.4240535257464,
9.47506958889527));
#28186=CARTESIAN_POINT('Ctrl Pts',(-21.028836400457,-93.6699555487327,9.31708642364663));
#28187=CARTESIAN_POINT('Ctrl Pts',(-23.7748706857521,-95.4005707111119,
9.159103258398));
#28188=CARTESIAN_POINT('Ctrl Pts',(-26.7248362715075,-94.0470362185693,
9.00112009314937));
#28189=CARTESIAN_POINT('Ctrl Pts',(-27.2034139025825,-90.8366309293727,
8.84313692790074));
#28190=CARTESIAN_POINT('Ctrl Pts',(-24.7763213754196,-88.6815091908567,
8.68515376265209));
#28191=CARTESIAN_POINT('Ctrl Pts',(-21.6451103995964,-89.5363385422618,
8.52717059740347));
#28192=CARTESIAN_POINT('Ctrl Pts',(-20.6498492277809,-92.6258092505549,
8.36918743215483));
#28193=CARTESIAN_POINT('Ctrl Pts',(-22.6932967144892,-95.147641615416,8.2112042669062));
#28194=CARTESIAN_POINT('Ctrl Pts',(-25.9219649800314,-94.8144595128954,
8.05322110165755));
#28195=CARTESIAN_POINT('Ctrl Pts',(-27.4073472203494,-91.9284646524673,
7.89523793640893));
#28196=CARTESIAN_POINT('Ctrl Pts',(-25.8021483443253,-89.1073557321131,
7.73725477116029));
#28197=CARTESIAN_POINT('Ctrl Pts',(-22.5623398433152,-88.9099734355125,
7.57927160591166));
#28198=CARTESIAN_POINT('Ctrl Pts',(-20.6265379620976,-91.5153509270514,
7.42128844066302));
#28199=CARTESIAN_POINT('Ctrl Pts',(-21.7505813969129,-94.5603215597406,
7.26330527541439));
#28200=CARTESIAN_POINT('Ctrl Pts',(-24.9149242312056,-95.2829932024021,
7.10532211016575));
#28201=CARTESIAN_POINT('Ctrl Pts',(-27.2493995844411,-93.0278779284887,
6.94733894491712));
#28202=CARTESIAN_POINT('Ctrl Pts',(-26.6365585933884,-89.8404423026853,
6.78935577966849));
#28203=CARTESIAN_POINT('Ctrl Pts',(-23.6322689727223,-88.6117992123508,
6.63137261441985));
#28204=CARTESIAN_POINT('Ctrl Pts',(-20.9615239423141,-90.4563698860691,
6.47338944917121));
#28205=CARTESIAN_POINT('Ctrl Pts',(-21.0467804073635,-93.7010657590101,
6.31540628392259));
#28206=CARTESIAN_POINT('Ctrl Pts',(-23.8107078419469,-95.4028369282512,
6.15742311867394));
#28207=CARTESIAN_POINT('Ctrl Pts',(-26.7463297251756,-94.0181188570853,
5.99943995342532));
#28208=CARTESIAN_POINT('Ctrl Pts',(-27.1909368093811,-90.8028980999997,
5.84145678817668));
#28209=CARTESIAN_POINT('Ctrl Pts',(-24.7412552940463,-88.6734896257781,
5.68347362292804));
#28210=CARTESIAN_POINT('Ctrl Pts',(-21.6192299263401,-89.5613396019551,
5.52549045767942));
#28211=CARTESIAN_POINT('Ctrl Pts',(-20.6566442762471,-92.661137795831,5.36750729243077));
#28212=CARTESIAN_POINT('Ctrl Pts',(-22.7265963834907,-95.1612614428767,
5.20952412718215));
#28213=CARTESIAN_POINT('Ctrl Pts',(-25.951569034899,-94.7940130605404,5.0515409619335));
#28214=CARTESIAN_POINT('Ctrl Pts',(-27.4064019604355,-91.8924994667599,
4.89355779668488));
#28215=CARTESIAN_POINT('Ctrl Pts',(-25.7715120400192,-89.0884925256083,
4.73557463143623));
#28216=CARTESIAN_POINT('Ctrl Pts',(-22.529800233879,-88.9253222402167,4.5775914661876));
#28217=CARTESIAN_POINT('Ctrl Pts',(-20.6216097965221,-91.5509896272809,
4.41960830093897));
#28218=CARTESIAN_POINT('Ctrl Pts',(-21.7777345857426,-94.5839247501514,
4.26162513569033));
#28219=CARTESIAN_POINT('Ctrl Pts',(-24.9495299557167,-95.2731519255295,
4.1036419704417));
#28220=CARTESIAN_POINT('Ctrl Pts',(-27.2600692477113,-92.9935185933678,
3.94565880519307));
#28221=CARTESIAN_POINT('Ctrl Pts',(-26.6136144561259,-89.8127299685233,
3.78767563994443));
#28222=CARTESIAN_POINT('Ctrl Pts',(-23.5965221501949,-88.6158699543453,
3.6296924746958));
#28223=CARTESIAN_POINT('Ctrl Pts',(-20.9453980141133,-90.4885313258635,
3.47170930944716));
#28224=CARTESIAN_POINT('Ctrl Pts',(-21.0649021628071,-93.7321465242476,
3.31372614419853));
#28225=CARTESIAN_POINT('Ctrl Pts',(-23.8466401830969,-95.4046453974022,
3.15574297894989));
#28226=CARTESIAN_POINT('Ctrl Pts',(-26.7674808896859,-93.9890153119552,
2.99775981370126));
#28227=CARTESIAN_POINT('Ctrl Pts',(-27.1781217693893,-90.7692791733585,
2.83977664845263));
#28228=CARTESIAN_POINT('Ctrl Pts',(-24.7060981363894,-88.6658514374356,
2.68179348320399));
#28229=CARTESIAN_POINT('Ctrl Pts',(-21.593618559257,-89.5866049274252,2.52381031795535));
#28230=CARTESIAN_POINT('Ctrl Pts',(-20.6638107867396,-92.6964009920719,
2.36582715270672));
#28231=CARTESIAN_POINT('Ctrl Pts',(-22.7600370239625,-95.1745153876391,
2.20784398745808));
#28232=CARTESIAN_POINT('Ctrl Pts',(-25.9809591063933,-94.7732813136335,
2.04986082220945));
#28233=CARTESIAN_POINT('Ctrl Pts',(-27.4050691572154,-91.8564938285714,
1.89187765696081));
#28234=CARTESIAN_POINT('Ctrl Pts',(-25.7406948903597,-89.0700604668216,
1.73389449171218));
#28235=CARTESIAN_POINT('Ctrl Pts',(-22.4973904284657,-88.9407959947845,
1.57591132646355));
#28236=CARTESIAN_POINT('Ctrl Pts',(-20.6171277124371,-91.587122926026,1.41792816121491));
#28237=CARTESIAN_POINT('Ctrl Pts',(-21.8049932574595,-94.606331774166,1.25994499596628));
#28238=CARTESIAN_POINT('Ctrl Pts',(-24.9843140377459,-95.2648119269358,
1.10196183071764));
#28239=CARTESIAN_POINT('Ctrl Pts',(-27.2697677078963,-92.9551896443915,
0.943978665469009));
#28240=CARTESIAN_POINT('Ctrl Pts',(-26.8162121163602,-90.8494815513232,
0.838656555303253));
#28241=CARTESIAN_POINT('Ctrl Pts',(-26.1951971040191,-90.1231365609212,
0.785995500220375));
#28242=CARTESIAN_POINT('Ctrl Pts',(-24.698066426161,-94.6111321859386,10.2140044997796));
#28243=CARTESIAN_POINT('Ctrl Pts',(-25.5620356702265,-94.3801565479507,
10.1613434446967));
#28244=CARTESIAN_POINT('Ctrl Pts',(-27.028047707573,-92.9966202320186,10.056021334531));
#28245=CARTESIAN_POINT('Ctrl Pts',(-26.4897761065395,-90.0038916474845,
9.89803816928236));
#28246=CARTESIAN_POINT('Ctrl Pts',(-23.6887664556898,-88.8263885790956,
9.74005500403371));
#28247=CARTESIAN_POINT('Ctrl Pts',(-21.1721999516397,-90.5251818354797,
9.58207183878509));
#28248=CARTESIAN_POINT('Ctrl Pts',(-21.2194956377293,-93.5627946871602,
9.42408867353644));
#28249=CARTESIAN_POINT('Ctrl Pts',(-23.7893172087738,-95.1823564673149,
9.26610550828781));
#28250=CARTESIAN_POINT('Ctrl Pts',(-26.5499838314408,-93.9156781324104,
9.10812234303918));
#28251=CARTESIAN_POINT('Ctrl Pts',(-26.9978511892308,-90.9112841930657,
8.95013917779054));
#28252=CARTESIAN_POINT('Ctrl Pts',(-24.7265049192209,-88.8944563764859,
8.79215601254191));
#28253=CARTESIAN_POINT('Ctrl Pts',(-21.7962234029808,-89.694431423617,8.63417284729327));
#28254=CARTESIAN_POINT('Ctrl Pts',(-20.8648280297145,-92.5856511406459,
8.47618968204465));
#28255=CARTESIAN_POINT('Ctrl Pts',(-22.7771477187876,-94.9456578035201,
8.318206516796));
#28256=CARTESIAN_POINT('Ctrl Pts',(-25.7986327013197,-94.6338559594106,
8.16022335154737));
#28257=CARTESIAN_POINT('Ctrl Pts',(-27.1886981287095,-91.9330550677512,
8.00224018629873));
#28258=CARTESIAN_POINT('Ctrl Pts',(-25.6865046857824,-89.2929763926183,
7.84425702105011));
#28259=CARTESIAN_POINT('Ctrl Pts',(-22.6545943354517,-89.1082600960069,
7.68627385580146));
#28260=CARTESIAN_POINT('Ctrl Pts',(-20.8430126453538,-91.5464508040853,
7.52829069055284));
#28261=CARTESIAN_POINT('Ctrl Pts',(-21.8949263381463,-94.3960260104053,
7.3703075253042));
#28262=CARTESIAN_POINT('Ctrl Pts',(-24.8562136451879,-95.0723238942441,
7.21232436005556));
#28263=CARTESIAN_POINT('Ctrl Pts',(-27.0408859750062,-92.9619191162963,
7.05434119480693));
#28264=CARTESIAN_POINT('Ctrl Pts',(-26.4673709220948,-89.9790208796034,
6.8963580295583));
#28265=CARTESIAN_POINT('Ctrl Pts',(-23.655866231787,-88.8292196795367,6.73837486430967));
#28266=CARTESIAN_POINT('Ctrl Pts',(-21.1565026125286,-90.5554244585598,
6.58039169906103));
#28267=CARTESIAN_POINT('Ctrl Pts',(-21.2362881797111,-93.5919085587089,
6.4224085338124));
#28268=CARTESIAN_POINT('Ctrl Pts',(-23.8228546986469,-95.1844772615529,
6.26442536856376));
#28269=CARTESIAN_POINT('Ctrl Pts',(-26.5700980525808,-93.8886163947921,
6.10644220331512));
#28270=CARTESIAN_POINT('Ctrl Pts',(-26.9861747497105,-90.8797159955968,
5.94845903806649));
#28271=CARTESIAN_POINT('Ctrl Pts',(-24.6936890243839,-88.8869514260051,
5.79047587281785));
#28272=CARTESIAN_POINT('Ctrl Pts',(-21.772003676811,-89.7178281680943,5.63249270756923));
#28273=CARTESIAN_POINT('Ctrl Pts',(-20.8711870406774,-92.6187126571061,
5.47450954232058));
#28274=CARTESIAN_POINT('Ctrl Pts',(-22.808310551738,-94.9584036481696,5.31652637707196));
#28275=CARTESIAN_POINT('Ctrl Pts',(-25.8263370672835,-94.6147215536259,
5.15854321182331));
#28276=CARTESIAN_POINT('Ctrl Pts',(-27.187813526019,-91.8993977640052,5.00056004657469));
#28277=CARTESIAN_POINT('Ctrl Pts',(-25.6578343097115,-89.2753236359738,
4.84257688132605));
#28278=CARTESIAN_POINT('Ctrl Pts',(-22.6241427891289,-89.1226239696228,
4.68459371607741));
#28279=CARTESIAN_POINT('Ctrl Pts',(-20.8384007196145,-91.5798025728902,
4.52661055082878));
#28280=CARTESIAN_POINT('Ctrl Pts',(-21.9203371098729,-94.4181145867162,
4.36862738558014));
#28281=CARTESIAN_POINT('Ctrl Pts',(-24.8885987242113,-95.0631141310124,
4.21064422033151));
#28282=CARTESIAN_POINT('Ctrl Pts',(-27.0508709671726,-92.9297646158834,
4.05266105508287));
#28283=CARTESIAN_POINT('Ctrl Pts',(-26.445899107565,-89.9530868428382,3.89467788983424));
#28284=CARTESIAN_POINT('Ctrl Pts',(-23.6224132788799,-88.8330292024708,
3.73669472458561));
#28285=CARTESIAN_POINT('Ctrl Pts',(-21.1414114833444,-90.5855221023446,
3.57871155933697));
#28286=CARTESIAN_POINT('Ctrl Pts',(-21.2532470641262,-93.6209948747027,
3.42072839408834));
#28287=CARTESIAN_POINT('Ctrl Pts',(-23.8564812654673,-95.18616968144,3.26274522883971));
#28288=CARTESIAN_POINT('Ctrl Pts',(-26.5898919492202,-93.8613804209116,
3.10476206359106));
#28289=CARTESIAN_POINT('Ctrl Pts',(-26.9741820494077,-90.8482543917338,
2.94677889834244));
#28290=CARTESIAN_POINT('Ctrl Pts',(-24.6607878976183,-88.8798033793578,
2.7887957330938));
#28291=CARTESIAN_POINT('Ctrl Pts',(-21.7480357883011,-89.741472220443,2.63081256784516));
#28292=CARTESIAN_POINT('Ctrl Pts',(-20.8778936769898,-92.6517130179715,
2.47282940259653));
#28293=CARTESIAN_POINT('Ctrl Pts',(-22.8396053100352,-94.9708070887728,
2.3148462373479));
#28294=CARTESIAN_POINT('Ctrl Pts',(-25.8538411811634,-94.595320160609,2.15686307209926));
#28295=CARTESIAN_POINT('Ctrl Pts',(-27.186566248633,-91.8657026036092,1.99887990685063));
#28296=CARTESIAN_POINT('Ctrl Pts',(-25.6289946931135,-89.2580743603465,
1.84089674160199));
#28297=CARTESIAN_POINT('Ctrl Pts',(-22.5938127173193,-89.1371047750836,
1.68291357635336));
#28298=CARTESIAN_POINT('Ctrl Pts',(-20.834206250366,-91.613617201879,1.52493041110472));
#28299=CARTESIAN_POINT('Ctrl Pts',(-21.9458465956616,-94.4390837544956,
1.36694724585609));
#28300=CARTESIAN_POINT('Ctrl Pts',(-24.9211507155708,-95.0553093091994,
1.20896408060745));
#28301=CARTESIAN_POINT('Ctrl Pts',(-27.0599470782477,-92.8938952312942,
1.05098091535882));
#28302=CARTESIAN_POINT('Ctrl Pts',(-26.6354960985062,-90.923310192037,0.945658805193063));
#28303=CARTESIAN_POINT('Ctrl Pts',(-26.054331550342,-90.2435746787731,0.892997750110186));
#28304=CARTESIAN_POINT('Ctrl Pts',(-24.6501999979751,-94.4320868020351,
10.3210067496694));
#28305=CARTESIAN_POINT('Ctrl Pts',(-25.4549268544596,-94.2169491679593,
10.2683456945866));
#28306=CARTESIAN_POINT('Ctrl Pts',(-26.8204144183814,-92.928281963658,10.1630235844208));
#28307=CARTESIAN_POINT('Ctrl Pts',(-26.3190521113202,-90.1407648353735,
10.0050404191722));
#28308=CARTESIAN_POINT('Ctrl Pts',(-23.7101077457725,-89.044003174893,9.84705725392353));
#28309=CARTESIAN_POINT('Ctrl Pts',(-21.3661022550113,-90.6263101452131,
9.6890740886749));
#28310=CARTESIAN_POINT('Ctrl Pts',(-21.4101548750016,-93.4556338255877,
9.53109092342626));
#28311=CARTESIAN_POINT('Ctrl Pts',(-23.8037637317956,-94.964142223518,9.37310775817762));
#28312=CARTESIAN_POINT('Ctrl Pts',(-26.375131391374,-93.7843200462514,9.21512459292899));
#28313=CARTESIAN_POINT('Ctrl Pts',(-26.7922884758791,-90.9859374567588,
9.05714142768035));
#28314=CARTESIAN_POINT('Ctrl Pts',(-24.6766884630223,-89.107403562115,8.89915826243172));
#28315=CARTESIAN_POINT('Ctrl Pts',(-21.9473364063653,-89.8525243049722,
8.74117509718308));
#28316=CARTESIAN_POINT('Ctrl Pts',(-21.0798068316481,-92.5454930307366,
8.58319193193445));
#28317=CARTESIAN_POINT('Ctrl Pts',(-22.8609987230861,-94.7436739916243,
8.42520876668582));
#28318=CARTESIAN_POINT('Ctrl Pts',(-25.6753004226081,-94.4532524059257,
8.26722560143718));
#28319=CARTESIAN_POINT('Ctrl Pts',(-26.9700490370695,-91.9376454830352,
8.10924243618854));
#28320=CARTESIAN_POINT('Ctrl Pts',(-25.5708610272396,-89.4785970531231,
7.95125927093992));
#28321=CARTESIAN_POINT('Ctrl Pts',(-22.7468488275882,-89.3065467565015,
7.79327610569128));
#28322=CARTESIAN_POINT('Ctrl Pts',(-21.0594873286101,-91.577550681119,7.63529294044264));
#28323=CARTESIAN_POINT('Ctrl Pts',(-22.0392712793796,-94.2317304610699,
7.47730977519402));
#28324=CARTESIAN_POINT('Ctrl Pts',(-24.7975030591702,-94.8616545860859,
7.31932660994537));
#28325=CARTESIAN_POINT('Ctrl Pts',(-26.8323723655712,-92.8959603041042,
7.16134344469674));
#28326=CARTESIAN_POINT('Ctrl Pts',(-26.2981832508011,-90.1175994565215,
7.00336027944811));
#28327=CARTESIAN_POINT('Ctrl Pts',(-23.6794634908517,-89.0466401467228,
6.84537711419948));
#28328=CARTESIAN_POINT('Ctrl Pts',(-21.3514812827431,-90.6544790310504,
6.68739394895084));
#28329=CARTESIAN_POINT('Ctrl Pts',(-21.4257959520587,-93.4827513584078,
6.5294107837022));
#28330=CARTESIAN_POINT('Ctrl Pts',(-23.835001555347,-94.9661175948546,6.37142761845357));
#28331=CARTESIAN_POINT('Ctrl Pts',(-26.393866379986,-93.7591139324989,6.21344445320494));
#28332=CARTESIAN_POINT('Ctrl Pts',(-26.7814126900399,-90.9565338911937,
6.0554612879563));
#28333=CARTESIAN_POINT('Ctrl Pts',(-24.6461227547216,-89.1004132262322,
5.89747812270766));
#28334=CARTESIAN_POINT('Ctrl Pts',(-21.9247774272818,-89.8743167342334,
5.73949495745903));
#28335=CARTESIAN_POINT('Ctrl Pts',(-21.0857298051078,-92.5762875183812,
5.5815117922104));
#28336=CARTESIAN_POINT('Ctrl Pts',(-22.8900247199853,-94.7555458534625,
5.42352862696176));
#28337=CARTESIAN_POINT('Ctrl Pts',(-25.7011050996681,-94.4354300467114,
5.26554546171313));
#28338=CARTESIAN_POINT('Ctrl Pts',(-26.9692250916024,-91.9062960612505,
5.1075622964645));
#28339=CARTESIAN_POINT('Ctrl Pts',(-25.5441565794039,-89.4621547463392,
4.94957913121586));
#28340=CARTESIAN_POINT('Ctrl Pts',(-22.7184853443789,-89.319925699029,4.79159596596723));
#28341=CARTESIAN_POINT('Ctrl Pts',(-21.0551916427068,-91.6086155184995,
4.63361280071859));
#28342=CARTESIAN_POINT('Ctrl Pts',(-22.0629396340032,-94.252304423281,4.47562963546995));
#28343=CARTESIAN_POINT('Ctrl Pts',(-24.8276674927059,-94.8530763364951,
4.31764647022132));
#28344=CARTESIAN_POINT('Ctrl Pts',(-26.841672686634,-92.8660106383991,4.15966330497269));
#28345=CARTESIAN_POINT('Ctrl Pts',(-26.2781837590041,-90.0934437171531,
4.00168013972405));
#28346=CARTESIAN_POINT('Ctrl Pts',(-23.648304407565,-89.0501884505964,3.84369697447542));
#28347=CARTESIAN_POINT('Ctrl Pts',(-21.3374249525755,-90.6825128788255,
3.68571380922678));
#28348=CARTESIAN_POINT('Ctrl Pts',(-21.4415919654453,-93.5098432251578,
3.52773064397815));
#28349=CARTESIAN_POINT('Ctrl Pts',(-23.8663223478376,-94.9676939654777,
3.36974747872952));
#28350=CARTESIAN_POINT('Ctrl Pts',(-26.4123030087544,-93.733745529868,3.21176431348088));
#28351=CARTESIAN_POINT('Ctrl Pts',(-26.7702423294261,-90.9272296101091,
3.05378114823225));
#28352=CARTESIAN_POINT('Ctrl Pts',(-24.6154776588472,-89.0937553212802,
2.89579798298361));
#28353=CARTESIAN_POINT('Ctrl Pts',(-21.9024530173453,-89.8963395134605,
2.73781481773497));
#28354=CARTESIAN_POINT('Ctrl Pts',(-21.09197656724,-92.6070250438713,2.57983165248634));
#28355=CARTESIAN_POINT('Ctrl Pts',(-22.9191735961078,-94.7670987899065,
2.42184848723771));
#28356=CARTESIAN_POINT('Ctrl Pts',(-25.7267232559334,-94.4173590075845,
2.26386532198907));
#28357=CARTESIAN_POINT('Ctrl Pts',(-26.9680633400506,-91.8749113786469,
2.10588215674044));
#28358=CARTESIAN_POINT('Ctrl Pts',(-25.5172944958673,-89.4460882538716,
1.94789899149181));
#28359=CARTESIAN_POINT('Ctrl Pts',(-22.6902350061731,-89.3334135553823,
1.78991582624317));
#28360=CARTESIAN_POINT('Ctrl Pts',(-21.051284788295,-91.6401114777323,1.63193266099454));
#28361=CARTESIAN_POINT('Ctrl Pts',(-22.0866999338637,-94.2718357348247,
1.4739494957459));
#28362=CARTESIAN_POINT('Ctrl Pts',(-24.8579873933956,-94.8458066914632,
1.31596633049727));
#28363=CARTESIAN_POINT('Ctrl Pts',(-26.8501264485991,-92.8326008181969,
1.15798316524863));
#28364=CARTESIAN_POINT('Ctrl Pts',(-26.4547800806521,-90.9971388327507,
1.05266105508287));
#28365=CARTESIAN_POINT('Ctrl Pts',(-25.913465996665,-90.364012796625,0.999999999999996));
#28366=CARTESIAN_POINT('Ctrl Pts',(-26.5149492652116,-91.9982505980886,
9.11258330249198));
#28367=CARTESIAN_POINT('Ctrl Pts',(-26.5168562980303,-91.7052247424894,
9.09410267755477));
#28368=CARTESIAN_POINT('Ctrl Pts',(-26.4695028989504,-91.412794780389,9.07562205261756));
#28369=CARTESIAN_POINT('Ctrl Pts',(-26.3701622929854,-91.1392455725669,
9.05714142768035));
#28370=CARTESIAN_POINT('Ctrl Pts',(-26.0870884715935,-90.3597594918776,
9.00448037259747));
#28371=CARTESIAN_POINT('Ctrl Pts',(-25.3818884673079,-89.7335815269963,
8.9518193175146));
#28372=CARTESIAN_POINT('Ctrl Pts',(-24.5743964557222,-89.5446793350319,
8.89915826243172));
#28373=CARTESIAN_POINT('Ctrl Pts',(-23.7669044441366,-89.3557771430674,
8.84649720734884));
#28374=CARTESIAN_POINT('Ctrl Pts',(-22.8571204252509,-89.6041507240198,
8.79383615226596));
#28375=CARTESIAN_POINT('Ctrl Pts',(-22.2576401533552,-90.1771656354567,
8.74117509718308));
#28376=CARTESIAN_POINT('Ctrl Pts',(-21.6581598814595,-90.7501805468937,
8.68851404210021));
#28377=CARTESIAN_POINT('Ctrl Pts',(-21.3689833565538,-91.6478367888151,
8.63585298701733));
#28378=CARTESIAN_POINT('Ctrl Pts',(-21.5212604093406,-92.4630284032571,
8.58319193193445));
#28379=CARTESIAN_POINT('Ctrl Pts',(-21.6735374621274,-93.2782200176992,
8.53053087685158));
#28380=CARTESIAN_POINT('Ctrl Pts',(-22.2672680926068,-94.0109470046617,
8.4778698217687));
#28381=CARTESIAN_POINT('Ctrl Pts',(-23.0331836911001,-94.3289069005266,
8.42520876668582));
#28382=CARTESIAN_POINT('Ctrl Pts',(-23.7990992895934,-94.6468667963914,
8.37254771160294));
#28383=CARTESIAN_POINT('Ctrl Pts',(-24.7371998561007,-94.5500596011586,
8.31988665652006));
#28384=CARTESIAN_POINT('Ctrl Pts',(-25.422041575098,-94.0823881830604,8.26722560143718));
#28385=CARTESIAN_POINT('Ctrl Pts',(-26.0924009622684,-93.6246066015112,
8.21567816845544));
#28386=CARTESIAN_POINT('Ctrl Pts',(-26.5200995637937,-92.8114802627189,
8.16413073547371));
#28387=CARTESIAN_POINT('Ctrl Pts',(-26.5215633824187,-91.9996804087644,
8.11258330249198));
#28388=CARTESIAN_POINT('Ctrl Pts',(-24.7937992825329,-94.9692229537457,
10.));
#28389=CARTESIAN_POINT('Ctrl Pts',(-24.8868523869064,-94.9351837125004,
10.));
#28390=CARTESIAN_POINT('Ctrl Pts',(-24.9778402151602,-94.896376143455,10.));
#28391=CARTESIAN_POINT('Ctrl Pts',(-25.0665542695767,-94.8531284786691,
10.));
#28392=CARTESIAN_POINT('Ctrl Pts',(-25.1572340298607,-94.8089225419499,
10.));
#28393=CARTESIAN_POINT('Ctrl Pts',(-25.2455388043612,-94.7600769477965,
10.));
#28394=CARTESIAN_POINT('Ctrl Pts',(-25.3312170072774,-94.7068966945096,
10.));
#28395=CARTESIAN_POINT('Ctrl Pts',(-25.4136695050773,-94.6557186285851,
10.));
#28396=CARTESIAN_POINT('Ctrl Pts',(-25.4936897697097,-94.6005252759114,
10.));
#28397=CARTESIAN_POINT('Ctrl Pts',(-25.5710205780852,-94.5415583960945,
10.));
#28398=CARTESIAN_POINT('Ctrl Pts',(-25.6386850354138,-94.4899623762547,
10.));
#28399=CARTESIAN_POINT('Ctrl Pts',(-25.7042900873087,-94.4354765516692,
10.));
#28400=CARTESIAN_POINT('Ctrl Pts',(-25.7676387673434,-94.3782501713689,
10.));
#28401=CARTESIAN_POINT('Ctrl Pts',(-25.7817376093299,-94.3655139045221,
10.));
#28402=CARTESIAN_POINT('Ctrl Pts',(-25.7957272919033,-94.3526391912685,
10.));
#28403=CARTESIAN_POINT('Ctrl Pts',(-25.8095861705285,-94.3396461050441,
10.));
#28404=CARTESIAN_POINT('Ctrl Pts',(-25.8820168750965,-94.2717402942496,
10.));
#28405=CARTESIAN_POINT('Ctrl Pts',(-25.9509819060194,-94.2005127260723,
10.));
#28406=CARTESIAN_POINT('Ctrl Pts',(-26.0162413172849,-94.1262540066716,
10.));
#28407=CARTESIAN_POINT('Ctrl Pts',(-26.0811410662591,-94.0524045471867,
10.));
#28408=CARTESIAN_POINT('Ctrl Pts',(-26.1423764147278,-93.9755564586353,
10.));
#28409=CARTESIAN_POINT('Ctrl Pts',(-26.1996677535222,-93.8959688011541,
10.));
#28410=CARTESIAN_POINT('Ctrl Pts',(-26.2548605589272,-93.8192963723989,
10.));
#28411=CARTESIAN_POINT('Ctrl Pts',(-26.3063931619513,-93.7400806580874,
10.));
#28412=CARTESIAN_POINT('Ctrl Pts',(-26.3539706372977,-93.6585396692493,
10.));
#28413=CARTESIAN_POINT('Ctrl Pts',(-26.3739594034205,-93.6242817826455,
10.));
#28414=CARTESIAN_POINT('Ctrl Pts',(-26.3932494781019,-93.5896133547583,
10.));
#28415=CARTESIAN_POINT('Ctrl Pts',(-26.4118163867695,-93.5545502531732,
10.));
#28416=CARTESIAN_POINT('Ctrl Pts',(-26.4248529713493,-93.5299310180799,
10.));
#28417=CARTESIAN_POINT('Ctrl Pts',(-26.4375330011256,-93.5051172053521,
10.));
#28418=CARTESIAN_POINT('Ctrl Pts',(-26.4498475176157,-93.480114301777,10.));
#28419=CARTESIAN_POINT('Ctrl Pts',(-26.4575999795916,-93.4643740119,10.));
#28420=CARTESIAN_POINT('Ctrl Pts',(-26.465208458444,-93.4485566581552,10.));
#28421=CARTESIAN_POINT('Ctrl Pts',(-26.4726610534608,-93.4326847361421,
10.));
#28422=CARTESIAN_POINT('Ctrl Pts',(-26.5147816015831,-93.3429798677795,
10.));
#28423=CARTESIAN_POINT('Ctrl Pts',(-26.5519999407493,-93.2513903181037,
10.));
#28424=CARTESIAN_POINT('Ctrl Pts',(-26.5840244250131,-93.158188555653,10.));
#28425=CARTESIAN_POINT('Ctrl Pts',(-26.6138868935444,-93.0712789687469,
10.));
#28426=CARTESIAN_POINT('Ctrl Pts',(-26.6392329460521,-92.9829667141397,
10.));
#28427=CARTESIAN_POINT('Ctrl Pts',(-26.6597755596719,-92.8934640331731,
10.));
#28428=CARTESIAN_POINT('Ctrl Pts',(-26.6612628263319,-92.8869841199622,
10.));
#28429=CARTESIAN_POINT('Ctrl Pts',(-26.6627248923853,-92.8804979658116,
10.));
#28430=CARTESIAN_POINT('Ctrl Pts',(-26.6641616381052,-92.8740056509469,
10.));
#28431=CARTESIAN_POINT('Ctrl Pts',(-26.6847472407915,-92.7809841702031,
10.));
#28432=CARTESIAN_POINT('Ctrl Pts',(-26.7001390631713,-92.6866969715701,
10.));
#28433=CARTESIAN_POINT('Ctrl Pts',(-26.7104141120204,-92.5915520773693,
10.));
#28434=CARTESIAN_POINT('Ctrl Pts',(-26.7162317525625,-92.5376818912505,
10.));
#28435=CARTESIAN_POINT('Ctrl Pts',(-26.7204081622487,-92.4835369406454,
10.));
#28436=CARTESIAN_POINT('Ctrl Pts',(-26.7229504259501,-92.429193979476,10.));
#28437=CARTESIAN_POINT('Ctrl Pts',(-26.7235977676582,-92.4153565222196,
10.));
#28438=CARTESIAN_POINT('Ctrl Pts',(-26.7241390041195,-92.401507632359,10.));
#28439=CARTESIAN_POINT('Ctrl Pts',(-26.7245740715224,-92.387660812466,10.));
#28440=CARTESIAN_POINT('Ctrl Pts',(-26.727502891379,-92.2944457364089,10.));
#28441=CARTESIAN_POINT('Ctrl Pts',(-26.7256323237373,-92.2011733961936,
10.));
#28442=CARTESIAN_POINT('Ctrl Pts',(-26.7190972361968,-92.1082190602615,
10.));
#28443=CARTESIAN_POINT('Ctrl Pts',(-26.7125517108832,-92.015116258641,10.));
#28444=CARTESIAN_POINT('Ctrl Pts',(-26.7013263747252,-91.9223314983086,
10.));
#28445=CARTESIAN_POINT('Ctrl Pts',(-26.6855058357789,-91.8302540028465,
10.));
#28446=CARTESIAN_POINT('Ctrl Pts',(-26.6699124599891,-91.7394986250815,
10.));
#28447=CARTESIAN_POINT('Ctrl Pts',(-26.6498544352219,-91.6494295035836,
10.));
#28448=CARTESIAN_POINT('Ctrl Pts',(-26.6253697912314,-91.5604445847042,
10.));
#28449=CARTESIAN_POINT('Ctrl Pts',(-26.6161277167569,-91.5268559710524,
10.));
#28450=CARTESIAN_POINT('Ctrl Pts',(-26.606254534053,-91.4934221580589,10.));
#28451=CARTESIAN_POINT('Ctrl Pts',(-26.5957508647621,-91.4601658756637,
10.));
#28452=CARTESIAN_POINT('Ctrl Pts',(-26.5880548971476,-91.4357992219538,
10.));
#28453=CARTESIAN_POINT('Ctrl Pts',(-26.5800204435636,-91.411527889357,10.));
#28454=CARTESIAN_POINT('Ctrl Pts',(-26.5716475015492,-91.3873611147699,
10.));
#28455=CARTESIAN_POINT('Ctrl Pts',(-26.5664800361945,-91.372446289109,10.));
#28456=CARTESIAN_POINT('Ctrl Pts',(-26.5611866348768,-91.3575799762243,
10.));
#28457=CARTESIAN_POINT('Ctrl Pts',(-26.5557684843854,-91.3427662651665,
10.));
#28458=CARTESIAN_POINT('Ctrl Pts',(-26.5240624592361,-91.2560791389784,
10.));
#28459=CARTESIAN_POINT('Ctrl Pts',(-26.4880796645469,-91.1711661845881,
10.));
#28460=CARTESIAN_POINT('Ctrl Pts',(-26.4478804014549,-91.0884282233226,
10.));
#28461=CARTESIAN_POINT('Ctrl Pts',(-26.417730954136,-91.0263747523735,10.));
#28462=CARTESIAN_POINT('Ctrl Pts',(-26.3852087542102,-90.9655451999197,
10.));
#28463=CARTESIAN_POINT('Ctrl Pts',(-26.3503241512938,-90.9061236582789,
10.));
#28464=CARTESIAN_POINT('Ctrl Pts',(-26.3345452493638,-90.879246279731,10.));
#28465=CARTESIAN_POINT('Ctrl Pts',(-26.3182828568508,-90.8526571659942,
10.));
#28466=CARTESIAN_POINT('Ctrl Pts',(-26.3015371511582,-90.8263744220268,
10.));
#28467=CARTESIAN_POINT('Ctrl Pts',(-26.2924151855709,-90.8120573015417,
10.));
#28468=CARTESIAN_POINT('Ctrl Pts',(-26.2831549824545,-90.7978392516847,
10.));
#28469=CARTESIAN_POINT('Ctrl Pts',(-26.2737572212358,-90.783723284612,10.));
#28470=CARTESIAN_POINT('Ctrl Pts',(-26.2261821464327,-90.7122628406009,
10.));
#28471=CARTESIAN_POINT('Ctrl Pts',(-26.175081861218,-90.6434116538366,10.));
#28472=CARTESIAN_POINT('Ctrl Pts',(-26.1204874224643,-90.577523210881,10.));
#28473=CARTESIAN_POINT('Ctrl Pts',(-26.0743569854985,-90.5218497259268,
10.));
#28474=CARTESIAN_POINT('Ctrl Pts',(-26.0257311604375,-90.4682919003903,
10.));
#28475=CARTESIAN_POINT('Ctrl Pts',(-25.9746123907308,-90.41708711057,10.));
#28476=CARTESIAN_POINT('Ctrl Pts',(-25.9557806038368,-90.3982236344852,
10.));
#28477=CARTESIAN_POINT('Ctrl Pts',(-25.9366103467742,-90.3796797449892,
10.));
#28478=CARTESIAN_POINT('Ctrl Pts',(-25.9171117712833,-90.3614597429256,
10.));
#28479=CARTESIAN_POINT('Origin',(-24.,-92.,5.));
#28480=CARTESIAN_POINT('Origin',(-24.,92.,1.));
#28481=CARTESIAN_POINT('Ctrl Pts',(-25.913465996665,93.635987203375,0.999999999999996));
#28482=CARTESIAN_POINT('Ctrl Pts',(-25.9756063047027,93.5775905725192,0.999999999999996));
#28483=CARTESIAN_POINT('Ctrl Pts',(-26.0343713138183,93.5159402490042,0.999999999999997));
#28484=CARTESIAN_POINT('Ctrl Pts',(-26.0897489850044,93.4514126613341,0.999999999999999));
#28485=CARTESIAN_POINT('Ctrl Pts',(-26.1464813764581,93.3853065162965,1.));
#28486=CARTESIAN_POINT('Ctrl Pts',(-26.1996591402971,93.3161801193224,1.));
#28487=CARTESIAN_POINT('Ctrl Pts',(-26.2492404445134,93.2443919311744,1.));
#28488=CARTESIAN_POINT('Ctrl Pts',(-26.2621841917353,93.2256508315686,1.));
#28489=CARTESIAN_POINT('Ctrl Pts',(-26.274882658945,93.2067281064287,1.));
#28490=CARTESIAN_POINT('Ctrl Pts',(-26.2873347259162,93.1876296997784,1.));
#28491=CARTESIAN_POINT('Ctrl Pts',(-26.2974956811164,93.1720452948103,1.));
#28492=CARTESIAN_POINT('Ctrl Pts',(-26.3074930000883,93.1563430141694,1.));
#28493=CARTESIAN_POINT('Ctrl Pts',(-26.3173172475083,93.1405406478853,1.));
#28494=CARTESIAN_POINT('Ctrl Pts',(-26.3647645432756,93.0642213620562,1.));
#28495=CARTESIAN_POINT('Ctrl Pts',(-26.4082282644583,92.985494853327,1.));
#28496=CARTESIAN_POINT('Ctrl Pts',(-26.4476736593442,92.9047536082207,1.));
#28497=CARTESIAN_POINT('Ctrl Pts',(-26.4795145181984,92.8395781778169,1.));
#28498=CARTESIAN_POINT('Ctrl Pts',(-26.5087365606955,92.7730888691482,1.));
#28499=CARTESIAN_POINT('Ctrl Pts',(-26.5353043305085,92.7054742951973,1.));
#28500=CARTESIAN_POINT('Ctrl Pts',(-26.546029034718,92.6781800845433,1.));
#28501=CARTESIAN_POINT('Ctrl Pts',(-26.5563210321205,92.650702354303,1.));
#28502=CARTESIAN_POINT('Ctrl Pts',(-26.5661772000867,92.6230529446547,1.));
#28503=CARTESIAN_POINT('Ctrl Pts',(-26.5713953802244,92.6084144359825,1.));
#28504=CARTESIAN_POINT('Ctrl Pts',(-26.5764908406454,92.5937291337602,0.999999999999998));
#28505=CARTESIAN_POINT('Ctrl Pts',(-26.5814593611535,92.5790106126507,0.999999999999999));
#28506=CARTESIAN_POINT('Ctrl Pts',(-26.6109734289791,92.4915794689899,1.));
#28507=CARTESIAN_POINT('Ctrl Pts',(-26.6360512213471,92.4028684426336,1.));
#28508=CARTESIAN_POINT('Ctrl Pts',(-26.6566599711623,92.3132752268106,1.));
#28509=CARTESIAN_POINT('Ctrl Pts',(-26.6775876501422,92.2222955178845,1.));
#28510=CARTESIAN_POINT('Ctrl Pts',(-26.6939073958785,92.1304052976179,1.));
#28511=CARTESIAN_POINT('Ctrl Pts',(-26.7055430518716,92.0379878724461,1.));
#28512=CARTESIAN_POINT('Ctrl Pts',(-26.7170875469971,91.9462945020825,1.00000000000001));
#28513=CARTESIAN_POINT('Ctrl Pts',(-26.7240214047279,91.854081225586,1.00000000000001));
#28514=CARTESIAN_POINT('Ctrl Pts',(-26.7262232901922,91.7617032514415,1.00000000000001));
#28515=CARTESIAN_POINT('Ctrl Pts',(-26.7273184961007,91.7157549472591,1.00000000000001));
#28516=CARTESIAN_POINT('Ctrl Pts',(-26.7272422423285,91.6697656845161,1.00000000000001));
#28517=CARTESIAN_POINT('Ctrl Pts',(-26.72597480777,91.6237784805461,1.00000000000001));
#28518=CARTESIAN_POINT('Ctrl Pts',(-26.7255580393425,91.6086565836768,1.00000000000001));
#28519=CARTESIAN_POINT('Ctrl Pts',(-26.7250123597643,91.5935330587279,1.));
#28520=CARTESIAN_POINT('Ctrl Pts',(-26.7243372523629,91.5784152587756,1.));
#28521=CARTESIAN_POINT('Ctrl Pts',(-26.7200633703958,91.4827094607578,1.));
#28522=CARTESIAN_POINT('Ctrl Pts',(-26.7106224530131,91.3875708354282,1.00000000000001));
#28523=CARTESIAN_POINT('Ctrl Pts',(-26.6959503279345,91.2933977109171,1.00000000000001));
#28524=CARTESIAN_POINT('Ctrl Pts',(-26.6917956796564,91.2667310755459,1.00000000000001));
#28525=CARTESIAN_POINT('Ctrl Pts',(-26.6872212841807,91.2401417271289,1.00000000000001));
#28526=CARTESIAN_POINT('Ctrl Pts',(-26.6822249702578,91.2136384506289,1.));
#28527=CARTESIAN_POINT('Ctrl Pts',(-26.6652600471296,91.1236468977731,1.));
#28528=CARTESIAN_POINT('Ctrl Pts',(-26.6434348327882,91.0346478147219,1.));
#28529=CARTESIAN_POINT('Ctrl Pts',(-26.6170519644759,90.9468734390352,1.));
#28530=CARTESIAN_POINT('Ctrl Pts',(-26.5900726212499,90.8571146235775,1.));
#28531=CARTESIAN_POINT('Ctrl Pts',(-26.5583270022612,90.7686358185392,1.00000000000001));
#28532=CARTESIAN_POINT('Ctrl Pts',(-26.5220844975705,90.6816890800664,1.00000000000001));
#28533=CARTESIAN_POINT('Ctrl Pts',(-26.5094176334725,90.6513009341755,1.00000000000001));
#28534=CARTESIAN_POINT('Ctrl Pts',(-26.4962010035771,90.6211000168169,1.));
#28535=CARTESIAN_POINT('Ctrl Pts',(-26.4824446757821,90.5910974447628,1.));
#28536=CARTESIAN_POINT('Ctrl Pts',(-26.4754977538534,90.5759461973644,1.));
#28537=CARTESIAN_POINT('Ctrl Pts',(-26.4684131851587,90.5608455364142,1.));
#28538=CARTESIAN_POINT('Ctrl Pts',(-26.4611921989836,90.545796919332,1.));
#28539=CARTESIAN_POINT('Ctrl Pts',(-26.455182228529,90.5332720727456,1.));
#28540=CARTESIAN_POINT('Ctrl Pts',(-26.4490796038181,90.5207872118101,1.));
#28541=CARTESIAN_POINT('Ctrl Pts',(-26.4428889235851,90.5083503619119,1.));
#28542=CARTESIAN_POINT('Ctrl Pts',(-26.3999256383549,90.4220386951104,1.));
#28543=CARTESIAN_POINT('Ctrl Pts',(-26.352675311748,90.3379337033055,1.));
#28544=CARTESIAN_POINT('Ctrl Pts',(-26.3014800112192,90.2562854651096,1.));
#28545=CARTESIAN_POINT('Ctrl Pts',(-26.2492799088519,90.1730347302195,1.));
#28546=CARTESIAN_POINT('Ctrl Pts',(-26.1929781409368,90.0923373579129,1.));
#28547=CARTESIAN_POINT('Ctrl Pts',(-26.1328823971401,90.014465764712,1.));
#28548=CARTESIAN_POINT('Ctrl Pts',(-26.0723186336165,89.935987715222,1.));
#28549=CARTESIAN_POINT('Ctrl Pts',(-26.0079011072123,89.8603787928957,1.));
#28550=CARTESIAN_POINT('Ctrl Pts',(-25.9398956031168,89.787937415356,1.));
#28551=CARTESIAN_POINT('Ctrl Pts',(-25.9029689988626,89.7486021568998,1.));
#28552=CARTESIAN_POINT('Ctrl Pts',(-25.8649836968098,89.7102012386594,0.999999999999998));
#28553=CARTESIAN_POINT('Ctrl Pts',(-25.8259770082825,89.6727861936411,0.999999999999997));
#28554=CARTESIAN_POINT('Ctrl Pts',(-25.8138450071499,89.6611492312207,0.999999999999997));
#28555=CARTESIAN_POINT('Ctrl Pts',(-25.8016141768636,89.6496076606791,1.));
#28556=CARTESIAN_POINT('Ctrl Pts',(-25.789285575206,89.6381630971647,1.));
#28557=CARTESIAN_POINT('Ctrl Pts',(-25.7779997494658,89.6276865359874,1.));
#28558=CARTESIAN_POINT('Ctrl Pts',(-25.7666377256336,89.6172966286238,1.));
#28559=CARTESIAN_POINT('Ctrl Pts',(-25.7552049288473,89.6069982204744,1.));
#28560=CARTESIAN_POINT('Ctrl Pts',(-25.679395860332,89.5387111037176,1.));
#28561=CARTESIAN_POINT('Ctrl Pts',(-25.600420502922,89.4743910090163,1.));
#28562=CARTESIAN_POINT('Ctrl Pts',(-25.5186050207122,89.4143205615864,1.));
#28563=CARTESIAN_POINT('Ctrl Pts',(-25.4367186080971,89.3541980357348,1.));
#28564=CARTESIAN_POINT('Ctrl Pts',(-25.3519865671594,89.2983316916956,1.));
#28565=CARTESIAN_POINT('Ctrl Pts',(-25.2646909477799,89.2470310937083,1.));
#28566=CARTESIAN_POINT('Ctrl Pts',(-25.1791591002471,89.1967670030634,1.));
#28567=CARTESIAN_POINT('Ctrl Pts',(-25.091165555463,89.1508853502904,1.));
#28568=CARTESIAN_POINT('Ctrl Pts',(-25.0009418604243,89.1097134462671,1.));
#28569=CARTESIAN_POINT('Ctrl Pts',(-24.9631524549254,89.0924689543891,1.));
#28570=CARTESIAN_POINT('Ctrl Pts',(-24.9249714626436,89.0760511834599,1.));
#28571=CARTESIAN_POINT('Ctrl Pts',(-24.8864145036881,89.0604865582877,1.));
#28572=CARTESIAN_POINT('Ctrl Pts',(-24.8564008056108,89.0483706660271,1.));
#28573=CARTESIAN_POINT('Ctrl Pts',(-24.8261592741353,89.0367717663531,1.));
#28574=CARTESIAN_POINT('Ctrl Pts',(-24.7957016814435,89.0256872793281,1.));
#28575=CARTESIAN_POINT('Ctrl Pts',(-23.2062007174672,89.0307770462543,0.999999999999999));
#28576=CARTESIAN_POINT('Ctrl Pts',(-23.1113643609077,89.065468609115,0.999999999999999));
#28577=CARTESIAN_POINT('Ctrl Pts',(-23.018571234946,89.1051505773298,0.999999999999999));
#28578=CARTESIAN_POINT('Ctrl Pts',(-22.9280622736109,89.1495027068318,1.));
#28579=CARTESIAN_POINT('Ctrl Pts',(-22.836281839029,89.1944778966946,1.));
#28580=CARTESIAN_POINT('Ctrl Pts',(-22.7468495274982,89.2442560843952,0.999999999999997));
#28581=CARTESIAN_POINT('Ctrl Pts',(-22.6600505960784,89.2985440193305,0.999999999999997));
#28582=CARTESIAN_POINT('Ctrl Pts',(-22.6355418278746,89.3138728994427,0.999999999999996));
#28583=CARTESIAN_POINT('Ctrl Pts',(-22.6112432552978,89.3295615450764,1.));
#28584=CARTESIAN_POINT('Ctrl Pts',(-22.5871618961201,89.3456038099341,1.));
#28585=CARTESIAN_POINT('Ctrl Pts',(-22.5678312416192,89.3584813006558,1.));
#28586=CARTESIAN_POINT('Ctrl Pts',(-22.5486384464619,89.3715882773608,0.999999999999998));
#28587=CARTESIAN_POINT('Ctrl Pts',(-22.5296064292129,89.3849077949563,0.999999999999998));
#28588=CARTESIAN_POINT('Ctrl Pts',(-22.446898789183,89.4427905644099,1.));
#28589=CARTESIAN_POINT('Ctrl Pts',(-22.3671459828654,89.5047351114195,0.999999999999997));
#28590=CARTESIAN_POINT('Ctrl Pts',(-22.2906143664206,89.5704442021524,0.999999999999998));
#28591=CARTESIAN_POINT('Ctrl Pts',(-22.2316015136182,89.6211119010635,0.999999999999999));
#28592=CARTESIAN_POINT('Ctrl Pts',(-22.1745045554968,89.6740188394976,0.999999999999999));
#28593=CARTESIAN_POINT('Ctrl Pts',(-22.1194631966057,89.7290405250296,1.));
#28594=CARTESIAN_POINT('Ctrl Pts',(-22.0901430624395,89.7583501793395,1.));
#28595=CARTESIAN_POINT('Ctrl Pts',(-22.0614065053773,89.7882600668129,1.));
#28596=CARTESIAN_POINT('Ctrl Pts',(-22.0332766723516,89.8187522038962,1.));
#28597=CARTESIAN_POINT('Ctrl Pts',(-22.0236426842444,89.8291952408583,1.));
#28598=CARTESIAN_POINT('Ctrl Pts',(-22.014080660821,89.8397057922762,1.));
#28599=CARTESIAN_POINT('Ctrl Pts',(-22.0045980888106,89.8502756076143,1.));
#28600=CARTESIAN_POINT('Ctrl Pts',(-21.9388055958393,89.9236116709296,1.));
#28601=CARTESIAN_POINT('Ctrl Pts',(-21.8767453524491,89.9998940820391,1.));
#28602=CARTESIAN_POINT('Ctrl Pts',(-21.8186611502822,90.0788444257391,1.));
#28603=CARTESIAN_POINT('Ctrl Pts',(-21.7610833540022,90.157106442539,1.));
#28604=CARTESIAN_POINT('Ctrl Pts',(-21.7074121340599,90.2379908580803,1.));
#28605=CARTESIAN_POINT('Ctrl Pts',(-21.6579307654416,90.3212488810837,1.));
#28606=CARTESIAN_POINT('Ctrl Pts',(-21.6098823874139,90.4020957346531,1.));
#28607=CARTESIAN_POINT('Ctrl Pts',(-21.5657844914906,90.4851814058657,1.));
#28608=CARTESIAN_POINT('Ctrl Pts',(-21.5259442417593,90.5702884177283,1.));
#28609=CARTESIAN_POINT('Ctrl Pts',(-21.5051329728217,90.6147455916742,1.));
#28610=CARTESIAN_POINT('Ctrl Pts',(-21.4854842990003,90.659754434822,1.));
#28611=CARTESIAN_POINT('Ctrl Pts',(-21.4670477073908,90.7052841842656,1.));
#28612=CARTESIAN_POINT('Ctrl Pts',(-21.4599070329778,90.7229183068716,1.));
#28613=CARTESIAN_POINT('Ctrl Pts',(-21.452948225379,90.7406305688681,1.));
#28614=CARTESIAN_POINT('Ctrl Pts',(-21.4461743283707,90.7584191738098,1.));
#28615=CARTESIAN_POINT('Ctrl Pts',(-21.441020443057,90.7719535440028,1.));
#28616=CARTESIAN_POINT('Ctrl Pts',(-21.4359736403243,90.7855322279792,1.));
#28617=CARTESIAN_POINT('Ctrl Pts',(-21.4310400911309,90.7991405304999,1.));
#28618=CARTESIAN_POINT('Ctrl Pts',(-21.3993682454182,90.8865015845694,1.));
#28619=CARTESIAN_POINT('Ctrl Pts',(-21.372305110326,90.975223579926,1.));
#28620=CARTESIAN_POINT('Ctrl Pts',(-21.3501019716912,91.0650831130208,1.));
#28621=CARTESIAN_POINT('Ctrl Pts',(-21.3450993725627,91.085329404743,1.));
#28622=CARTESIAN_POINT('Ctrl Pts',(-21.3403436950143,91.1056334832557,1.));
#28623=CARTESIAN_POINT('Ctrl Pts',(-21.3358381789014,91.1259928495363,1.));
#28624=CARTESIAN_POINT('Ctrl Pts',(-21.3154926547754,91.21792948176,1.));
#28625=CARTESIAN_POINT('Ctrl Pts',(-21.3002441342106,91.3109938333365,1.));
#28626=CARTESIAN_POINT('Ctrl Pts',(-21.2899827069894,91.4047941591649,1.));
#28627=CARTESIAN_POINT('Ctrl Pts',(-21.2792695744501,91.5027235505803,1.));
#28628=CARTESIAN_POINT('Ctrl Pts',(-21.2739922714095,91.6014563765819,0.999999999999999));
#28629=CARTESIAN_POINT('Ctrl Pts',(-21.2740832157028,91.7005321536462,0.999999999999999));
#28630=CARTESIAN_POINT('Ctrl Pts',(-21.2741183389869,91.7387958702903,0.999999999999999));
#28631=CARTESIAN_POINT('Ctrl Pts',(-21.2749547528149,91.7771104872721,0.999999999999999));
#28632=CARTESIAN_POINT('Ctrl Pts',(-21.2765906985084,91.8154482999678,0.999999999999999));
#28633=CARTESIAN_POINT('Ctrl Pts',(-21.277178303569,91.8292186181647,0.999999999999999));
#28634=CARTESIAN_POINT('Ctrl Pts',(-21.2778690508016,91.8429901308369,0.999999999999999));
#28635=CARTESIAN_POINT('Ctrl Pts',(-21.2786619686978,91.8567498857155,0.999999999999999));
#28636=CARTESIAN_POINT('Ctrl Pts',(-21.2840135874423,91.9496182173293,1.));
#28637=CARTESIAN_POINT('Ctrl Pts',(-21.2940209180043,92.0420994637286,1.));
#28638=CARTESIAN_POINT('Ctrl Pts',(-21.3085609026778,92.1338217237554,1.));
#28639=CARTESIAN_POINT('Ctrl Pts',(-21.3230638385398,92.2253102695935,1.));
#28640=CARTESIAN_POINT('Ctrl Pts',(-21.3420767703985,92.3160446363129,0.999999999999998));
#28641=CARTESIAN_POINT('Ctrl Pts',(-21.3655261680114,92.4056386468098,0.999999999999998));
#28642=CARTESIAN_POINT('Ctrl Pts',(-21.3885742626337,92.4936993836192,0.999999999999998));
#28643=CARTESIAN_POINT('Ctrl Pts',(-21.4159087427557,92.5806592446602,0.999999999999998));
#28644=CARTESIAN_POINT('Ctrl Pts',(-21.4475001239804,92.6661223199064,0.999999999999998));
#28645=CARTESIAN_POINT('Ctrl Pts',(-21.4633626089743,92.7090345540687,0.999999999999998));
#28646=CARTESIAN_POINT('Ctrl Pts',(-21.4802989345861,92.7515688848743,0.999999999999994));
#28647=CARTESIAN_POINT('Ctrl Pts',(-21.4983087570456,92.7936714133834,0.999999999999994));
#28648=CARTESIAN_POINT('Ctrl Pts',(-21.5036080709844,92.8060599039801,0.999999999999994));
#28649=CARTESIAN_POINT('Ctrl Pts',(-21.5090003429253,92.8184109900054,0.999999999999999));
#28650=CARTESIAN_POINT('Ctrl Pts',(-21.5144855985927,92.8307232495397,0.999999999999999));
#28651=CARTESIAN_POINT('Ctrl Pts',(-21.5200790278412,92.8432783165719,0.999999999999999));
#28652=CARTESIAN_POINT('Ctrl Pts',(-21.5257654643176,92.8557847221215,0.999999999999994));
#28653=CARTESIAN_POINT('Ctrl Pts',(-21.5315436189536,92.8682391310481,0.999999999999995));
#28654=CARTESIAN_POINT('Ctrl Pts',(-21.5690290041703,92.9490362619096,0.999999999999995));
#28655=CARTESIAN_POINT('Ctrl Pts',(-21.6103840907841,93.0276765322135,1.));
#28656=CARTESIAN_POINT('Ctrl Pts',(-21.6555390550696,93.1038122346988,1.));
#28657=CARTESIAN_POINT('Ctrl Pts',(-21.6999358276416,93.1786695515261,1.));
#28658=CARTESIAN_POINT('Ctrl Pts',(-21.7480063970068,93.251106371718,0.999999999999998));
#28659=CARTESIAN_POINT('Ctrl Pts',(-21.7997205984681,93.3207580281866,0.999999999999998));
#28660=CARTESIAN_POINT('Ctrl Pts',(-21.8498548445433,93.3882817100044,0.999999999999997));
#28661=CARTESIAN_POINT('Ctrl Pts',(-21.9034139287086,93.4531882520499,0.999999999999996));
#28662=CARTESIAN_POINT('Ctrl Pts',(-21.960398059015,93.5151051166907,0.999999999999996));
#28663=CARTESIAN_POINT('Ctrl Pts',(-21.9815871896649,93.5381284484017,0.999999999999995));
#28664=CARTESIAN_POINT('Ctrl Pts',(-22.0032501397421,93.5607379645122,0.999999999999999));
#28665=CARTESIAN_POINT('Ctrl Pts',(-22.0253877587029,93.5829128445691,0.999999999999999));
#28666=CARTESIAN_POINT('Ctrl Pts',(-22.0442145502047,93.6017713245233,0.999999999999999));
#28667=CARTESIAN_POINT('Ctrl Pts',(-22.0633846686702,93.6203154277105,0.999999999999998));
#28668=CARTESIAN_POINT('Ctrl Pts',(-22.0828883826538,93.638540237813,0.999999999999998));
#28669=CARTESIAN_POINT('Origin',(-24.,92.,12.2084234471775));
#28670=CARTESIAN_POINT('Ctrl Pts',(-27.076766805402,92.0019372679896,9.70842344717746));
#28671=CARTESIAN_POINT('Ctrl Pts',(-27.0777009893786,92.1261018275903,9.70197366100994));
#28672=CARTESIAN_POINT('Ctrl Pts',(-27.0146667615987,93.2631137100916,9.64286281975954));
#28673=CARTESIAN_POINT('Ctrl Pts',(-25.5990316467514,95.2555126958587,9.53109092342626));
#28674=CARTESIAN_POINT('Ctrl Pts',(-22.1476051047098,95.1179530605298,9.37310775817762));
#28675=CARTESIAN_POINT('Ctrl Pts',(-20.3764282219686,92.1527149914235,9.215124592929));
#28676=CARTESIAN_POINT('Ctrl Pts',(-21.8919231533181,89.0487577497888,9.05714142768035));
#28677=CARTESIAN_POINT('Ctrl Pts',(-25.3195311476576,88.6217766146216,8.89915826243172));
#28678=CARTESIAN_POINT('Ctrl Pts',(-26.9608439554881,90.5621019356809,8.78291893559742));
#28679=CARTESIAN_POINT('Ctrl Pts',(-27.0762792831289,91.7866862376245,8.719340663846));
#28680=CARTESIAN_POINT('Ctrl Pts',(-27.0743674416594,91.9973209105276,8.70842344717745));
#28681=CARTESIAN_POINT('Ctrl Pts',(-27.0702888275776,91.9968971804148,9.79157655282255));
#28682=CARTESIAN_POINT('Ctrl Pts',(-27.0652853128242,92.6903808619892,9.75572892504928));
#28683=CARTESIAN_POINT('Ctrl Pts',(-26.4922439119073,94.4123573994235,9.66722024219312));
#28684=CARTESIAN_POINT('Ctrl Pts',(-23.6460838986402,95.6088399383518,9.5260505042541));
#28685=CARTESIAN_POINT('Ctrl Pts',(-20.7843955634607,93.6770749374766,9.36806733900546));
#28686=CARTESIAN_POINT('Ctrl Pts',(-20.8381773234134,90.2228835564638,9.21008417375683));
#28687=CARTESIAN_POINT('Ctrl Pts',(-23.760424197283,88.3812153351417,9.05210100850819));
#28688=CARTESIAN_POINT('Ctrl Pts',(-26.5324622678489,89.6531111499585,8.91259846819677));
#28689=CARTESIAN_POINT('Ctrl Pts',(-27.0660796534741,91.3404823888654,8.82575698296822));
#28690=CARTESIAN_POINT('Ctrl Pts',(-27.0703857423214,92.0021357609841,8.79157655282255));
#28691=CARTESIAN_POINT('Ctrl Pts',(-22.0865340033349,93.6359872033749,10.));
#28692=CARTESIAN_POINT('Ctrl Pts',(-21.5452199193478,93.0028611672492,9.94733894491712));
#28693=CARTESIAN_POINT('Ctrl Pts',(-21.1498718103827,91.167401053521,9.84201683475137));
#28694=CARTESIAN_POINT('Ctrl Pts',(-23.1420133042203,89.1541928650905,9.68403366950274));
#28695=CARTESIAN_POINT('Ctrl Pts',(-25.9132996010903,89.7281648944129,9.52605050425409));
#28696=CARTESIAN_POINT('Ctrl Pts',(-26.9487151037096,92.3598882319117,9.36806733900546));
#28697=CARTESIAN_POINT('Ctrl Pts',(-25.3097648188374,94.6665863711807,9.21008417375683));
#28698=CARTESIAN_POINT('Ctrl Pts',(-22.4827056616583,94.5539114461962,9.05210100850819));
#28699=CARTESIAN_POINT('Ctrl Pts',(-21.0319368956584,92.1250886581775,8.89411784325956));
#28700=CARTESIAN_POINT('Ctrl Pts',(-22.2732768955518,89.5826411697067,8.73613467801092));
#28701=CARTESIAN_POINT('Ctrl Pts',(-25.0808263101441,89.2329014567464,8.57815151276229));
#28702=CARTESIAN_POINT('Ctrl Pts',(-26.9080231896089,91.3929749996272,8.42016834751365));
#28703=CARTESIAN_POINT('Ctrl Pts',(-26.0975468057329,94.1036603137053,8.26218518226502));
#28704=CARTESIAN_POINT('Ctrl Pts',(-23.3845223931579,94.9062444322857,8.10420201701639));
#28705=CARTESIAN_POINT('Ctrl Pts',(-21.2297579033362,93.0727703008244,7.94621885176775));
#28706=CARTESIAN_POINT('Ctrl Pts',(-21.5876971940873,90.2662546152948,7.78823568651912));
#28707=CARTESIAN_POINT('Ctrl Pts',(-24.1336776409024,89.0323062843058,7.63025252127048));
#28708=CARTESIAN_POINT('Ctrl Pts',(-26.5584078194921,90.4901569016087,7.47226935602185));
#28709=CARTESIAN_POINT('Ctrl Pts',(-26.6625748235914,93.3174870105019,7.31428619077321));
#28710=CARTESIAN_POINT('Ctrl Pts',(-24.3516955628713,94.9498113013859,7.15630302552459));
#28711=CARTESIAN_POINT('Ctrl Pts',(-21.7218164325105,93.9065561225942,6.99831986027594));
#28712=CARTESIAN_POINT('Ctrl Pts',(-21.1583275522511,91.1339894343907,6.84033669502731));
#28713=CARTESIAN_POINT('Ctrl Pts',(-23.1723325768719,89.1469239033541,6.68235352977868));
#28714=CARTESIAN_POINT('Ctrl Pts',(-25.9370602031581,89.7476957660557,6.52437036453004));
#28715=CARTESIAN_POINT('Ctrl Pts',(-26.9448081097383,92.3913844486005,6.36638719928141));
#28716=CARTESIAN_POINT('Ctrl Pts',(-25.2815145478907,94.6800740756701,6.20840403403277));
#28717=CARTESIAN_POINT('Ctrl Pts',(-22.4558435504054,94.5378450403174,6.05042086878414));
#28718=CARTESIAN_POINT('Ctrl Pts',(-21.0307751580051,92.0937039308721,5.8924377035355));
#28719=CARTESIAN_POINT('Ctrl Pts',(-22.2988950433351,89.5645701580226,5.73445453828688));
#28720=CARTESIAN_POINT('Ctrl Pts',(-25.1099751867048,89.244454378182,5.57647137303823));
#28721=CARTESIAN_POINT('Ctrl Pts',(-26.9142699499045,91.4237125300643,5.4184882077896));
#28722=CARTESIAN_POINT('Ctrl Pts',(-26.0752223982648,94.1256830870714,5.26050504254097));
#28723=CARTESIAN_POINT('Ctrl Pts',(-23.3538772995946,94.8995865300144,5.10252187729233));
#28724=CARTESIAN_POINT('Ctrl Pts',(-21.2185875437792,93.0434660210873,4.9445387120437));
#28725=CARTESIAN_POINT('Ctrl Pts',(-21.606133821254,90.2408862153809,4.78655554679506));
#28726=CARTESIAN_POINT('Ctrl Pts',(-24.1649984307827,89.0338826544914,4.62857238154643));
#28727=CARTESIAN_POINT('Ctrl Pts',(-26.5742038315408,90.5172487662401,4.47058921629779));
#28728=CARTESIAN_POINT('Ctrl Pts',(-26.6485184946104,93.3455208558374,4.31260605104916));
#28729=CARTESIAN_POINT('Ctrl Pts',(-24.3205364822007,94.9533596050058,4.15462288580052));
#28730=CARTESIAN_POINT('Ctrl Pts',(-21.7018169423985,93.8824003852299,3.99663972055189));
#28731=CARTESIAN_POINT('Ctrl Pts',(-21.1676278725257,91.1040397712239,3.83865655530325));
#28732=CARTESIAN_POINT('Ctrl Pts',(-23.2024970078836,89.1383456544602,3.68067339005462));
#28733=CARTESIAN_POINT('Ctrl Pts',(-25.9607285557694,89.768269726576,3.52269022480599));
#28734=CARTESIAN_POINT('Ctrl Pts',(-26.9405124242392,92.4224492832981,3.36470705955735));
#28735=CARTESIAN_POINT('Ctrl Pts',(-25.2531510669841,94.6934530172095,3.20672389430872));
#28736=CARTESIAN_POINT('Ctrl Pts',(-22.4291391049686,94.5214027346518,3.04874072906009));
#28737=CARTESIAN_POINT('Ctrl Pts',(-21.029951212319,92.0623545122335,2.89075756381144));
#28738=CARTESIAN_POINT('Ctrl Pts',(-22.3246997187609,89.5467477993204,2.73277439856282));
#28739=CARTESIAN_POINT('Ctrl Pts',(-25.1390011801809,89.2563262409203,2.57479123331418));
#28740=CARTESIAN_POINT('Ctrl Pts',(-26.9201929246498,91.4545070114807,2.41680806806554));
#28741=CARTESIAN_POINT('Ctrl Pts',(-26.0526634178927,94.1474755214498,2.25882490281691));
#28742=CARTESIAN_POINT('Ctrl Pts',(-23.3233115994341,94.892596181515,2.10084173756827));
#28743=CARTESIAN_POINT('Ctrl Pts',(-21.2077117493853,93.0140624829425,1.94285857231964));
#28744=CARTESIAN_POINT('Ctrl Pts',(-21.6248688237331,90.215680056917,1.78487540707101));
#28745=CARTESIAN_POINT('Ctrl Pts',(-24.1962362281276,89.0358581128856,1.62689224182237));
#28746=CARTESIAN_POINT('Ctrl Pts',(-26.5898449391916,90.5443661358105,1.46890907657374));
#28747=CARTESIAN_POINT('Ctrl Pts',(-26.6338974915197,93.3736900328969,1.31092591132511));
#28748=CARTESIAN_POINT('Ctrl Pts',(-24.2898922274084,94.9559960431297,1.15294274607647));
#28749=CARTESIAN_POINT('Ctrl Pts',(-21.6809482123999,93.8592359252299,0.994959580827835));
#28750=CARTESIAN_POINT('Ctrl Pts',(-21.1795852070609,91.0717155076706,0.836976415579202));
#28751=CARTESIAN_POINT('Ctrl Pts',(-22.5450731455404,89.7830508320407,0.731654305413445));
#28752=CARTESIAN_POINT('Ctrl Pts',(-23.3498000020249,89.5679131979649,0.678993250330566));
#28753=CARTESIAN_POINT('Ctrl Pts',(-21.9456684496579,93.7564253212268,10.1070022498898));
#28754=CARTESIAN_POINT('Ctrl Pts',(-21.3645039014938,93.0766898079629,10.0543411948069));
#28755=CARTESIAN_POINT('Ctrl Pts',(-20.9400510525638,91.106106778216,9.94901908464118));
#28756=CARTESIAN_POINT('Ctrl Pts',(-23.0788500334022,88.9446902147085,9.79103591939254));
#28757=CARTESIAN_POINT('Ctrl Pts',(-26.0541529050567,89.5609169210655,9.63305275414391));
#28758=CARTESIAN_POINT('Ctrl Pts',(-27.1657936336882,92.3863824863894,9.47506958889527));
#28759=CARTESIAN_POINT('Ctrl Pts',(-25.4061870948087,94.8628951460734,9.31708642364664));
#28760=CARTESIAN_POINT('Ctrl Pts',(-22.3710054760088,94.7419253176408,9.159103258398));
#28761=CARTESIAN_POINT('Ctrl Pts',(-20.8134340044285,92.134297435926,9.00112009314937));
#28762=CARTESIAN_POINT('Ctrl Pts',(-22.1461589814739,89.4046800297342,8.84313692790073));
#28763=CARTESIAN_POINT('Ctrl Pts',(-25.1603945893153,89.0291931760381,8.6851537626521));
#28764=CARTESIAN_POINT('Ctrl Pts',(-27.1221060619588,91.3482870287292,8.52717059740346));
#28765=CARTESIAN_POINT('Ctrl Pts',(-26.2519640217524,94.2585275939991,8.36918743215483));
#28766=CARTESIAN_POINT('Ctrl Pts',(-23.3392121582153,95.1201963560661,8.2112042669062));
#28767=CARTESIAN_POINT('Ctrl Pts',(-21.0258182004901,93.1517455126427,8.05322110165756));
#28768=CARTESIAN_POINT('Ctrl Pts',(-21.4101082685543,90.1386197349378,7.89523793640893));
#28769=CARTESIAN_POINT('Ctrl Pts',(-24.1435187224439,88.813830586732,7.73725477116029));
#28770=CARTESIAN_POINT('Ctrl Pts',(-26.7467527049787,90.3790052613962,7.57927160591167));
#28771=CARTESIAN_POINT('Ctrl Pts',(-26.8585882763444,93.4144777788355,7.42128844066302));
#28772=CARTESIAN_POINT('Ctrl Pts',(-24.3775866893799,95.1669705312529,7.2633052754144));
#28773=CARTESIAN_POINT('Ctrl Pts',(-21.5541010980485,94.0469129851116,7.10532211016575));
#28774=CARTESIAN_POINT('Ctrl Pts',(-20.9491292892987,91.0702354622651,6.94733894491712));
#28775=CARTESIAN_POINT('Ctrl Pts',(-23.1114013504886,88.936886126494,6.78935577966849));
#28776=CARTESIAN_POINT('Ctrl Pts',(-26.0796627153006,89.5818856165591,6.63137261441985));
#28777=CARTESIAN_POINT('Ctrl Pts',(-27.1615990146061,92.4201973917876,6.47338944917122));
#28778=CARTESIAN_POINT('Ctrl Pts',(-25.3758570952097,94.8773757884901,6.31540628392258));
#28779=CARTESIAN_POINT('Ctrl Pts',(-22.342165829654,94.7246761349771,6.15742311867395));
#28780=CARTESIAN_POINT('Ctrl Pts',(-20.8121867419641,92.1006022275374,5.99943995342532));
#28781=CARTESIAN_POINT('Ctrl Pts',(-22.1736630862473,89.3852786661803,5.84145678817668));
#28782=CARTESIAN_POINT('Ctrl Pts',(-25.1916893480828,89.0415966005281,5.68347362292805));
#28783=CARTESIAN_POINT('Ctrl Pts',(-27.1288126962993,91.381287394906,5.52549045767941));
#28784=CARTESIAN_POINT('Ctrl Pts',(-26.2279961358928,94.2821716400552,5.36750729243078));
#28785=CARTESIAN_POINT('Ctrl Pts',(-23.3063110339308,95.113048312297,5.20952412718214));
#28786=CARTESIAN_POINT('Ctrl Pts',(-21.0138255013219,93.1202839102265,5.05154096193351));
#28787=CARTESIAN_POINT('Ctrl Pts',(-21.4299021634741,90.1113837639743,4.89355779668487));
#28788=CARTESIAN_POINT('Ctrl Pts',(-24.1771452864616,88.8155230061493,4.73557463143624));
#28789=CARTESIAN_POINT('Ctrl Pts',(-26.7637115879574,90.4080915751154,4.5775914661876));
#28790=CARTESIAN_POINT('Ctrl Pts',(-26.843497148434,93.4445754200009,4.41960830093897));
#28791=CARTESIAN_POINT('Ctrl Pts',(-24.3441337392816,95.1707800539146,4.26162513569034));
#28792=CARTESIAN_POINT('Ctrl Pts',(-21.5326292853278,94.0209789504981,4.1036419704417));
#28793=CARTESIAN_POINT('Ctrl Pts',(-20.9591142806189,91.0380809645771,3.94565880519306));
#28794=CARTESIAN_POINT('Ctrl Pts',(-23.1437864268023,88.9276763640108,3.78767563994443));
#28795=CARTESIAN_POINT('Ctrl Pts',(-26.1050734848668,89.6039741910547,3.6296924746958));
#28796=CARTESIAN_POINT('Ctrl Pts',(-27.1569870893008,92.4535491577125,3.47170930944716));
#28797=CARTESIAN_POINT('Ctrl Pts',(-25.3454055513592,94.891739661045,3.31372614419853));
#28798=CARTESIAN_POINT('Ctrl Pts',(-22.3134954561587,94.7070233795333,3.1557429789499));
#28799=CARTESIAN_POINT('Ctrl Pts',(-20.8113021390385,92.0669449271691,2.99775981370126));
#28800=CARTESIAN_POINT('Ctrl Pts',(-22.2013674504565,89.3661442609453,2.83977664845263));
#28801=CARTESIAN_POINT('Ctrl Pts',(-25.2228521773581,89.0543424461441,2.68179348320399));
#28802=CARTESIAN_POINT('Ctrl Pts',(-27.1351717086426,91.4143489046793,2.52381031795536));
#28803=CARTESIAN_POINT('Ctrl Pts',(-26.2037764083394,94.3055683900266,2.36582715270672));
#28804=CARTESIAN_POINT('Ctrl Pts',(-23.2734951478333,95.1055433482707,2.20784398745809));
#28805=CARTESIAN_POINT('Ctrl Pts',(-21.0021490526171,93.0887157421965,2.04986082220945));
#28806=CARTESIAN_POINT('Ctrl Pts',(-21.4500163995022,90.084321978353,1.89187765696082));
#28807=CARTESIAN_POINT('Ctrl Pts',(-24.210682748199,88.8176438938542,1.73389449171219));
#28808=CARTESIAN_POINT('Ctrl Pts',(-26.7805041627851,90.4372052713962,1.57591132646355));
#28809=CARTESIAN_POINT('Ctrl Pts',(-26.8277997762314,93.4748183557424,1.41792816121491));
#28810=CARTESIAN_POINT('Ctrl Pts',(-24.3112335155169,95.1736105813595,1.25994499596628));
#28811=CARTESIAN_POINT('Ctrl Pts',(-21.5102242410122,93.9961091691131,1.10196183071765));
#28812=CARTESIAN_POINT('Ctrl Pts',(-20.9719518902951,91.0033770531542,0.943978665469013));
#28813=CARTESIAN_POINT('Ctrl Pts',(-22.4379643297735,89.6198434520492,0.838656555303256));
#28814=CARTESIAN_POINT('Ctrl Pts',(-23.301933573839,89.3888678140614,0.785995500220377));
#28815=CARTESIAN_POINT('Ctrl Pts',(-21.8048028959809,93.8768634390787,10.2140044997796));
#28816=CARTESIAN_POINT('Ctrl Pts',(-21.1837878836397,93.1505184486767,10.1613434446967));
#28817=CARTESIAN_POINT('Ctrl Pts',(-20.7302302947449,91.0448125029107,10.056021334531));
#28818=CARTESIAN_POINT('Ctrl Pts',(-23.0156867625841,88.7351875643265,9.89803816928235));
#28819=CARTESIAN_POINT('Ctrl Pts',(-26.1950062090231,89.3936689477181,9.74005500403371));
#28820=CARTESIAN_POINT('Ctrl Pts',(-27.3828721636666,92.4128767408671,9.58207183878509));
#28821=CARTESIAN_POINT('Ctrl Pts',(-25.5026093707801,95.059203920966,9.42408867353644));
#28822=CARTESIAN_POINT('Ctrl Pts',(-22.2593052903593,94.9299391890853,9.26610550828782));
#28823=CARTESIAN_POINT('Ctrl Pts',(-20.5949311131986,92.1435062136747,9.10812234303918));
#28824=CARTESIAN_POINT('Ctrl Pts',(-22.019041067396,89.2267188897615,8.95013917779055));
#28825=CARTESIAN_POINT('Ctrl Pts',(-25.2399628684864,88.8254848953298,8.79215601254191));
#28826=CARTESIAN_POINT('Ctrl Pts',(-27.3361889343087,91.3035990578311,8.63417284729328));
#28827=CARTESIAN_POINT('Ctrl Pts',(-26.4063812377719,94.4133948742933,8.47618968204464));
#28828=CARTESIAN_POINT('Ctrl Pts',(-23.2939019232727,95.3341482798463,8.31820651679601));
#28829=CARTESIAN_POINT('Ctrl Pts',(-20.821878497644,93.2307207244612,8.16022335154738));
#28830=CARTESIAN_POINT('Ctrl Pts',(-21.2325193430214,90.0109848545807,8.00224018629874));
#28831=CARTESIAN_POINT('Ctrl Pts',(-24.1533598039853,88.5953548891582,7.84425702105011));
#28832=CARTESIAN_POINT('Ctrl Pts',(-26.9350975904653,90.2678536211836,7.68627385580147));
#28833=CARTESIAN_POINT('Ctrl Pts',(-27.0546017290974,93.5114685471691,7.52829069055283));
#28834=CARTESIAN_POINT('Ctrl Pts',(-24.4034778158886,95.3841297611199,7.37030752530421));
#28835=CARTESIAN_POINT('Ctrl Pts',(-21.3863857635864,94.1872698476289,7.21232436005556));
#28836=CARTESIAN_POINT('Ctrl Pts',(-20.7399310263462,91.0064814901395,7.05434119480693));
#28837=CARTESIAN_POINT('Ctrl Pts',(-23.0504701241054,88.7268483496341,6.8963580295583));
#28838=CARTESIAN_POINT('Ctrl Pts',(-26.222265227443,89.4160754670625,6.73837486430966));
#28839=CARTESIAN_POINT('Ctrl Pts',(-27.378389919474,92.449010334975,6.58039169906103));
#28840=CARTESIAN_POINT('Ctrl Pts',(-25.4701996425288,95.0746775013101,6.42240853381239));
#28841=CARTESIAN_POINT('Ctrl Pts',(-22.2284881089027,94.9115072296366,6.26442536856376));
#28842=CARTESIAN_POINT('Ctrl Pts',(-20.5935983259232,92.1075005242027,6.10644220331512));
#28843=CARTESIAN_POINT('Ctrl Pts',(-22.0484311291595,89.205987174338,5.9484590380665));
#28844=CARTESIAN_POINT('Ctrl Pts',(-25.2734035094609,88.8387388228741,5.79047587281786));
#28845=CARTESIAN_POINT('Ctrl Pts',(-27.3433554426941,91.3388622597476,5.63249270756922));
#28846=CARTESIAN_POINT('Ctrl Pts',(-26.3807698735208,94.4386601930392,5.47450954232059));
#28847=CARTESIAN_POINT('Ctrl Pts',(-23.2587447682671,95.3265100945794,5.31652637707196));
#28848=CARTESIAN_POINT('Ctrl Pts',(-20.8090634588646,93.1971017993658,5.15854321182332));
#28849=CARTESIAN_POINT('Ctrl Pts',(-21.2536705056942,89.9818813125677,5.00056004657469));
#28850=CARTESIAN_POINT('Ctrl Pts',(-24.1892921421406,88.5971633578074,4.84257688132605));
#28851=CARTESIAN_POINT('Ctrl Pts',(-26.9532193443741,90.2989343839904,4.68459371607741));
#28852=CARTESIAN_POINT('Ctrl Pts',(-27.0384758022577,93.5436299841646,4.52661055082878));
#28853=CARTESIAN_POINT('Ctrl Pts',(-24.3677309963625,95.3882005028233,4.36862738558015));
#28854=CARTESIAN_POINT('Ctrl Pts',(-21.3634416282571,94.1595575157663,4.21064422033151));
#28855=CARTESIAN_POINT('Ctrl Pts',(-20.7506006887122,90.9721221579303,4.05266105508288));
#28856=CARTESIAN_POINT('Ctrl Pts',(-23.085075845721,88.7170070735612,3.89467788983424));
#28857=CARTESIAN_POINT('Ctrl Pts',(-26.2494184139641,89.4396786555336,3.73669472458561));
#28858=CARTESIAN_POINT('Ctrl Pts',(-27.3734617543622,92.4846490321267,3.57871155933697));
#28859=CARTESIAN_POINT('Ctrl Pts',(-25.4376600357343,95.0900263048807,3.42072839408834));
#28860=CARTESIAN_POINT('Ctrl Pts',(-22.1978518073487,94.8926440244144,3.26274522883971));
#28861=CARTESIAN_POINT('Ctrl Pts',(-20.592653065758,92.071535342105,3.10476206359107));
#28862=CARTESIAN_POINT('Ctrl Pts',(-22.0780351821522,89.1855407225702,2.94677889834244));
#28863=CARTESIAN_POINT('Ctrl Pts',(-25.3067031745353,88.8523586513677,2.7887957330938));
#28864=CARTESIAN_POINT('Ctrl Pts',(-27.3501504926354,91.3741907978781,2.63081256784517));
#28865=CARTESIAN_POINT('Ctrl Pts',(-26.354889398786,94.4636612586034,2.47282940259654));
#28866=CARTESIAN_POINT('Ctrl Pts',(-23.2236786962326,95.3184905150264,2.3148462373479));
#28867=CARTESIAN_POINT('Ctrl Pts',(-20.7965863558489,93.1633690014506,2.15686307209926));
#28868=CARTESIAN_POINT('Ctrl Pts',(-21.2751639752712,89.952963899789,1.99887990685063));
#28869=CARTESIAN_POINT('Ctrl Pts',(-24.2251292682703,88.5994296748227,1.840896741602));
#28870=CARTESIAN_POINT('Ctrl Pts',(-26.9711633863787,90.3300444069818,1.68291357635336));
#28871=CARTESIAN_POINT('Ctrl Pts',(-27.021702060943,93.575946678588,1.52493041110472));
#28872=CARTESIAN_POINT('Ctrl Pts',(-24.3325748036253,95.3912251195891,1.3669472458561));
#28873=CARTESIAN_POINT('Ctrl Pts',(-21.3395002696245,94.1329824129964,1.20896408060746));
#28874=CARTESIAN_POINT('Ctrl Pts',(-20.7643185735292,90.9350385986377,1.05098091535882));
#28875=CARTESIAN_POINT('Ctrl Pts',(-22.3308555140066,89.4566360720578,0.945658805193066));
#28876=CARTESIAN_POINT('Ctrl Pts',(-23.2540671456531,89.2098224301578,0.892997750110188));
#28877=CARTESIAN_POINT('Ctrl Pts',(-21.6639373423038,93.9973015569306,10.3210067496694));
#28878=CARTESIAN_POINT('Ctrl Pts',(-21.0030718657857,93.2243470893904,10.2683456945866));
#28879=CARTESIAN_POINT('Ctrl Pts',(-20.520409536926,90.9835182276056,10.1630235844208));
#28880=CARTESIAN_POINT('Ctrl Pts',(-22.9525234917661,88.5256849139446,10.0050404191722));
#28881=CARTESIAN_POINT('Ctrl Pts',(-26.3358595129894,89.2264209743707,9.84705725392353));
#28882=CARTESIAN_POINT('Ctrl Pts',(-27.5999506936452,92.4393709953448,9.68907408867489));
#28883=CARTESIAN_POINT('Ctrl Pts',(-25.5990316467514,95.2555126958587,9.53109092342626));
#28884=CARTESIAN_POINT('Ctrl Pts',(-22.1476051047098,95.1179530605298,9.37310775817762));
#28885=CARTESIAN_POINT('Ctrl Pts',(-20.3764282219686,92.1527149914235,9.215124592929));
#28886=CARTESIAN_POINT('Ctrl Pts',(-21.8919231533181,89.0487577497888,9.05714142768035));
#28887=CARTESIAN_POINT('Ctrl Pts',(-25.3195311476576,88.6217766146216,8.89915826243172));
#28888=CARTESIAN_POINT('Ctrl Pts',(-27.5502718066586,91.2589110869332,8.74117509718309));
#28889=CARTESIAN_POINT('Ctrl Pts',(-26.5607984537915,94.5682621545871,8.58319193193445));
#28890=CARTESIAN_POINT('Ctrl Pts',(-23.24859168833,95.5481002036266,8.42520876668582));
#28891=CARTESIAN_POINT('Ctrl Pts',(-20.6179387947979,93.3096959362796,8.26722560143718));
#28892=CARTESIAN_POINT('Ctrl Pts',(-21.0549304174885,89.8833499742237,8.10924243618856));
#28893=CARTESIAN_POINT('Ctrl Pts',(-24.1632008855267,88.3768791915844,7.95125927093991));
#28894=CARTESIAN_POINT('Ctrl Pts',(-27.123442475952,90.156701980971,7.79327610569129));
#28895=CARTESIAN_POINT('Ctrl Pts',(-27.2506151818504,93.6084593155026,7.63529294044264));
#28896=CARTESIAN_POINT('Ctrl Pts',(-24.4293689423972,95.6012889909869,7.47730977519402));
#28897=CARTESIAN_POINT('Ctrl Pts',(-21.2186704291245,94.3276267101463,7.31932660994538));
#28898=CARTESIAN_POINT('Ctrl Pts',(-20.5307327633938,90.9427275180138,7.16134344469674));
#28899=CARTESIAN_POINT('Ctrl Pts',(-22.9895388977221,88.5168105727741,7.00336027944811));
#28900=CARTESIAN_POINT('Ctrl Pts',(-26.3648677395855,89.2502653175659,6.84537711419947));
#28901=CARTESIAN_POINT('Ctrl Pts',(-27.5951808243418,92.4778232781622,6.68739394895084));
#28902=CARTESIAN_POINT('Ctrl Pts',(-25.5645421898479,95.27197921413,6.5294107837022));
#28903=CARTESIAN_POINT('Ctrl Pts',(-22.1148103881513,95.0983383242963,6.37142761845358));
#28904=CARTESIAN_POINT('Ctrl Pts',(-20.3750099098822,92.114398820868,6.21344445320493));
#28905=CARTESIAN_POINT('Ctrl Pts',(-21.9231991720717,89.0266956824957,6.05546128795631));
#28906=CARTESIAN_POINT('Ctrl Pts',(-25.355117670839,88.6358810452203,5.89747812270766));
#28907=CARTESIAN_POINT('Ctrl Pts',(-27.557898189089,91.2964371245891,5.73949495745904));
#28908=CARTESIAN_POINT('Ctrl Pts',(-26.5335436111487,94.5951487460233,5.5815117922104));
#28909=CARTESIAN_POINT('Ctrl Pts',(-23.2111785026033,95.5399718768618,5.42352862696177));
#28910=CARTESIAN_POINT('Ctrl Pts',(-20.6043014164074,93.2739196885051,5.26554546171313));
#28911=CARTESIAN_POINT('Ctrl Pts',(-21.0774388479142,89.8523788611612,5.1075622964645));
#28912=CARTESIAN_POINT('Ctrl Pts',(-24.2014389978196,88.3788037094653,4.94957913121586));
#28913=CARTESIAN_POINT('Ctrl Pts',(-27.1427271007907,90.1897771928657,4.79159596596723));
#28914=CARTESIAN_POINT('Ctrl Pts',(-27.2334544560815,93.6426845483281,4.63361280071859));
#28915=CARTESIAN_POINT('Ctrl Pts',(-24.3913282534434,95.6056209517321,4.47562963546996));
#28916=CARTESIAN_POINT('Ctrl Pts',(-21.1942539711864,94.2981360810344,4.31764647022132));
#28917=CARTESIAN_POINT('Ctrl Pts',(-20.5420870968054,90.9061633512837,4.15966330497269));
#28918=CARTESIAN_POINT('Ctrl Pts',(-23.0263652646397,88.5063377831116,4.00168013972405));
#28919=CARTESIAN_POINT('Ctrl Pts',(-26.3937633430615,89.2753831200125,3.84369697447542));
#28920=CARTESIAN_POINT('Ctrl Pts',(-27.5899364194237,92.5157489065408,3.68571380922678));
#28921=CARTESIAN_POINT('Ctrl Pts',(-25.5299145201095,95.2883129487163,3.52773064397815));
#28922=CARTESIAN_POINT('Ctrl Pts',(-22.0822081585386,95.0782646692958,3.36974747872952));
#28923=CARTESIAN_POINT('Ctrl Pts',(-20.3740039924776,92.0761257570406,3.21176431348088));
#28924=CARTESIAN_POINT('Ctrl Pts',(-21.9547029138477,89.0049371841951,3.05378114823225));
#28925=CARTESIAN_POINT('Ctrl Pts',(-25.3905541717125,88.6503748565914,2.89579798298361));
#28926=CARTESIAN_POINT('Ctrl Pts',(-27.5651292766281,91.3340326910768,2.73781481773498));
#28927=CARTESIAN_POINT('Ctrl Pts',(-26.5060023892327,94.6217541271801,2.57983165248635));
#28928=CARTESIAN_POINT('Ctrl Pts',(-23.1738622446318,95.5314376817822,2.42184848723771));
#28929=CARTESIAN_POINT('Ctrl Pts',(-20.5910236590807,93.2380222607045,2.26386532198907));
#28930=CARTESIAN_POINT('Ctrl Pts',(-21.1003115510402,89.8216058212251,2.10588215674044));
#28931=CARTESIAN_POINT('Ctrl Pts',(-24.2395757883417,88.3812154557912,1.94789899149181));
#28932=CARTESIAN_POINT('Ctrl Pts',(-27.1618226099723,90.2228835425675,1.78991582624317));
#28933=CARTESIAN_POINT('Ctrl Pts',(-27.2156043456547,93.6770750014334,1.63193266099454));
#28934=CARTESIAN_POINT('Ctrl Pts',(-24.3539160917338,95.6088396578189,1.4739494957459));
#28935=CARTESIAN_POINT('Ctrl Pts',(-21.1687762982368,94.2698556568795,1.31596633049727));
#28936=CARTESIAN_POINT('Ctrl Pts',(-20.5566852567634,90.8667001441213,1.15798316524863));
#28937=CARTESIAN_POINT('Ctrl Pts',(-22.2237466982397,89.2934286920664,1.05266105508288));
#28938=CARTESIAN_POINT('Ctrl Pts',(-23.2062007174672,89.0307770462543,0.999999999999999));
#28939=CARTESIAN_POINT('Ctrl Pts',(-22.0865340033349,93.6359872033749,10.));
#28940=CARTESIAN_POINT('Ctrl Pts',(-22.0249228618564,93.5780878591467,10.));
#28941=CARTESIAN_POINT('Ctrl Pts',(-21.966680820328,93.517037957369,10.));
#28942=CARTESIAN_POINT('Ctrl Pts',(-21.9118055510414,93.4532222734472,10.));
#28943=CARTESIAN_POINT('Ctrl Pts',(-21.8554775805296,93.3877172106225,10.));
#28944=CARTESIAN_POINT('Ctrl Pts',(-21.8026965604156,93.319297559701,10.));
#28945=CARTESIAN_POINT('Ctrl Pts',(-21.7534854803777,93.2483309191729,10.));
#28946=CARTESIAN_POINT('Ctrl Pts',(-21.7029129709051,93.1754009794607,10.));
#28947=CARTESIAN_POINT('Ctrl Pts',(-21.6561101248005,93.0997806200771,10.));
#28948=CARTESIAN_POINT('Ctrl Pts',(-21.6131359910424,93.0218257865766,10.));
#28949=CARTESIAN_POINT('Ctrl Pts',(-21.5942445812211,92.9875568769228,10.));
#28950=CARTESIAN_POINT('Ctrl Pts',(-21.5760935456704,92.9528363378501,10.));
#28951=CARTESIAN_POINT('Ctrl Pts',(-21.558690318408,92.917692336787,10.));
#28952=CARTESIAN_POINT('Ctrl Pts',(-21.548765297561,92.8976497930713,10.));
#28953=CARTESIAN_POINT('Ctrl Pts',(-21.5390835217549,92.877469502106,10.));
#28954=CARTESIAN_POINT('Ctrl Pts',(-21.5296466035414,92.8571565405433,10.));
#28955=CARTESIAN_POINT('Ctrl Pts',(-21.5211295714091,92.8388236332939,10.));
#28956=CARTESIAN_POINT('Ctrl Pts',(-21.5128096038615,92.8203769112349,10.));
#28957=CARTESIAN_POINT('Ctrl Pts',(-21.5047015810338,92.8018519372552,10.));
#28958=CARTESIAN_POINT('Ctrl Pts',(-21.4681367627671,92.7183097073719,10.));
#28959=CARTESIAN_POINT('Ctrl Pts',(-21.4358322656584,92.6330839819686,10.));
#28960=CARTESIAN_POINT('Ctrl Pts',(-21.4078131930248,92.5465734750324,10.));
#28961=CARTESIAN_POINT('Ctrl Pts',(-21.3793314408844,92.4586344183647,10.));
#28962=CARTESIAN_POINT('Ctrl Pts',(-21.355277318963,92.3693670435349,10.));
#28963=CARTESIAN_POINT('Ctrl Pts',(-21.3357162703818,92.2791530220287,10.));
#28964=CARTESIAN_POINT('Ctrl Pts',(-21.3167358111454,92.1916166330335,10.));
#28965=CARTESIAN_POINT('Ctrl Pts',(-21.3019855060024,92.1031880411159,10.));
#28966=CARTESIAN_POINT('Ctrl Pts',(-21.2915659618292,92.014194029087,10.));
#28967=CARTESIAN_POINT('Ctrl Pts',(-21.2872066009676,91.9769604412726,10.));
#28968=CARTESIAN_POINT('Ctrl Pts',(-21.2836058304749,91.9396276882027,10.));
#28969=CARTESIAN_POINT('Ctrl Pts',(-21.2807733396412,91.902219087546,10.));
#28970=CARTESIAN_POINT('Ctrl Pts',(-21.279002750376,91.8788349812459,10.));
#28971=CARTESIAN_POINT('Ctrl Pts',(-21.277532394138,91.8554212321296,10.));
#28972=CARTESIAN_POINT('Ctrl Pts',(-21.2763649279069,91.8319835034305,10.));
#28973=CARTESIAN_POINT('Ctrl Pts',(-21.2756806561547,91.8182462532588,10.));
#28974=CARTESIAN_POINT('Ctrl Pts',(-21.2751007108994,91.8045053338933,10.));
#28975=CARTESIAN_POINT('Ctrl Pts',(-21.2746256143519,91.790770119806,10.));
#28976=CARTESIAN_POINT('Ctrl Pts',(-21.2712677542687,91.6936931627977,10.));
#28977=CARTESIAN_POINT('Ctrl Pts',(-21.2731370867467,91.5967807433318,10.));
#28978=CARTESIAN_POINT('Ctrl Pts',(-21.2802984098211,91.5004551184403,10.));
#28979=CARTESIAN_POINT('Ctrl Pts',(-21.2874597328954,91.4041294935487,10.));
#28980=CARTESIAN_POINT('Ctrl Pts',(-21.2999126116946,91.3083896087231,10.));
#28981=CARTESIAN_POINT('Ctrl Pts',(-21.3177747368199,91.2136387821642,10.));
#28982=CARTESIAN_POINT('Ctrl Pts',(-21.3348522432755,91.1230500173404,10.));
#28983=CARTESIAN_POINT('Ctrl Pts',(-21.3568741021771,91.0333643557261,10.));
#28984=CARTESIAN_POINT('Ctrl Pts',(-21.3835656166832,90.9448211375735,10.));
#28985=CARTESIAN_POINT('Ctrl Pts',(-21.3925004778797,90.9151817042657,10.));
#28986=CARTESIAN_POINT('Ctrl Pts',(-21.4019590305019,90.8856703233236,10.));
#28987=CARTESIAN_POINT('Ctrl Pts',(-21.4119322462714,90.8562961512492,10.));
#28988=CARTESIAN_POINT('Ctrl Pts',(-21.4184134249047,90.8372070970445,10.));
#28989=CARTESIAN_POINT('Ctrl Pts',(-21.4251119666752,90.8181759907897,10.));
#28990=CARTESIAN_POINT('Ctrl Pts',(-21.432025530206,90.7992053804605,10.));
#28991=CARTESIAN_POINT('Ctrl Pts',(-21.4386151870839,90.781123560242,10.));
#28992=CARTESIAN_POINT('Ctrl Pts',(-21.4454019414903,90.7630924899962,10.));
#28993=CARTESIAN_POINT('Ctrl Pts',(-21.452372973352,90.7451415274744,10.));
#28994=CARTESIAN_POINT('Ctrl Pts',(-21.4862164573767,90.6579918593344,10.));
#28995=CARTESIAN_POINT('Ctrl Pts',(-21.5244382858088,90.5726164812308,10.));
#28996=CARTESIAN_POINT('Ctrl Pts',(-21.5667072739919,90.4892490087442,10.));
#28997=CARTESIAN_POINT('Ctrl Pts',(-21.6105455323499,90.4027864518056,10.));
#28998=CARTESIAN_POINT('Ctrl Pts',(-21.6587371595505,90.3184829337529,10.));
#28999=CARTESIAN_POINT('Ctrl Pts',(-21.7109686726983,90.2366020739748,10.));
#29000=CARTESIAN_POINT('Ctrl Pts',(-21.7637886184686,90.1537987563519,10.));
#29001=CARTESIAN_POINT('Ctrl Pts',(-21.8207403975229,90.0734721713631,10.));
#29002=CARTESIAN_POINT('Ctrl Pts',(-21.8815515974698,89.9959097942702,10.));
#29003=CARTESIAN_POINT('Ctrl Pts',(-21.9232140422193,89.9427709275303,10.));
#29004=CARTESIAN_POINT('Ctrl Pts',(-21.9666890946703,89.8909298239753,10.));
#29005=CARTESIAN_POINT('Ctrl Pts',(-22.0119013665037,89.8404859712607,10.));
#29006=CARTESIAN_POINT('Ctrl Pts',(-22.0240086331348,89.8269777543553,10.));
#29007=CARTESIAN_POINT('Ctrl Pts',(-22.0362418077641,89.8135685184895,10.));
#29008=CARTESIAN_POINT('Ctrl Pts',(-22.0485858237953,89.800274672024,10.));
#29009=CARTESIAN_POINT('Ctrl Pts',(-22.1172467098524,89.7263305621724,10.));
#29010=CARTESIAN_POINT('Ctrl Pts',(-22.1894214869168,89.6558543371947,10.));
#29011=CARTESIAN_POINT('Ctrl Pts',(-22.2647996928107,89.5891358089895,10.));
#29012=CARTESIAN_POINT('Ctrl Pts',(-22.3277046148832,89.5334575958008,10.));
#29013=CARTESIAN_POINT('Ctrl Pts',(-22.3928415833451,89.4803963686579,10.));
#29014=CARTESIAN_POINT('Ctrl Pts',(-22.460053826701,89.4301343334532,10.));
#29015=CARTESIAN_POINT('Ctrl Pts',(-22.4819361315296,89.4137705116145,10.));
#29016=CARTESIAN_POINT('Ctrl Pts',(-22.5040385611967,89.3977035154392,10.));
#29017=CARTESIAN_POINT('Ctrl Pts',(-22.5263561315554,89.3819400183082,10.));
#29018=CARTESIAN_POINT('Ctrl Pts',(-22.5491248910509,89.3658578342168,10.));
#29019=CARTESIAN_POINT('Ctrl Pts',(-22.5721229921732,89.3500881169297,10.));
#29020=CARTESIAN_POINT('Ctrl Pts',(-22.595316006075,89.33465717982,10.));
#29021=CARTESIAN_POINT('Ctrl Pts',(-22.6802613709847,89.2781407396011,10.));
#29022=CARTESIAN_POINT('Ctrl Pts',(-22.7678730042567,89.2261247336488,10.));
#29023=CARTESIAN_POINT('Ctrl Pts',(-22.8578606395619,89.1789172288512,10.));
#29024=CARTESIAN_POINT('Ctrl Pts',(-22.9411343064062,89.1352318712602,10.));
#29025=CARTESIAN_POINT('Ctrl Pts',(-23.0264434722402,89.0956640032309,10.));
#29026=CARTESIAN_POINT('Ctrl Pts',(-23.1135855312338,89.060486601523,10.));
#29027=CARTESIAN_POINT('Ctrl Pts',(-23.14360948864,89.0483665664591,10.));
#29028=CARTESIAN_POINT('Ctrl Pts',(-23.1738512261799,89.0367679981665,10.));
#29029=CARTESIAN_POINT('Ctrl Pts',(-23.2042983602307,89.0256873161863,10.));
#29030=CARTESIAN_POINT('Ctrl Pts',(-26.5182105203766,91.9978055611691,8.38741669750802));
#29031=CARTESIAN_POINT('Ctrl Pts',(-26.5197765073294,91.8252749644444,8.39833391417657));
#29032=CARTESIAN_POINT('Ctrl Pts',(-26.5035405383448,91.6530372868482,8.40925113084511));
#29033=CARTESIAN_POINT('Ctrl Pts',(-26.4684109790521,91.4847436281601,8.42016834751366));
#29034=CARTESIAN_POINT('Ctrl Pts',(-26.2989575631207,90.6729504853336,8.47282940259653));
#29035=CARTESIAN_POINT('Ctrl Pts',(-25.6898919366324,89.95292597104,8.52549045767941));
#29036=CARTESIAN_POINT('Ctrl Pts',(-24.9174342209562,89.6512036660532,8.57815151276229));
#29037=CARTESIAN_POINT('Ctrl Pts',(-24.14497650528,89.3494813610665,8.63081256784517));
#29038=CARTESIAN_POINT('Ctrl Pts',(-23.2091267004159,89.4660612653866,8.68347362292804));
#29039=CARTESIAN_POINT('Ctrl Pts',(-22.5343117980016,89.9480924656251,8.73613467801092));
#29040=CARTESIAN_POINT('Ctrl Pts',(-21.8594968955873,90.4301236658636,8.7887957330938));
#29041=CARTESIAN_POINT('Ctrl Pts',(-21.4457168956229,91.2776061620205,8.84145678817668));
#29042=CARTESIAN_POINT('Ctrl Pts',(-21.480621689974,92.1061512081021,8.89411784325956));
#29043=CARTESIAN_POINT('Ctrl Pts',(-21.5155264843251,92.9346962541837,8.94677889834244));
#29044=CARTESIAN_POINT('Ctrl Pts',(-21.9991160729917,93.7443038501899,8.99943995342531));
#29045=CARTESIAN_POINT('Ctrl Pts',(-22.7120873935215,94.1678868023571,9.05210100850819));
#29046=CARTESIAN_POINT('Ctrl Pts',(-23.4250587140513,94.5914697545244,9.10476206359107));
#29047=CARTESIAN_POINT('Ctrl Pts',(-24.3674117664444,94.6290280628526,9.15742311867395));
#29048=CARTESIAN_POINT('Ctrl Pts',(-25.1117466734529,94.2633575271385,9.21008417375683));
#29049=CARTESIAN_POINT('Ctrl Pts',(-25.8560815804615,93.8976869914244,9.26274522883971));
#29050=CARTESIAN_POINT('Ctrl Pts',(-26.4023983420856,93.1287876116681,9.31540628392258));
#29051=CARTESIAN_POINT('Ctrl Pts',(-26.502987472461,92.3057173655401,9.36806733900546));
#29052=CARTESIAN_POINT('Ctrl Pts',(-26.5153073620014,92.2049099077324,9.37451712517298));
#29053=CARTESIAN_POINT('Ctrl Pts',(-26.5209410251377,92.1032898490186,9.3809669113405));
#29054=CARTESIAN_POINT('Ctrl Pts',(-26.5201758362126,92.0015868137837,9.38741669750802));
#29055=CARTESIAN_POINT('Ctrl Pts',(-24.7937992825329,89.0307770462543,10.));
#29056=CARTESIAN_POINT('Ctrl Pts',(-25.7762533017603,89.2934286920664,9.94733894491712));
#29057=CARTESIAN_POINT('Ctrl Pts',(-27.443314608871,90.8667010511062,9.84201683475136));
#29058=CARTESIAN_POINT('Ctrl Pts',(-26.8312238178928,94.2698553838416,9.68403366950273));
#29059=CARTESIAN_POINT('Ctrl Pts',(-23.6460838986402,95.6088399383518,9.5260505042541));
#29060=CARTESIAN_POINT('Ctrl Pts',(-20.7843955634607,93.6770749374766,9.36806733900546));
#29061=CARTESIAN_POINT('Ctrl Pts',(-20.8381773234134,90.2228835564638,9.21008417375683));
#29062=CARTESIAN_POINT('Ctrl Pts',(-23.760424197283,88.3812153351417,9.05210100850819));
#29063=CARTESIAN_POINT('Ctrl Pts',(-26.8996885260907,89.8216057842524,8.89411784325956));
#29064=CARTESIAN_POINT('Ctrl Pts',(-27.4089764216848,93.2380222823145,8.73613467801092));
#29065=CARTESIAN_POINT('Ctrl Pts',(-24.8261377777637,95.5314377737091,8.57815151276229));
#29066=CARTESIAN_POINT('Ctrl Pts',(-21.493997547754,94.6217541894132,8.42016834751366));
#29067=CARTESIAN_POINT('Ctrl Pts',(-20.4348706359933,91.3340326759415,8.26218518226502));
#29068=CARTESIAN_POINT('Ctrl Pts',(-22.6094457936036,88.6503747732116,8.10420201701639));
#29069=CARTESIAN_POINT('Ctrl Pts',(-26.0452971368403,89.0049371106047,7.94621885176775));
#29070=CARTESIAN_POINT('Ctrl Pts',(-27.6259960969404,92.0761257587368,7.78823568651912));
#29071=CARTESIAN_POINT('Ctrl Pts',(-25.9177918888646,95.0782647453892,7.63025252127048));
#29072=CARTESIAN_POINT('Ctrl Pts',(-22.4700854420894,95.288313029852,7.47226935602185));
#29073=CARTESIAN_POINT('Ctrl Pts',(-20.4100634919605,92.5157489192991,7.31428619077322));
#29074=CARTESIAN_POINT('Ctrl Pts',(-21.6062365978313,89.275383052732,7.15630302552458));
#29075=CARTESIAN_POINT('Ctrl Pts',(-24.9736347594025,88.5063376968639,6.99831986027595));
#29076=CARTESIAN_POINT('Ctrl Pts',(-27.4579129885641,90.9061633242749,6.84033669502731));
#29077=CARTESIAN_POINT('Ctrl Pts',(-26.8057460980852,94.2981361377744,6.68235352977868));
#29078=CARTESIAN_POINT('Ctrl Pts',(-23.6086717368945,95.6056210407497,6.52437036453004));
#29079=CARTESIAN_POINT('Ctrl Pts',(-20.7665454640887,93.6426845888844,6.36638719928141));
#29080=CARTESIAN_POINT('Ctrl Pts',(-20.857272821619,90.1897771481731,6.20840403403277));
#29081=CARTESIAN_POINT('Ctrl Pts',(-23.7985609972073,88.3788036200625,6.05042086878414));
#29082=CARTESIAN_POINT('Ctrl Pts',(-26.9225612242403,89.8523788081389,5.89243770353549));
#29083=CARTESIAN_POINT('Ctrl Pts',(-27.3956986674284,93.2739197199569,5.73445453828688));
#29084=CARTESIAN_POINT('Ctrl Pts',(-24.7888215168716,95.5399719642594,5.57647137303822));
#29085=CARTESIAN_POINT('Ctrl Pts',(-21.4664563263011,94.5951488100945,5.41848820778961));
#29086=CARTESIAN_POINT('Ctrl Pts',(-20.4421017230708,91.2964371072188,5.26050504254096));
#29087=CARTESIAN_POINT('Ctrl Pts',(-22.6448822957049,88.6358809621643,5.10252187729233));
#29088=CARTESIAN_POINT('Ctrl Pts',(-26.0768008792021,89.0266956090883,4.9445387120437));
#29089=CARTESIAN_POINT('Ctrl Pts',(-27.6249901796144,92.1143988236926,4.78655554679506));
#29090=CARTESIAN_POINT('Ctrl Pts',(-25.8851896583917,95.0983384007904,4.62857238154643));
#29091=CARTESIAN_POINT('Ctrl Pts',(-22.4354577715254,95.2719792949115,4.47058921629779));
#29092=CARTESIAN_POINT('Ctrl Pts',(-20.4048190868974,92.4778232899584,4.31260605104916));
#29093=CARTESIAN_POINT('Ctrl Pts',(-21.6351322020288,89.2502652496793,4.15462288580052));
#29094=CARTESIAN_POINT('Ctrl Pts',(-25.010461127225,88.5168104867762,3.99663972055189));
#29095=CARTESIAN_POINT('Ctrl Pts',(-27.4692673222584,90.9427274919152,3.83865655530326));
#29096=CARTESIAN_POINT('Ctrl Pts',(-26.7813296395429,94.327626767605,3.68067339005462));
#29097=CARTESIAN_POINT('Ctrl Pts',(-23.5706310470027,95.6012890799134,3.52269022480599));
#29098=CARTESIAN_POINT('Ctrl Pts',(-20.7493847378944,93.6084593551842,3.36470705955735));
#29099=CARTESIAN_POINT('Ctrl Pts',(-20.8765574469375,90.1567019355188,3.20672389430872));
#29100=CARTESIAN_POINT('Ctrl Pts',(-23.8367991104361,88.3768791020246,3.04874072906008));
#29101=CARTESIAN_POINT('Ctrl Pts',(-26.9450696552404,89.8833499221761,2.89075756381144));
#29102=CARTESIAN_POINT('Ctrl Pts',(-27.3820612886588,93.3096959682138,2.73277439856281));
#29103=CARTESIAN_POINT('Ctrl Pts',(-24.7514083303165,95.5481002919865,2.57479123331418));
#29104=CARTESIAN_POINT('Ctrl Pts',(-21.4392014827728,94.5682622165549,2.41680806806554));
#29105=CARTESIAN_POINT('Ctrl Pts',(-20.4497281061605,91.2589110713399,2.25882490281691));
#29106=CARTESIAN_POINT('Ctrl Pts',(-22.6804688187274,88.6217765261786,2.10084173756827));
#29107=CARTESIAN_POINT('Ctrl Pts',(-26.1080769010003,89.0487576862312,1.94285857231964));
#29108=CARTESIAN_POINT('Ctrl Pts',(-27.623571862538,92.1527149782027,1.784875407071));
#29109=CARTESIAN_POINT('Ctrl Pts',(-25.8523949517842,95.1179531681003,1.62689224182237));
#29110=CARTESIAN_POINT('Ctrl Pts',(-22.40096829048,95.2555127221397,1.46890907657374));
#29111=CARTESIAN_POINT('Ctrl Pts',(-20.4000492676845,92.4393710995324,1.3109259113251));
#29112=CARTESIAN_POINT('Ctrl Pts',(-21.6641403201723,89.2264207486354,1.15294274607647));
#29113=CARTESIAN_POINT('Ctrl Pts',(-25.0474767585968,88.5256850731752,0.994959580827833));
#29114=CARTESIAN_POINT('Ctrl Pts',(-27.4795898385891,90.983517556268,0.836976415579199));
#29115=CARTESIAN_POINT('Ctrl Pts',(-26.9969281342143,93.2243470893905,0.731654305413442));
#29116=CARTESIAN_POINT('Ctrl Pts',(-26.3360626576961,93.9973015569307,0.678993250330564));
#29117=CARTESIAN_POINT('Ctrl Pts',(-24.745932854347,89.2098224301578,10.1070022498898));
#29118=CARTESIAN_POINT('Ctrl Pts',(-25.6691444859934,89.4566360720578,10.0543411948069));
#29119=CARTESIAN_POINT('Ctrl Pts',(-27.2356813002074,90.9350394509311,9.94901908464117));
#29120=CARTESIAN_POINT('Ctrl Pts',(-26.6604998395025,94.1329821564226,9.79103591939255));
#29121=CARTESIAN_POINT('Ctrl Pts',(-23.6674251873291,95.3912253832059,9.63305275414391));
#29122=CARTESIAN_POINT('Ctrl Pts',(-20.9782978536527,93.5759466184876,9.47506958889528));
#29123=CARTESIAN_POINT('Ctrl Pts',(-21.0288365510238,90.3300444200403,9.31708642364664));
#29124=CARTESIAN_POINT('Ctrl Pts',(-23.7748707182211,88.5994295614483,9.159103258398));
#29125=CARTESIAN_POINT('Ctrl Pts',(-26.7248360972087,89.9529638650458,9.00112009314937));
#29126=CARTESIAN_POINT('Ctrl Pts',(-27.2034137200465,93.1633690217573,8.84313692790073));
#29127=CARTESIAN_POINT('Ctrl Pts',(-24.7763213248124,95.3184906014102,8.6851537626521));
#29128=CARTESIAN_POINT('Ctrl Pts',(-21.6451105420004,94.4636613170838,8.52717059740347));
#29129=CARTESIAN_POINT('Ctrl Pts',(-20.649849425255,91.3741907836555,8.36918743215483));
#29130=CARTESIAN_POINT('Ctrl Pts',(-22.6932967928723,88.8523585730158,8.2112042669062));
#29131=CARTESIAN_POINT('Ctrl Pts',(-25.9219648654793,89.1855406534173,8.05322110165756));
#29132=CARTESIAN_POINT('Ctrl Pts',(-27.407347018268,92.0715353436988,7.89523793640893));
#29133=CARTESIAN_POINT('Ctrl Pts',(-25.8021482371961,94.8926440959194,7.73725477116029));
#29134=CARTESIAN_POINT('Ctrl Pts',(-22.562339928744,95.0900263811238,7.57927160591167));
#29135=CARTESIAN_POINT('Ctrl Pts',(-20.6265381623655,92.4846490441157,7.42128844066302));
#29136=CARTESIAN_POINT('Ctrl Pts',(-21.7505815304928,89.4396785923101,7.26330527541439));
#29137=CARTESIAN_POINT('Ctrl Pts',(-24.9149241768714,88.7170069925143,7.10532211016575));
#29138=CARTESIAN_POINT('Ctrl Pts',(-27.2493993915096,90.9721221325502,6.94733894491713));
#29139=CARTESIAN_POINT('Ctrl Pts',(-26.6365584368374,94.1595575690848,6.78935577966848));
#29140=CARTESIAN_POINT('Ctrl Pts',(-23.632268994558,95.3882005864732,6.63137261441985));
#29141=CARTESIAN_POINT('Ctrl Pts',(-20.9615241227262,93.5436300222751,6.47338944917122));
#29142=CARTESIAN_POINT('Ctrl Pts',(-21.0467805827144,90.2989343419931,6.31540628392258));
#29143=CARTESIAN_POINT('Ctrl Pts',(-23.8107078531861,88.5971632737953,6.15742311867395));
#29144=CARTESIAN_POINT('Ctrl Pts',(-26.7463295621094,89.9818812627429,5.99943995342531));
#29145=CARTESIAN_POINT('Ctrl Pts',(-27.1909366199158,93.1971018289209,5.84145678817668));
#29146=CARTESIAN_POINT('Ctrl Pts',(-24.7412552500335,95.3265101767069,5.68347362292804));
#29147=CARTESIAN_POINT('Ctrl Pts',(-21.6192300677009,94.4386602532469,5.52549045767941));
#29148=CARTESIAN_POINT('Ctrl Pts',(-20.6566444747624,91.3388622434247,5.36750729243077));
#29149=CARTESIAN_POINT('Ctrl Pts',(-22.7265964591003,88.8387387448265,5.20952412718214));
#29150=CARTESIAN_POINT('Ctrl Pts',(-25.9515689190225,89.2059871053571,5.05154096193351));
#29151=CARTESIAN_POINT('Ctrl Pts',(-27.4064017581768,92.107500526857,4.89355779668487));
#29152=CARTESIAN_POINT('Ctrl Pts',(-25.7715119348338,94.9115073015181,4.73557463143624));
#29153=CARTESIAN_POINT('Ctrl Pts',(-22.5298003211736,95.0746775772204,4.5775914661876));
#29154=CARTESIAN_POINT('Ctrl Pts',(-20.6216099971176,92.4490103460599,4.41960830093897));
#29155=CARTESIAN_POINT('Ctrl Pts',(-21.7777347176919,89.4160754032695,4.26162513569033));
#29156=CARTESIAN_POINT('Ctrl Pts',(-24.9495298993374,88.7268482688219,4.1036419704417));
#29157=CARTESIAN_POINT('Ctrl Pts',(-27.2600690541411,91.0064814656145,3.94565880519306));
#29158=CARTESIAN_POINT('Ctrl Pts',(-26.6136143009403,94.1872699016228,3.78767563994443));
#29159=CARTESIAN_POINT('Ctrl Pts',(-23.5965221741505,95.3841298446841,3.6296924746958));
#29160=CARTESIAN_POINT('Ctrl Pts',(-20.9453981954867,93.5114685844578,3.47170930944716));
#29161=CARTESIAN_POINT('Ctrl Pts',(-21.0649023370739,90.2678535784722,3.31372614419852));
#29162=CARTESIAN_POINT('Ctrl Pts',(-23.8466401922209,88.5953548049988,3.15574297894989));
#29163=CARTESIAN_POINT('Ctrl Pts',(-26.7674807253219,90.0109848056715,2.99775981370126));
#29164=CARTESIAN_POINT('Ctrl Pts',(-27.1781215807802,93.2307207544698,2.83977664845262));
#29165=CARTESIAN_POINT('Ctrl Pts',(-24.7060980942495,95.334148362878,2.68179348320399));
#29166=CARTESIAN_POINT('Ctrl Pts',(-21.5936187026176,94.4133949325243,2.52381031795535));
#29167=CARTESIAN_POINT('Ctrl Pts',(-20.6638109837674,91.3035990431782,2.36582715270672));
#29168=CARTESIAN_POINT('Ctrl Pts',(-22.7600370999256,88.82548481222,2.20784398745809));
#29169=CARTESIAN_POINT('Ctrl Pts',(-25.980958983647,89.2267188300363,2.04986082220945));
#29170=CARTESIAN_POINT('Ctrl Pts',(-27.4050689662123,92.1435062012512,1.89187765696082));
#29171=CARTESIAN_POINT('Ctrl Pts',(-25.740694762728,94.9299392901692,1.73389449171218));
#29172=CARTESIAN_POINT('Ctrl Pts',(-22.4973905702363,95.0592039456622,1.57591132646355));
#29173=CARTESIAN_POINT('Ctrl Pts',(-20.6171277999948,92.4128768387722,1.41792816121491));
#29174=CARTESIAN_POINT('Ctrl Pts',(-21.8049936341991,89.3936687355948,1.25994499596628));
#29175=CARTESIAN_POINT('Ctrl Pts',(-24.9843134726817,88.7351877139554,1.10196183071764));
#29176=CARTESIAN_POINT('Ctrl Pts',(-27.2697691184269,91.0448118720551,0.94397866546901));
#29177=CARTESIAN_POINT('Ctrl Pts',(-26.8162121163602,93.1505184486767,0.838656555303253));
#29178=CARTESIAN_POINT('Ctrl Pts',(-26.1951971040191,93.8768634390788,0.785995500220375));
#29179=CARTESIAN_POINT('Ctrl Pts',(-24.698066426161,89.3888678140614,10.2140044997796));
#29180=CARTESIAN_POINT('Ctrl Pts',(-25.5620356702265,89.6198434520493,10.1613434446967));
#29181=CARTESIAN_POINT('Ctrl Pts',(-27.0280479915439,91.0033778507559,10.056021334531));
#29182=CARTESIAN_POINT('Ctrl Pts',(-26.4897758611121,93.9961089290037,9.89803816928235));
#29183=CARTESIAN_POINT('Ctrl Pts',(-23.688766476018,95.1736108280599,9.74005500403372));
#29184=CARTESIAN_POINT('Ctrl Pts',(-21.1722001438448,93.4748182994988,9.58207183878508));
#29185=CARTESIAN_POINT('Ctrl Pts',(-21.2194957786343,90.4372052836167,9.42408867353644));
#29186=CARTESIAN_POINT('Ctrl Pts',(-23.7893172391594,88.817643787755,9.26610550828782));
#29187=CARTESIAN_POINT('Ctrl Pts',(-26.5499836683267,90.0843219458393,9.10812234303918));
#29188=CARTESIAN_POINT('Ctrl Pts',(-26.9978510184081,93.0887157612002,8.95013917779054));
#29189=CARTESIAN_POINT('Ctrl Pts',(-24.7265048718612,95.1055434291113,8.79215601254191));
#29190=CARTESIAN_POINT('Ctrl Pts',(-21.7962235362467,94.3055684447543,8.63417284729327));
#29191=CARTESIAN_POINT('Ctrl Pts',(-20.8648282145167,91.4143488913694,8.47618968204464));
#29192=CARTESIAN_POINT('Ctrl Pts',(-22.7771477921409,89.0543423728199,8.318206516796));
#29193=CARTESIAN_POINT('Ctrl Pts',(-25.7986325941185,89.36614419623,8.16022335154738));
#29194=CARTESIAN_POINT('Ctrl Pts',(-27.1886979395956,92.0669449286608,8.00224018629874));
#29195=CARTESIAN_POINT('Ctrl Pts',(-25.6865045855277,94.7070234464497,7.84425702105011));
#29196=CARTESIAN_POINT('Ctrl Pts',(-22.6545944153985,94.8917397323956,7.68627385580146));
#29197=CARTESIAN_POINT('Ctrl Pts',(-20.8430128327706,92.4535491689321,7.52829069055284));
#29198=CARTESIAN_POINT('Ctrl Pts',(-21.8949264631544,89.6039741318884,7.3703075253042));
#29199=CARTESIAN_POINT('Ctrl Pts',(-24.8562135943403,88.9276762881646,7.21232436005557));
#29200=CARTESIAN_POINT('Ctrl Pts',(-27.040885794455,91.0380809408257,7.05434119480693));
#29201=CARTESIAN_POINT('Ctrl Pts',(-26.4673707755896,94.0209790003952,6.8963580295583));
#29202=CARTESIAN_POINT('Ctrl Pts',(-23.6558662522216,95.1707801321966,6.73837486430966));
#29203=CARTESIAN_POINT('Ctrl Pts',(-21.1565027813636,93.444575455666,6.58039169906103));
#29204=CARTESIAN_POINT('Ctrl Pts',(-21.2362883438098,90.4080915358129,6.42240853381239));
#29205=CARTESIAN_POINT('Ctrl Pts',(-23.822854709165,88.8155229275284,6.26442536856376));
#29206=CARTESIAN_POINT('Ctrl Pts',(-26.5700978999786,90.1113837173467,6.10644220331512));
#29207=CARTESIAN_POINT('Ctrl Pts',(-26.9861745724031,93.120283937885,5.94845903806649));
#29208=CARTESIAN_POINT('Ctrl Pts',(-24.6936889831954,95.1130483891543,5.79047587281785));
#29209=CARTESIAN_POINT('Ctrl Pts',(-21.7720038091006,94.2821716963994,5.63249270756922));
#29210=CARTESIAN_POINT('Ctrl Pts',(-20.8711872264541,91.3812873796306,5.47450954232059));
#29211=CARTESIAN_POINT('Ctrl Pts',(-22.8083106224958,89.0415965274887,5.31652637707195));
#29212=CARTESIAN_POINT('Ctrl Pts',(-25.8263369588428,89.3852786016259,5.15854321182332));
#29213=CARTESIAN_POINT('Ctrl Pts',(-27.1878133367392,92.1006022300214,5.00056004657468));
#29214=CARTESIAN_POINT('Ctrl Pts',(-25.6578342112759,94.7246762022458,4.84257688132605));
#29215=CARTESIAN_POINT('Ctrl Pts',(-22.6241428708219,94.8773758595294,4.68459371607741));
#29216=CARTESIAN_POINT('Ctrl Pts',(-20.8384009073378,92.4201974021612,4.52661055082878));
#29217=CARTESIAN_POINT('Ctrl Pts',(-21.9203372333551,89.5818855568597,4.36862738558014));
#29218=CARTESIAN_POINT('Ctrl Pts',(-24.8885986714499,88.9368860508676,4.21064422033151));
#29219=CARTESIAN_POINT('Ctrl Pts',(-27.0508707860238,91.0702354393139,4.05266105508288));
#29220=CARTESIAN_POINT('Ctrl Pts',(-26.4458989623376,94.0469130356406,3.89467788983424));
#29221=CARTESIAN_POINT('Ctrl Pts',(-23.6224133012983,95.1669706094549,3.73669472458561));
#29222=CARTESIAN_POINT('Ctrl Pts',(-21.1414116530791,93.4144778137314,3.57871155933697));
#29223=CARTESIAN_POINT('Ctrl Pts',(-21.2532472272103,90.3790052214256,3.42072839408834));
#29224=CARTESIAN_POINT('Ctrl Pts',(-23.8564812740058,88.8138305079731,3.2627452288397));
#29225=CARTESIAN_POINT('Ctrl Pts',(-26.5898917954034,90.1386196891669,3.10476206359107));
#29226=CARTESIAN_POINT('Ctrl Pts',(-26.9741818729016,93.1517455407258,2.94677889834244));
#29227=CARTESIAN_POINT('Ctrl Pts',(-24.6607878581825,95.1201964337696,2.7887957330938));
#29228=CARTESIAN_POINT('Ctrl Pts',(-21.7480359224623,94.2585276484937,2.63081256784516));
#29229=CARTESIAN_POINT('Ctrl Pts',(-20.8778938613744,91.3482870150165,2.47282940259653));
#29230=CARTESIAN_POINT('Ctrl Pts',(-22.8396053811238,89.0291930982614,2.31484623734789));
#29231=CARTESIAN_POINT('Ctrl Pts',(-25.8538410662937,89.4046799738415,2.15686307209927));
#29232=CARTESIAN_POINT('Ctrl Pts',(-27.1865660698866,92.1342974242998,1.99887990685063));
#29233=CARTESIAN_POINT('Ctrl Pts',(-25.6289945736719,94.7419254122381,1.84089674160199));
#29234=CARTESIAN_POINT('Ctrl Pts',(-22.5938128499926,94.8628951691849,1.68291357635336));
#29235=CARTESIAN_POINT('Ctrl Pts',(-20.8342063323051,92.3863825780119,1.52493041110472));
#29236=CARTESIAN_POINT('Ctrl Pts',(-21.9458469482259,89.5609167225542,1.36694724585609));
#29237=CARTESIAN_POINT('Ctrl Pts',(-24.9211501867667,88.9446903547357,1.20896408060745));
#29238=CARTESIAN_POINT('Ctrl Pts',(-27.0599483982647,91.1061061878422,1.05098091535882));
#29239=CARTESIAN_POINT('Ctrl Pts',(-26.6354960985062,93.076689807963,0.945658805193063));
#29240=CARTESIAN_POINT('Ctrl Pts',(-26.054331550342,93.7564253212269,0.892997750110186));
#29241=CARTESIAN_POINT('Ctrl Pts',(-24.6501999979751,89.5679131979649,10.3210067496694));
#29242=CARTESIAN_POINT('Ctrl Pts',(-25.4549268544596,89.7830508320407,10.2683456945866));
#29243=CARTESIAN_POINT('Ctrl Pts',(-26.8204146828804,91.0717162505807,10.1630235844208));
#29244=CARTESIAN_POINT('Ctrl Pts',(-26.3190518827217,93.859235701585,10.0050404191722));
#29245=CARTESIAN_POINT('Ctrl Pts',(-23.7101077647069,94.9559962729138,9.84705725392353));
#29246=CARTESIAN_POINT('Ctrl Pts',(-21.3661024340368,93.3736899805099,9.68907408867489));
#29247=CARTESIAN_POINT('Ctrl Pts',(-21.4101550062448,90.544366147193,9.53109092342626));
#29248=CARTESIAN_POINT('Ctrl Pts',(-23.8037637600975,89.0358580140619,9.37310775817763));
#29249=CARTESIAN_POINT('Ctrl Pts',(-26.3751312394447,90.2156800266326,9.21512459292898));
#29250=CARTESIAN_POINT('Ctrl Pts',(-26.7922883167697,93.0140625006431,9.05714142768037));
#29251=CARTESIAN_POINT('Ctrl Pts',(-24.67668841891,94.8925962568123,8.89915826243172));
#29252=CARTESIAN_POINT('Ctrl Pts',(-21.9473365304931,94.1474755724248,8.74117509718309));
#29253=CARTESIAN_POINT('Ctrl Pts',(-21.0798070037785,91.4545069990835,8.58319193193445));
#29254=CARTESIAN_POINT('Ctrl Pts',(-22.8609987914095,89.256326172624,8.42520876668581));
#29255=CARTESIAN_POINT('Ctrl Pts',(-25.6753003227576,89.5467477390427,8.26722560143719));
#29256=CARTESIAN_POINT('Ctrl Pts',(-26.9700488609232,92.0623545136228,8.10924243618855));
#29257=CARTESIAN_POINT('Ctrl Pts',(-25.5708609338593,94.5214027969798,7.95125927093991));
#29258=CARTESIAN_POINT('Ctrl Pts',(-22.746848902053,94.6934530836676,7.79327610569128));
#29259=CARTESIAN_POINT('Ctrl Pts',(-21.0594875031757,92.4224492937484,7.63529294044265));
#29260=CARTESIAN_POINT('Ctrl Pts',(-22.0392713958159,89.7682696714667,7.47730977519401));
#29261=CARTESIAN_POINT('Ctrl Pts',(-24.7975030118093,89.1383455838149,7.31932660994537));
#29262=CARTESIAN_POINT('Ctrl Pts',(-26.8323721974004,91.104039749101,7.16134344469675));
#29263=CARTESIAN_POINT('Ctrl Pts',(-26.2981831143418,93.8824004317056,7.0033602794481));
#29264=CARTESIAN_POINT('Ctrl Pts',(-23.6794635098851,94.95335967792,6.84537711419948));
#29265=CARTESIAN_POINT('Ctrl Pts',(-21.3514814400011,93.345520889057,6.68739394895083));
#29266=CARTESIAN_POINT('Ctrl Pts',(-21.4257961049051,90.5172487296326,6.5294107837022));
#29267=CARTESIAN_POINT('Ctrl Pts',(-23.8350015651438,89.0338825812615,6.37142761845357));
#29268=CARTESIAN_POINT('Ctrl Pts',(-26.3938662378477,90.2408861719505,6.21344445320493));
#29269=CARTESIAN_POINT('Ctrl Pts',(-26.7814125248905,93.0434660468493,6.0554612879563));
#29270=CARTESIAN_POINT('Ctrl Pts',(-24.6461227163573,94.8995866016016,5.89747812270766));
#29271=CARTESIAN_POINT('Ctrl Pts',(-21.9247775505004,94.125683139552,5.73949495745904));
#29272=CARTESIAN_POINT('Ctrl Pts',(-21.0857299781457,91.4237125158365,5.5815117922104));
#29273=CARTESIAN_POINT('Ctrl Pts',(-22.8900247858913,89.2444543101509,5.42352862696176));
#29274=CARTESIAN_POINT('Ctrl Pts',(-25.7011049986632,89.5645700978948,5.26554546171313));
#29275=CARTESIAN_POINT('Ctrl Pts',(-26.9692249153015,92.0937039331857,5.10756229646449));
#29276=CARTESIAN_POINT('Ctrl Pts',(-25.544156487718,94.5378451029737,4.94957913121586));
#29277=CARTESIAN_POINT('Ctrl Pts',(-22.7184854204702,94.6800741418382,4.79159596596723));
#29278=CARTESIAN_POINT('Ctrl Pts',(-21.055191817558,92.3913844582627,4.63361280071859));
#29279=CARTESIAN_POINT('Ctrl Pts',(-22.0629397490182,89.7476957104498,4.47562963546996));
#29280=CARTESIAN_POINT('Ctrl Pts',(-24.8276674435624,89.1469238329133,4.31764647022132));
#29281=CARTESIAN_POINT('Ctrl Pts',(-26.8416725179065,91.1339894130133,4.15966330497269));
#29282=CARTESIAN_POINT('Ctrl Pts',(-26.2781836237349,93.9065561696585,4.00168013972405));
#29283=CARTESIAN_POINT('Ctrl Pts',(-23.6483044284461,94.9498113742255,3.84369697447542));
#29284=CARTESIAN_POINT('Ctrl Pts',(-21.3374251106716,93.3174870430051,3.68571380922678));
#29285=CARTESIAN_POINT('Ctrl Pts',(-21.4415921173467,90.4901568643789,3.52773064397815));
#29286=CARTESIAN_POINT('Ctrl Pts',(-23.8663223557907,89.0323062109474,3.36974747872951));
#29287=CARTESIAN_POINT('Ctrl Pts',(-26.4123028654849,90.2662545726625,3.21176431348088));
#29288=CARTESIAN_POINT('Ctrl Pts',(-26.7702421650231,93.0727703269818,3.05378114823224));
#29289=CARTESIAN_POINT('Ctrl Pts',(-24.6154776221154,94.9062445046611,2.89579798298361));
#29290=CARTESIAN_POINT('Ctrl Pts',(-21.902453142307,94.103660364463,2.73781481773497));
#29291=CARTESIAN_POINT('Ctrl Pts',(-21.0919767389813,91.3929749868548,2.57983165248634));
#29292=CARTESIAN_POINT('Ctrl Pts',(-22.9191736623219,89.2329013843028,2.4218484872377));
#29293=CARTESIAN_POINT('Ctrl Pts',(-25.7267231489403,89.5826411176466,2.26386532198907));
#29294=CARTESIAN_POINT('Ctrl Pts',(-26.9680631735609,92.1250886473484,2.10588215674044));
#29295=CARTESIAN_POINT('Ctrl Pts',(-25.5172943846158,94.553911534307,1.9478989914918));
#29296=CARTESIAN_POINT('Ctrl Pts',(-22.690235129749,94.6665863927075,1.78991582624317));
#29297=CARTESIAN_POINT('Ctrl Pts',(-21.0512848646155,92.3598883172517,1.63193266099453));
#29298=CARTESIAN_POINT('Ctrl Pts',(-22.0867002622527,89.7281647095134,1.4739494957459));
#29299=CARTESIAN_POINT('Ctrl Pts',(-24.8579869008516,89.1541929955161,1.31596633049727));
#29300=CARTESIAN_POINT('Ctrl Pts',(-26.8501276781025,91.1674005036292,1.15798316524863));
#29301=CARTESIAN_POINT('Ctrl Pts',(-26.4547800806521,93.0028611672493,1.05266105508287));
#29302=CARTESIAN_POINT('Ctrl Pts',(-25.913465996665,93.635987203375,0.999999999999996));
#29303=CARTESIAN_POINT('Ctrl Pts',(-26.5149491154365,92.0017493991467,9.11258330249198));
#29304=CARTESIAN_POINT('Ctrl Pts',(-26.5168561491793,92.2947752403159,9.09410267755477));
#29305=CARTESIAN_POINT('Ctrl Pts',(-26.4695027538977,92.5872051880346,9.07562205261757));
#29306=CARTESIAN_POINT('Ctrl Pts',(-26.3701621542389,92.8607543810029,9.05714142768036));
#29307=CARTESIAN_POINT('Ctrl Pts',(-26.0870883508165,93.6402404193662,9.00448037259748));
#29308=CARTESIAN_POINT('Ctrl Pts',(-25.3818883848633,94.2664183380893,8.95181931751459));
#29309=CARTESIAN_POINT('Ctrl Pts',(-24.5743964204838,94.4553205167195,8.89915826243172));
#29310=CARTESIAN_POINT('Ctrl Pts',(-23.7669044561044,94.6442226953498,8.84649720734884));
#29311=CARTESIAN_POINT('Ctrl Pts',(-22.8571204932987,94.3958491338873,8.79383615226596));
#29312=CARTESIAN_POINT('Ctrl Pts',(-22.2576402574435,93.8228342575992,8.74117509718308));
#29313=CARTESIAN_POINT('Ctrl Pts',(-21.6581600215882,93.249819381311,8.68851404210021));
#29314=CARTESIAN_POINT('Ctrl Pts',(-21.3689835126833,92.3521631901972,8.63585298701733));
#29315=CARTESIAN_POINT('Ctrl Pts',(-21.5212605561694,91.5369716235638,8.58319193193445));
#29316=CARTESIAN_POINT('Ctrl Pts',(-21.6735375996555,90.7217800569303,8.53053087685157));
#29317=CARTESIAN_POINT('Ctrl Pts',(-22.2672681955325,89.9890531147772,8.47786982176869));
#29318=CARTESIAN_POINT('Ctrl Pts',(-23.0331837486957,89.6710932381037,8.42520876668581));
#29319=CARTESIAN_POINT('Ctrl Pts',(-23.7990993018589,89.3531333614303,8.37254771160294));
#29320=CARTESIAN_POINT('Ctrl Pts',(-24.7371998123082,89.4499405502364,8.31988665652006));
#29321=CARTESIAN_POINT('Ctrl Pts',(-25.4220414905605,89.9176119404029,8.26722560143718));
#29322=CARTESIAN_POINT('Ctrl Pts',(-26.0924008378476,90.375393494611,8.21567816845545));
#29323=CARTESIAN_POINT('Ctrl Pts',(-26.5200994141618,91.1885197854572,8.16413073547372));
#29324=CARTESIAN_POINT('Ctrl Pts',(-26.5215632327497,92.0003195913041,8.11258330249199));
#29325=CARTESIAN_POINT('Ctrl Pts',(-24.7937992825329,89.0307770462543,10.));
#29326=CARTESIAN_POINT('Ctrl Pts',(-24.8868524293128,89.0648163030121,10.));
#29327=CARTESIAN_POINT('Ctrl Pts',(-24.9778402996117,89.1036238816563,10.));
#29328=CARTESIAN_POINT('Ctrl Pts',(-25.0665543950931,89.146871551718,10.));
#29329=CARTESIAN_POINT('Ctrl Pts',(-25.1572341761829,89.19107748351,10.));
#29330=CARTESIAN_POINT('Ctrl Pts',(-25.2455389715748,89.2399230660525,10.));
#29331=CARTESIAN_POINT('Ctrl Pts',(-25.3312171949433,89.2931033029458,10.));
#29332=CARTESIAN_POINT('Ctrl Pts',(-25.413669686943,89.3442813372769,10.));
#29333=CARTESIAN_POINT('Ctrl Pts',(-25.4936899468709,89.3994746514444,10.));
#29334=CARTESIAN_POINT('Ctrl Pts',(-25.5710207513823,89.4584414877532,10.));
#29335=CARTESIAN_POINT('Ctrl Pts',(-25.6386852053297,89.5100374695235,10.));
#29336=CARTESIAN_POINT('Ctrl Pts',(-25.7042902544872,89.5645232522079,10.));
#29337=CARTESIAN_POINT('Ctrl Pts',(-25.7676389322598,89.6217495880626,10.));
#29338=CARTESIAN_POINT('Ctrl Pts',(-25.78173773919,89.6344858138041,10.));
#29339=CARTESIAN_POINT('Ctrl Pts',(-25.7957273872409,89.6473604851229,10.));
#29340=CARTESIAN_POINT('Ctrl Pts',(-25.8095862319979,89.6603535287235,10.));
#29341=CARTESIAN_POINT('Ctrl Pts',(-25.8820169439212,89.7282592895964,10.));
#29342=CARTESIAN_POINT('Ctrl Pts',(-25.950981982325,89.7994868058506,10.));
#29343=CARTESIAN_POINT('Ctrl Pts',(-26.0162414008611,89.8737454733438,10.));
#29344=CARTESIAN_POINT('Ctrl Pts',(-26.0811411487042,89.9475948716925,10.));
#29345=CARTESIAN_POINT('Ctrl Pts',(-26.1423764967775,90.0244428983472,10.));
#29346=CARTESIAN_POINT('Ctrl Pts',(-26.1996678356882,90.1040304952653,10.));
#29347=CARTESIAN_POINT('Ctrl Pts',(-26.2548606489779,90.1807028764735,10.));
#29348=CARTESIAN_POINT('Ctrl Pts',(-26.3063932593322,90.2599185451886,10.));
#29349=CARTESIAN_POINT('Ctrl Pts',(-26.3539707411373,90.341459492214,10.));
#29350=CARTESIAN_POINT('Ctrl Pts',(-26.3739595056633,90.3757173538636,10.));
#29351=CARTESIAN_POINT('Ctrl Pts',(-26.393249578895,90.4103857572883,10.));
#29352=CARTESIAN_POINT('Ctrl Pts',(-26.4118164862517,90.4454488350539,10.));
#29353=CARTESIAN_POINT('Ctrl Pts',(-26.4248530614507,90.4700680374454,10.));
#29354=CARTESIAN_POINT('Ctrl Pts',(-26.4375330823773,90.4948818175359,10.));
#29355=CARTESIAN_POINT('Ctrl Pts',(-26.4498475905638,90.5198846886023,10.));
#29356=CARTESIAN_POINT('Ctrl Pts',(-26.457600065583,90.5356249951102,10.));
#29357=CARTESIAN_POINT('Ctrl Pts',(-26.4652085570304,90.5514423659275,10.));
#29358=CARTESIAN_POINT('Ctrl Pts',(-26.4726611641404,90.5673143053848,10.));
#29359=CARTESIAN_POINT('Ctrl Pts',(-26.514781719135,90.6570191414131,10.));
#29360=CARTESIAN_POINT('Ctrl Pts',(-26.5520000635457,90.7486086651382,10.));
#29361=CARTESIAN_POINT('Ctrl Pts',(-26.5840245510355,90.8418104101182,10.));
#29362=CARTESIAN_POINT('Ctrl Pts',(-26.6138870174205,90.9287199657321,10.));
#29363=CARTESIAN_POINT('Ctrl Pts',(-26.6392330675846,91.0170321959346,10.));
#29364=CARTESIAN_POINT('Ctrl Pts',(-26.6597756784745,91.1065348612826,10.));
#29365=CARTESIAN_POINT('Ctrl Pts',(-26.6612629487393,91.11301478993,10.));
#29366=CARTESIAN_POINT('Ctrl Pts',(-26.6627250182667,91.1195009595951,10.));
#29367=CARTESIAN_POINT('Ctrl Pts',(-26.6641617673287,91.1259932900523,10.));
#29368=CARTESIAN_POINT('Ctrl Pts',(-26.6847473682253,91.2190147697362,10.));
#29369=CARTESIAN_POINT('Ctrl Pts',(-26.7001391868307,91.313301977244,10.));
#29370=CARTESIAN_POINT('Ctrl Pts',(-26.710414230246,91.4084468885593,10.));
#29371=CARTESIAN_POINT('Ctrl Pts',(-26.7162318667374,91.4623170753475,10.));
#29372=CARTESIAN_POINT('Ctrl Pts',(-26.7204082723903,91.5164620291722,10.));
#29373=CARTESIAN_POINT('Ctrl Pts',(-26.7229505321309,91.5708049958447,10.));
#29374=CARTESIAN_POINT('Ctrl Pts',(-26.7235978728721,91.5846424553929,10.));
#29375=CARTESIAN_POINT('Ctrl Pts',(-26.7241391083581,91.5984913477053,10.));
#29376=CARTESIAN_POINT('Ctrl Pts',(-26.7245741747786,91.6123381701919,10.));
#29377=CARTESIAN_POINT('Ctrl Pts',(-26.727502988299,91.7055532725557,10.));
#29378=CARTESIAN_POINT('Ctrl Pts',(-26.7256324130775,91.7988256455911,10.));
#29379=CARTESIAN_POINT('Ctrl Pts',(-26.7190973170402,91.8917800191792,10.));
#29380=CARTESIAN_POINT('Ctrl Pts',(-26.7125517832716,91.9848828577297,10.));
#29381=CARTESIAN_POINT('Ctrl Pts',(-26.701326437817,92.0776676598524,10.));
#29382=CARTESIAN_POINT('Ctrl Pts',(-26.6855058890497,92.169745200331,10.));
#29383=CARTESIAN_POINT('Ctrl Pts',(-26.6699125051892,92.2605006131003,10.));
#29384=CARTESIAN_POINT('Ctrl Pts',(-26.6498544727619,92.350569772881,10.));
#29385=CARTESIAN_POINT('Ctrl Pts',(-26.625369821818,92.4395547318735,10.));
#29386=CARTESIAN_POINT('Ctrl Pts',(-26.6161277488857,92.4731433455226,10.));
#29387=CARTESIAN_POINT('Ctrl Pts',(-26.606254568394,92.5065771589137,10.));
#29388=CARTESIAN_POINT('Ctrl Pts',(-26.5957509020014,92.5398334420584,10.));
#29389=CARTESIAN_POINT('Ctrl Pts',(-26.5880549567592,92.5642000322064,10.));
#29390=CARTESIAN_POINT('Ctrl Pts',(-26.5800205276971,92.5884713019318,10.));
#29391=CARTESIAN_POINT('Ctrl Pts',(-26.5716476123613,92.6126380143925,10.));
#29392=CARTESIAN_POINT('Ctrl Pts',(-26.5664801186219,92.627552931161,10.));
#29393=CARTESIAN_POINT('Ctrl Pts',(-26.5611866874407,92.6424193349119,10.));
#29394=CARTESIAN_POINT('Ctrl Pts',(-26.5557685057611,92.6572331361345,10.));
#29395=CARTESIAN_POINT('Ctrl Pts',(-26.5240624701884,92.7439203194567,10.));
#29396=CARTESIAN_POINT('Ctrl Pts',(-26.4880796645806,92.8288333308672,10.));
#29397=CARTESIAN_POINT('Ctrl Pts',(-26.4478803904145,92.9115713473252,10.));
#29398=CARTESIAN_POINT('Ctrl Pts',(-26.4177309347899,92.9736248596687,10.));
#29399=CARTESIAN_POINT('Ctrl Pts',(-26.3852087264707,93.034454452489,10.));
#29400=CARTESIAN_POINT('Ctrl Pts',(-26.3503241152161,93.0938760327216,10.));
#29401=CARTESIAN_POINT('Ctrl Pts',(-26.3345452312659,93.1207533916747,10.));
#29402=CARTESIAN_POINT('Ctrl Pts',(-26.3182828580768,93.1473424862479,10.));
#29403=CARTESIAN_POINT('Ctrl Pts',(-26.3015371730653,93.1736252114869,10.));
#29404=CARTESIAN_POINT('Ctrl Pts',(-26.2924151850266,93.1879423746897,10.));
#29405=CARTESIAN_POINT('Ctrl Pts',(-26.2831549587563,93.2021604667855,10.));
#29406=CARTESIAN_POINT('Ctrl Pts',(-26.2737571737911,93.2162764754243,10.));
#29407=CARTESIAN_POINT('Ctrl Pts',(-26.22618210498,93.2877369402902,10.));
#29408=CARTESIAN_POINT('Ctrl Pts',(-26.1750818283943,93.3565881459249,10.));
#29409=CARTESIAN_POINT('Ctrl Pts',(-26.1204874011636,93.422476604652,10.));
#29410=CARTESIAN_POINT('Ctrl Pts',(-26.0743569378935,93.4781501464292,10.));
#29411=CARTESIAN_POINT('Ctrl Pts',(-26.0257310846976,93.5317080232741,10.));
#29412=CARTESIAN_POINT('Ctrl Pts',(-25.974612285206,93.5829128576333,10.));
#29413=CARTESIAN_POINT('Ctrl Pts',(-25.9557804971257,93.6017763403232,10.));
#29414=CARTESIAN_POINT('Ctrl Pts',(-25.9366102390046,93.6203202358367,10.));
#29415=CARTESIAN_POINT('Ctrl Pts',(-25.9171116625783,93.6385402433575,10.));
#29416=CARTESIAN_POINT('Origin',(-24.,92.,5.));
#29417=CARTESIAN_POINT('Origin',(92.,24.,1.));
#29418=CARTESIAN_POINT('Ctrl Pts',(90.0865340033349,25.6359872033749,1.));
#29419=CARTESIAN_POINT('Ctrl Pts',(90.0243936537204,25.5775905334472,1.));
#29420=CARTESIAN_POINT('Ctrl Pts',(89.9656286004716,25.515940174112,1.));
#29421=CARTESIAN_POINT('Ctrl Pts',(89.9102508840482,25.4514125531291,1.));
#29422=CARTESIAN_POINT('Ctrl Pts',(89.8535184531324,25.385306381983,1.));
#29423=CARTESIAN_POINT('Ctrl Pts',(89.8003406478074,25.3161799622637,1.00000000000001));
#29424=CARTESIAN_POINT('Ctrl Pts',(89.750759301611,25.2443917537902,1.00000000000001));
#29425=CARTESIAN_POINT('Ctrl Pts',(89.7378154616087,25.2256505304105,1.00000000000001));
#29426=CARTESIAN_POINT('Ctrl Pts',(89.7251169046858,25.2067276793656,1.));
#29427=CARTESIAN_POINT('Ctrl Pts',(89.7126647511175,25.1876291447746,1.));
#29428=CARTESIAN_POINT('Ctrl Pts',(89.7025039315658,25.1720449518382,1.));
#29429=CARTESIAN_POINT('Ctrl Pts',(89.6925067437675,25.1563428868077,1.));
#29430=CARTESIAN_POINT('Ctrl Pts',(89.6826826227138,25.1405407390384,1.));
#29431=CARTESIAN_POINT('Ctrl Pts',(89.6352352786345,25.0642214491697,1.));
#29432=CARTESIAN_POINT('Ctrl Pts',(89.5917715087151,24.985494938699,1.));
#29433=CARTESIAN_POINT('Ctrl Pts',(89.5523260662542,24.9047536930622,1.));
#29434=CARTESIAN_POINT('Ctrl Pts',(89.5204851860134,24.8395782970616,1.));
#29435=CARTESIAN_POINT('Ctrl Pts',(89.4912631200874,24.7730890249891,1.));
#29436=CARTESIAN_POINT('Ctrl Pts',(89.4646953255791,24.7054744889604,1.));
#29437=CARTESIAN_POINT('Ctrl Pts',(89.4539704661986,24.6781799240781,1.));
#29438=CARTESIAN_POINT('Ctrl Pts',(89.4436783251344,24.6507018348571,1.));
#29439=CARTESIAN_POINT('Ctrl Pts',(89.433822025196,24.6230520618988,1.));
#29440=CARTESIAN_POINT('Ctrl Pts',(89.4286038515389,24.6084135750653,1.));
#29441=CARTESIAN_POINT('Ctrl Pts',(89.4235083975283,24.5937282955295,1.));
#29442=CARTESIAN_POINT('Ctrl Pts',(89.4185398830814,24.5790097971537,1.));
#29443=CARTESIAN_POINT('Ctrl Pts',(89.389025801749,24.4915786418671,1.));
#29444=CARTESIAN_POINT('Ctrl Pts',(89.3639479999348,24.4028676051837,1.));
#29445=CARTESIAN_POINT('Ctrl Pts',(89.3433392465014,24.3132743791318,1.));
#29446=CARTESIAN_POINT('Ctrl Pts',(89.3224115745818,24.2222947064846,1.));
#29447=CARTESIAN_POINT('Ctrl Pts',(89.3060918371883,24.1304045235307,1.));
#29448=CARTESIAN_POINT('Ctrl Pts',(89.2944561926122,24.0379871349153,1.00000000000001));
#29449=CARTESIAN_POINT('Ctrl Pts',(89.2829117117522,23.9462938241557,1.00000000000001));
#29450=CARTESIAN_POINT('Ctrl Pts',(89.2759778689656,23.8540806067861,1.00000000000001));
#29451=CARTESIAN_POINT('Ctrl Pts',(89.273776000804,23.7617026893423,1.00000000000001));
#29452=CARTESIAN_POINT('Ctrl Pts',(89.2726808058124,23.715754510296,1.00000000000001));
#29453=CARTESIAN_POINT('Ctrl Pts',(89.2727570661434,23.6697653722625,1.));
#29454=CARTESIAN_POINT('Ctrl Pts',(89.2740245029826,23.6237782920667,1.));
#29455=CARTESIAN_POINT('Ctrl Pts',(89.2744412788452,23.6086561933353,1.));
#29456=CARTESIAN_POINT('Ctrl Pts',(89.2749869695608,23.5935324657531,1.));
#29457=CARTESIAN_POINT('Ctrl Pts',(89.275662091735,23.5784144647086,1.));
#29458=CARTESIAN_POINT('Ctrl Pts',(89.2799360088404,23.4827087010319,1.));
#29459=CARTESIAN_POINT('Ctrl Pts',(89.2893769673482,23.3875701065554,1.));
#29460=CARTESIAN_POINT('Ctrl Pts',(89.3040491413972,23.2933970076216,1.));
#29461=CARTESIAN_POINT('Ctrl Pts',(89.3082037215585,23.266730905703,1.));
#29462=CARTESIAN_POINT('Ctrl Pts',(89.3127780329822,23.2401420872658,1.));
#29463=CARTESIAN_POINT('Ctrl Pts',(89.3177742468288,23.2136393367139,1.));
#29464=CARTESIAN_POINT('Ctrl Pts',(89.3347391581862,23.1236478296161,1.));
#29465=CARTESIAN_POINT('Ctrl Pts',(89.356564364113,23.034648784227,1.));
#29466=CARTESIAN_POINT('Ctrl Pts',(89.3829472265017,22.9468744390315,1.));
#29467=CARTESIAN_POINT('Ctrl Pts',(89.4099265677864,22.8571156410599,1.));
#29468=CARTESIAN_POINT('Ctrl Pts',(89.4416721888927,22.7686368463988,1.));
#29469=CARTESIAN_POINT('Ctrl Pts',(89.4779146987112,22.6816901122092,1.));
#29470=CARTESIAN_POINT('Ctrl Pts',(89.4905815187872,22.6513020777246,1.));
#29471=CARTESIAN_POINT('Ctrl Pts',(89.5037981010522,22.6211012696727,1.00000000000001));
#29472=CARTESIAN_POINT('Ctrl Pts',(89.5175543776716,22.5910988047463,1.00000000000001));
#29473=CARTESIAN_POINT('Ctrl Pts',(89.5245011977754,22.5759477771625,1.00000000000001));
#29474=CARTESIAN_POINT('Ctrl Pts',(89.5315856607301,22.5608473343647,1.));
#29475=CARTESIAN_POINT('Ctrl Pts',(89.5388065372973,22.5457989337137,1.));
#29476=CARTESIAN_POINT('Ctrl Pts',(89.5448162869273,22.5332745373471,1.));
#29477=CARTESIAN_POINT('Ctrl Pts',(89.5509186846871,22.5207901225854,1.00000000000001));
#29478=CARTESIAN_POINT('Ctrl Pts',(89.5571091315649,22.5083537155743,1.00000000000001));
#29479=CARTESIAN_POINT('Ctrl Pts',(89.6000723368599,22.4220420295041,1.00000000000001));
#29480=CARTESIAN_POINT('Ctrl Pts',(89.6473225868892,22.337937009213,1.00000000000001));
#29481=CARTESIAN_POINT('Ctrl Pts',(89.6985178128694,22.2562887342086,1.00000000000001));
#29482=CARTESIAN_POINT('Ctrl Pts',(89.7507178517981,22.1730379417357,1.00000000000001));
#29483=CARTESIAN_POINT('Ctrl Pts',(89.8070195603585,22.0923405044241,1.));
#29484=CARTESIAN_POINT('Ctrl Pts',(89.8671152472941,22.0144688397376,1.));
#29485=CARTESIAN_POINT('Ctrl Pts',(89.9276789696687,21.9359906972714,1.));
#29486=CARTESIAN_POINT('Ctrl Pts',(89.9920964595121,21.8603816769157,1.));
#29487=CARTESIAN_POINT('Ctrl Pts',(90.0601019298659,21.7879401973074,1.));
#29488=CARTESIAN_POINT('Ctrl Pts',(90.0970286042451,21.7486047892127,1.));
#29489=CARTESIAN_POINT('Ctrl Pts',(90.1350139823262,21.7102037246147,1.));
#29490=CARTESIAN_POINT('Ctrl Pts',(90.1740207522492,21.6727885370382,1.));
#29491=CARTESIAN_POINT('Ctrl Pts',(90.186150608565,21.6611536118642,1.));
#29492=CARTESIAN_POINT('Ctrl Pts',(90.1983792592015,21.6496140448139,1.));
#29493=CARTESIAN_POINT('Ctrl Pts',(90.2107056469257,21.6381714501822,1.));
#29494=CARTESIAN_POINT('Ctrl Pts',(90.2219939257138,21.627692532826,1.));
#29495=CARTESIAN_POINT('Ctrl Pts',(90.2333584433832,21.6173003008198,1.));
#29496=CARTESIAN_POINT('Ctrl Pts',(90.2447937623118,21.6069996110817,1.));
#29497=CARTESIAN_POINT('Ctrl Pts',(90.3206028376455,21.5387124238838,1.));
#29498=CARTESIAN_POINT('Ctrl Pts',(90.3995782020434,21.4743922574611,0.999999999999998));
#29499=CARTESIAN_POINT('Ctrl Pts',(90.4813936898827,21.4143217382276,0.999999999999999));
#29500=CARTESIAN_POINT('Ctrl Pts',(90.5632801177989,21.3541991334127,1.));
#29501=CARTESIAN_POINT('Ctrl Pts',(90.6480121733501,21.2983327113302,1.));
#29502=CARTESIAN_POINT('Ctrl Pts',(90.7353078050742,21.2470320374408,1.));
#29503=CARTESIAN_POINT('Ctrl Pts',(90.8208396632406,21.1967678732862,1.));
#29504=CARTESIAN_POINT('Ctrl Pts',(90.9088332163986,21.1508861489069,1.));
#29505=CARTESIAN_POINT('Ctrl Pts',(90.9990569161034,21.1097141762738,1.));
#29506=CARTESIAN_POINT('Ctrl Pts',(91.0368467525653,21.0924694598887,1.00000000000001));
#29507=CARTESIAN_POINT('Ctrl Pts',(91.0750281840494,21.0760514837458,1.));
#29508=CARTESIAN_POINT('Ctrl Pts',(91.1135855898122,21.0604866736419,1.));
#29509=CARTESIAN_POINT('Ctrl Pts',(91.1435992944683,21.0483707751719,1.));
#29510=CARTESIAN_POINT('Ctrl Pts',(91.1738408319515,21.0367718698255,1.));
#29511=CARTESIAN_POINT('Ctrl Pts',(91.2042984301044,21.0256873776386,1.));
#29512=CARTESIAN_POINT('Ctrl Pts',(92.7937992825329,21.0307770462543,1.));
#29513=CARTESIAN_POINT('Ctrl Pts',(92.8886355471641,21.0654685754872,1.));
#29514=CARTESIAN_POINT('Ctrl Pts',(92.981428580578,21.1051505313063,1.00000000000001));
#29515=CARTESIAN_POINT('Ctrl Pts',(93.0719374504447,21.1495026644839,1.));
#29516=CARTESIAN_POINT('Ctrl Pts',(93.1637178577445,21.1944778901568,1.));
#29517=CARTESIAN_POINT('Ctrl Pts',(93.2531501397529,21.2442561370497,1.));
#29518=CARTESIAN_POINT('Ctrl Pts',(93.3399490406757,21.2985441485801,0.999999999999999));
#29519=CARTESIAN_POINT('Ctrl Pts',(93.3644577825898,21.3138730392628,0.999999999999999));
#29520=CARTESIAN_POINT('Ctrl Pts',(93.3887563291026,21.3295616963359,1.));
#29521=CARTESIAN_POINT('Ctrl Pts',(93.4128376624865,21.3456039733805,1.));
#29522=CARTESIAN_POINT('Ctrl Pts',(93.4321684182458,21.3584815551335,1.));
#29523=CARTESIAN_POINT('Ctrl Pts',(93.4513613131721,21.3715886263023,1.));
#29524=CARTESIAN_POINT('Ctrl Pts',(93.4703934284029,21.3849082414666,1.));
#29525=CARTESIAN_POINT('Ctrl Pts',(93.5531010557067,21.4427911280235,1.));
#29526=CARTESIAN_POINT('Ctrl Pts',(93.6328538471322,21.5047358078477,1.));
#29527=CARTESIAN_POINT('Ctrl Pts',(93.7093854474969,21.5704450409762,1.));
#29528=CARTESIAN_POINT('Ctrl Pts',(93.7683982885621,21.6211128502557,1.));
#29529=CARTESIAN_POINT('Ctrl Pts',(93.8254952341963,21.6740199048097,1.));
#29530=CARTESIAN_POINT('Ctrl Pts',(93.8805365802951,21.7290417093972,1.));
#29531=CARTESIAN_POINT('Ctrl Pts',(93.9098566848023,21.7583514042907,1.));
#29532=CARTESIAN_POINT('Ctrl Pts',(93.9385932130282,21.7882613322448,1.));
#29533=CARTESIAN_POINT('Ctrl Pts',(93.966723018163,21.8187535093172,1.));
#29534=CARTESIAN_POINT('Ctrl Pts',(93.9763569992674,21.8291965627383,1.));
#29535=CARTESIAN_POINT('Ctrl Pts',(93.9859190158138,21.8397071306493,1.));
#29536=CARTESIAN_POINT('Ctrl Pts',(93.9954015810245,21.8502769624256,1.));
#29537=CARTESIAN_POINT('Ctrl Pts',(94.0611940655502,21.9236131829668,1.));
#29538=CARTESIAN_POINT('Ctrl Pts',(94.1232543001003,21.9998957526439,1.));
#29539=CARTESIAN_POINT('Ctrl Pts',(94.1813384939113,22.0788462503669,1.));
#29540=CARTESIAN_POINT('Ctrl Pts',(94.2389162823979,22.1571084205125,1.));
#29541=CARTESIAN_POINT('Ctrl Pts',(94.2925874949548,22.2379929849892,1.));
#29542=CARTESIAN_POINT('Ctrl Pts',(94.3420688574455,22.3212511467048,0.999999999999999));
#29543=CARTESIAN_POINT('Ctrl Pts',(94.390117240581,22.4020981535756,0.999999999999999));
#29544=CARTESIAN_POINT('Ctrl Pts',(94.4342151409803,22.4851839694888,1.));
#29545=CARTESIAN_POINT('Ctrl Pts',(94.4740553951334,22.57029111177,1.));
#29546=CARTESIAN_POINT('Ctrl Pts',(94.4948666592991,22.6147483387141,1.));
#29547=CARTESIAN_POINT('Ctrl Pts',(94.5145153291242,22.6597572305835,1.));
#29548=CARTESIAN_POINT('Ctrl Pts',(94.532951917645,22.7052870236586,1.));
#29549=CARTESIAN_POINT('Ctrl Pts',(94.5400925813619,22.7229211397036,1.));
#29550=CARTESIAN_POINT('Ctrl Pts',(94.5470513788846,22.7406333941673,0.999999999999999));
#29551=CARTESIAN_POINT('Ctrl Pts',(94.5538252664571,22.7584219905631,0.999999999999999));
#29552=CARTESIAN_POINT('Ctrl Pts',(94.5589791553681,22.7719563825541,0.999999999999999));
#29553=CARTESIAN_POINT('Ctrl Pts',(94.5640259616331,22.7855350879592,0.999999999999999));
#29554=CARTESIAN_POINT('Ctrl Pts',(94.5689595142746,22.7991434114529,1.));
#29555=CARTESIAN_POINT('Ctrl Pts',(94.6006313710319,22.8865045695715,1.));
#29556=CARTESIAN_POINT('Ctrl Pts',(94.6276945170064,22.9752266495777,1.));
#29557=CARTESIAN_POINT('Ctrl Pts',(94.6498976668917,23.0650862424225,1.));
#29558=CARTESIAN_POINT('Ctrl Pts',(94.6549002608062,23.0853325162461,1.));
#29559=CARTESIAN_POINT('Ctrl Pts',(94.659655933924,23.1056365754165,1.));
#29560=CARTESIAN_POINT('Ctrl Pts',(94.6641614464107,23.1259959208575,1.));
#29561=CARTESIAN_POINT('Ctrl Pts',(94.684506977676,23.2179325652312,1.));
#29562=CARTESIAN_POINT('Ctrl Pts',(94.6997555099893,23.3109969010515,0.999999999999998));
#29563=CARTESIAN_POINT('Ctrl Pts',(94.7100169526532,23.4047971880022,0.999999999999998));
#29564=CARTESIAN_POINT('Ctrl Pts',(94.7207301009448,23.5027265354449,0.999999999999998));
#29565=CARTESIAN_POINT('Ctrl Pts',(94.7260074241417,23.6014592922061,0.999999999999998));
#29566=CARTESIAN_POINT('Ctrl Pts',(94.7259165033721,23.7005349801267,0.999999999999998));
#29567=CARTESIAN_POINT('Ctrl Pts',(94.72588138918,23.7387986546096,0.999999999999998));
#29568=CARTESIAN_POINT('Ctrl Pts',(94.7250449852703,23.7771132264404,0.999999999999997));
#29569=CARTESIAN_POINT('Ctrl Pts',(94.7234090502602,23.8154509913219,0.999999999999997));
#29570=CARTESIAN_POINT('Ctrl Pts',(94.7228214486292,23.8292213019001,0.999999999999996));
#29571=CARTESIAN_POINT('Ctrl Pts',(94.7221307047809,23.8429928066208,0.999999999999999));
#29572=CARTESIAN_POINT('Ctrl Pts',(94.7213377902191,23.8567525532216,0.999999999999999));
#29573=CARTESIAN_POINT('Ctrl Pts',(94.7159861969755,23.9496207769742,1.));
#29574=CARTESIAN_POINT('Ctrl Pts',(94.7059788948869,24.042101901153,0.999999999999996));
#29575=CARTESIAN_POINT('Ctrl Pts',(94.6914389407265,24.1338240294237,0.999999999999997));
#29576=CARTESIAN_POINT('Ctrl Pts',(94.6769360336291,24.2253124543804,0.999999999999997));
#29577=CARTESIAN_POINT('Ctrl Pts',(94.6579231315279,24.3160466905483,1.));
#29578=CARTESIAN_POINT('Ctrl Pts',(94.634473763784,24.4056405654129,1.));
#29579=CARTESIAN_POINT('Ctrl Pts',(94.6114256905903,24.4937011992063,1.));
#29580=CARTESIAN_POINT('Ctrl Pts',(94.5840912290588,24.5806609515592,0.999999999999999));
#29581=CARTESIAN_POINT('Ctrl Pts',(94.5524998627482,24.6661239164516,0.999999999999999));
#29582=CARTESIAN_POINT('Ctrl Pts',(94.5366373928654,24.7090360745829,0.999999999999999));
#29583=CARTESIAN_POINT('Ctrl Pts',(94.5197010824682,24.7515703293015,1.));
#29584=CARTESIAN_POINT('Ctrl Pts',(94.5016912752121,24.7936727822635,1.));
#29585=CARTESIAN_POINT('Ctrl Pts',(94.4963919593661,24.8060612655474,1.));
#29586=CARTESIAN_POINT('Ctrl Pts',(94.4909996852932,24.8184123442166,1.));
#29587=CARTESIAN_POINT('Ctrl Pts',(94.4855144272657,24.830724596362,1.));
#29588=CARTESIAN_POINT('Ctrl Pts',(94.4799210126452,24.8432796176239,1.));
#29589=CARTESIAN_POINT('Ctrl Pts',(94.4742345911846,24.855785977545,0.999999999999998));
#29590=CARTESIAN_POINT('Ctrl Pts',(94.4684564518667,24.8682403411912,0.999999999999998));
#29591=CARTESIAN_POINT('Ctrl Pts',(94.4309710840811,24.9490373549233,0.999999999999997));
#29592=CARTESIAN_POINT('Ctrl Pts',(94.3896160117749,25.0276775108318,1.));
#29593=CARTESIAN_POINT('Ctrl Pts',(94.3444610578896,25.1038131056636,1.));
#29594=CARTESIAN_POINT('Ctrl Pts',(94.3000642811839,25.1786703408565,0.999999999999999));
#29595=CARTESIAN_POINT('Ctrl Pts',(94.2519937015338,25.2511070843615,0.999999999999999));
#29596=CARTESIAN_POINT('Ctrl Pts',(94.2002794828524,25.3207586726253,0.999999999999999));
#29597=CARTESIAN_POINT('Ctrl Pts',(94.1501451979328,25.3882823181555,1.));
#29598=CARTESIAN_POINT('Ctrl Pts',(94.0965860653805,25.4531888295719,0.999999999999999));
#29599=CARTESIAN_POINT('Ctrl Pts',(94.0396018763204,25.5151056720679,0.999999999999999));
#29600=CARTESIAN_POINT('Ctrl Pts',(94.0184128643754,25.5381288428261,0.999999999999999));
#29601=CARTESIAN_POINT('Ctrl Pts',(93.9967500378537,25.5607382046462,0.999999999999998));
#29602=CARTESIAN_POINT('Ctrl Pts',(93.9746125472696,25.5829129376406,0.999999999999998));
#29603=CARTESIAN_POINT('Ctrl Pts',(93.9557857592068,25.6017713984427,0.999999999999998));
#29604=CARTESIAN_POINT('Ctrl Pts',(93.936615643811,25.6203154841753,0.999999999999998));
#29605=CARTESIAN_POINT('Ctrl Pts',(93.9171119325403,25.6385402784441,0.999999999999998));
#29606=CARTESIAN_POINT('Origin',(92.,24.,12.2084234471775));
#29607=CARTESIAN_POINT('Ctrl Pts',(88.9232326966468,24.0019373937314,9.70842344717745));
#29608=CARTESIAN_POINT('Ctrl Pts',(88.9222985312732,24.1261020010043,9.70197366100993));
#29609=CARTESIAN_POINT('Ctrl Pts',(88.9853329189178,25.263114277285,9.64286281975953));
#29610=CARTESIAN_POINT('Ctrl Pts',(90.4009679157595,27.2555128800837,9.53109092342627));
#29611=CARTESIAN_POINT('Ctrl Pts',(93.8523952892238,27.1179538105414,9.37310775817762));
#29612=CARTESIAN_POINT('Ctrl Pts',(95.6235723677572,24.1527148994824,9.215124592929));
#29613=CARTESIAN_POINT('Ctrl Pts',(94.1080772256066,21.0487573061686,9.05714142768035));
#29614=CARTESIAN_POINT('Ctrl Pts',(90.6804686178369,20.6217759976464,8.89915826243173));
#29615=CARTESIAN_POINT('Ctrl Pts',(89.0391555349924,22.5621016925695,8.78291893559742));
#29616=CARTESIAN_POINT('Ctrl Pts',(88.9237201879855,23.7866862070449,8.719340663846));
#29617=CARTESIAN_POINT('Ctrl Pts',(88.925632029797,23.9973209161002,8.70842344717745));
#29618=CARTESIAN_POINT('Ctrl Pts',(88.929711085108,23.9968960951897,9.79157655282255));
#29619=CARTESIAN_POINT('Ctrl Pts',(88.9347146766408,24.6903800819212,9.75572892504928));
#29620=CARTESIAN_POINT('Ctrl Pts',(89.5077563627456,26.4123579721077,9.66722024219312));
#29621=CARTESIAN_POINT('Ctrl Pts',(92.3539160756187,27.6088391884301,9.5260505042541));
#29622=CARTESIAN_POINT('Ctrl Pts',(95.2156041936735,25.6770751085581,9.36806733900546));
#29623=CARTESIAN_POINT('Ctrl Pts',(95.1618224985938,22.2228835192268,9.21008417375683));
#29624=CARTESIAN_POINT('Ctrl Pts',(92.2395757642924,20.3812156575975,9.05210100850819));
#29625=CARTESIAN_POINT('Ctrl Pts',(89.4675379096604,21.6531112748897,8.91259846819677));
#29626=CARTESIAN_POINT('Ctrl Pts',(88.9339205520176,23.3404824212939,8.82575698296822));
#29627=CARTESIAN_POINT('Ctrl Pts',(88.9296144608475,24.002135757227,8.79157655282255));
#29628=CARTESIAN_POINT('Ctrl Pts',(93.9134659966651,25.6359872033749,10.));
#29629=CARTESIAN_POINT('Ctrl Pts',(94.4547800806522,25.0028611672492,9.94733894491712));
#29630=CARTESIAN_POINT('Ctrl Pts',(94.850124624194,23.1673972202025,9.84201683475137));
#29631=CARTESIAN_POINT('Ctrl Pts',(92.8579881232768,21.154193771773,9.68403366950273));
#29632=CARTESIAN_POINT('Ctrl Pts',(90.0866994468077,21.7281636060897,9.5260505042541));
#29633=CARTESIAN_POINT('Ctrl Pts',(89.0512846745644,24.3598888261915,9.36806733900546));
#29634=CARTESIAN_POINT('Ctrl Pts',(90.6902348228159,26.6665865220793,9.21008417375683));
#29635=CARTESIAN_POINT('Ctrl Pts',(93.5172946610121,26.5539120605297,9.0521010085082));
#29636=CARTESIAN_POINT('Ctrl Pts',(94.9680635873854,24.1250885828687,8.89411784325955));
#29637=CARTESIAN_POINT('Ctrl Pts',(93.726723414825,21.5826408063378,8.73613467801094));
#29638=CARTESIAN_POINT('Ctrl Pts',(90.9191734977728,21.2329009513827,8.57815151276228));
#29639=CARTESIAN_POINT('Ctrl Pts',(89.0919763121477,23.3929749104686,8.42016834751366));
#29640=CARTESIAN_POINT('Ctrl Pts',(89.9024528317436,26.1036606678714,8.26218518226502));
#29641=CARTESIAN_POINT('Ctrl Pts',(92.6154777134031,26.906244937241,8.10420201701639));
#29642=CARTESIAN_POINT('Ctrl Pts',(94.7702425736134,25.0727704833333,7.94621885176775));
#29643=CARTESIAN_POINT('Ctrl Pts',(94.4123032215513,22.2662543178418,7.78823568651912));
#29644=CARTESIAN_POINT('Ctrl Pts',(91.866322336025,21.0323057724808,7.63025252127049));
#29645=CARTESIAN_POINT('Ctrl Pts',(89.441591739827,22.4901566418531,7.47226935602184));
#29646=CARTESIAN_POINT('Ctrl Pts',(89.3374247177566,25.3174872372792,7.31428619077322));
#29647=CARTESIAN_POINT('Ctrl Pts',(91.6483043765505,26.9498118095941,7.15630302552458));
#29648=CARTESIAN_POINT('Ctrl Pts',(94.2781839599183,25.906556450965,6.99831986027594));
#29649=CARTESIAN_POINT('Ctrl Pts',(94.8416729372438,23.1339892852383,6.84033669502732));
#29650=CARTESIAN_POINT('Ctrl Pts',(92.8276675656984,21.1469234118836,6.68235352977867));
#29651=CARTESIAN_POINT('Ctrl Pts',(90.0629394631723,21.7476953780895,6.52437036453004));
#29652=CARTESIAN_POINT('Ctrl Pts',(89.0551913830017,24.3913845160155,6.36638719928141));
#29653=CARTESIAN_POINT('Ctrl Pts',(90.7184852313611,26.6800745373299,6.20840403403277));
#29654=CARTESIAN_POINT('Ctrl Pts',(93.5441567155844,26.537845477475,6.05042086878414));
#29655=CARTESIAN_POINT('Ctrl Pts',(94.9692253534609,24.0937039470136,5.8924377035355));
#29656=CARTESIAN_POINT('Ctrl Pts',(93.70110524969,21.5645697385057,5.73445453828687));
#29657=CARTESIAN_POINT('Ctrl Pts',(90.8900246220956,21.2444539035236,5.57647137303823));
#29658=CARTESIAN_POINT('Ctrl Pts',(89.0857295480959,23.4237124307955,5.4184882077896));
#29659=CARTESIAN_POINT('Ctrl Pts',(89.9247772442662,26.1256834532325,5.26050504254097));
#29660=CARTESIAN_POINT('Ctrl Pts',(92.6461228117038,26.8995870294848,5.10252187729233));
#29661=CARTESIAN_POINT('Ctrl Pts',(94.781412935335,25.0434662008304,4.9445387120437));
#29662=CARTESIAN_POINT('Ctrl Pts',(94.393866591103,22.2408859123632,4.78655554679506));
#29663=CARTESIAN_POINT('Ctrl Pts',(91.8350015407957,21.0338821435613,4.62857238154643));
#29664=CARTESIAN_POINT('Ctrl Pts',(89.4257957250371,22.5172485108266,4.4705892162978));
#29665=CARTESIAN_POINT('Ctrl Pts',(89.3514810491689,25.3455210876135,4.31260605104916));
#29666=CARTESIAN_POINT('Ctrl Pts',(91.6794634625817,26.953360113734,4.15462288580053));
#29667=CARTESIAN_POINT('Ctrl Pts',(94.2981834534832,25.8824007094939,3.99663972055189));
#29668=CARTESIAN_POINT('Ctrl Pts',(94.8323726153541,23.1040396168705,3.83865655530326));
#29669=CARTESIAN_POINT('Ctrl Pts',(92.797503129515,21.1383451615613,3.68067339005462));
#29670=CARTESIAN_POINT('Ctrl Pts',(90.0392711064376,21.7682693420746,3.52269022480599));
#29671=CARTESIAN_POINT('Ctrl Pts',(89.0594870693288,24.4224493562101,3.36470705955735));
#29672=CARTESIAN_POINT('Ctrl Pts',(90.7468487169863,26.6934534808945,3.20672389430872));
#29673=CARTESIAN_POINT('Ctrl Pts',(93.5708611659363,26.521403169517,3.04874072906008));
#29674=CARTESIAN_POINT('Ctrl Pts',(94.9700492986991,24.0623545219302,2.89075756381145));
#29675=CARTESIAN_POINT('Ctrl Pts',(93.6753005709137,21.5467473787504,2.73277439856282));
#29676=CARTESIAN_POINT('Ctrl Pts',(90.8609986216085,21.2563257644251,2.57479123331418));
#29677=CARTESIAN_POINT('Ctrl Pts',(89.0798065759794,23.4545069249601,2.41680806806555));
#29678=CARTESIAN_POINT('Ctrl Pts',(89.947336222007,26.1474758771512,2.25882490281691));
#29679=CARTESIAN_POINT('Ctrl Pts',(92.6766885285289,26.8925967067901,2.10084173756828));
#29680=CARTESIAN_POINT('Ctrl Pts',(94.7922887122239,25.0140626065851,1.94285857231964));
#29681=CARTESIAN_POINT('Ctrl Pts',(94.3751316170022,22.215679845363,1.78487540707101));
#29682=CARTESIAN_POINT('Ctrl Pts',(91.8037636898017,21.0358574238383,1.62689224182237));
#29683=CARTESIAN_POINT('Ctrl Pts',(89.410154680019,22.5443662144373,1.46890907657374));
#29684=CARTESIAN_POINT('Ctrl Pts',(89.3661019891307,25.3736896687445,1.3109259113251));
#29685=CARTESIAN_POINT('Ctrl Pts',(91.7101077177225,26.9559976441494,1.15294274607647));
#29686=CARTESIAN_POINT('Ctrl Pts',(94.3190524504204,25.8592343694376,0.994959580827835));
#29687=CARTESIAN_POINT('Ctrl Pts',(94.8204140260176,23.0717206863195,0.836976415579202));
#29688=CARTESIAN_POINT('Ctrl Pts',(93.4549268544596,21.7830508320407,0.731654305413445));
#29689=CARTESIAN_POINT('Ctrl Pts',(92.6501999979751,21.5679131979649,0.678993250330566));
#29690=CARTESIAN_POINT('Ctrl Pts',(94.0543315503421,25.7564253212268,10.1070022498898));
#29691=CARTESIAN_POINT('Ctrl Pts',(94.6354960985062,25.0766898079629,10.0543411948069));
#29692=CARTESIAN_POINT('Ctrl Pts',(95.0599451195336,23.1061026626961,9.94901908464117));
#29693=CARTESIAN_POINT('Ctrl Pts',(92.9211514991843,20.9446911881392,9.79103591939255));
#29694=CARTESIAN_POINT('Ctrl Pts',(89.9458460727495,21.5609155378985,9.63305275414391));
#29695=CARTESIAN_POINT('Ctrl Pts',(88.834206128263,24.3863831244189,9.47506958889527));
#29696=CARTESIAN_POINT('Ctrl Pts',(90.5938125204637,26.8628953080808,9.31708642364664));
#29697=CARTESIAN_POINT('Ctrl Pts',(93.628994870416,26.7419259772002,9.159103258398));
#29698=CARTESIAN_POINT('Ctrl Pts',(95.1865665141759,24.1342973550732,9.00112009314937));
#29699=CARTESIAN_POINT('Ctrl Pts',(93.8538413517522,21.4046796396148,8.84313692790074));
#29700=CARTESIAN_POINT('Ctrl Pts',(90.8396052044608,21.0291926334706,8.6851537626521));
#29701=CARTESIAN_POINT('Ctrl Pts',(88.8778934031181,23.348286933007,8.52717059740347));
#29702=CARTESIAN_POINT('Ctrl Pts',(89.7480355890358,26.2585279742383,8.36918743215483));
#29703=CARTESIAN_POINT('Ctrl Pts',(92.6607879561905,27.1201968981952,8.2112042669062));
#29704=CARTESIAN_POINT('Ctrl Pts',(94.9741823115716,25.1517457085876,8.05322110165757));
#29705=CARTESIAN_POINT('Ctrl Pts',(94.5898921776827,22.1386194155869,7.89523793640892));
#29706=CARTESIAN_POINT('Ctrl Pts',(91.8564812527851,20.8138300372275,7.7372547711603));
#29707=CARTESIAN_POINT('Ctrl Pts',(89.2532468218983,22.3790049825178,7.57927160591166));
#29708=CARTESIAN_POINT('Ctrl Pts',(89.1414112312387,25.4144780223077,7.42128844066303));
#29709=CARTESIAN_POINT('Ctrl Pts',(91.6224132455821,27.1669710768744,7.26330527541439));
#29710=CARTESIAN_POINT('Ctrl Pts',(94.4458993232702,26.0469133376563,7.10532211016575));
#29711=CARTESIAN_POINT('Ctrl Pts',(95.0508712362317,23.0702353021324,6.94733894491713));
#29712=CARTESIAN_POINT('Ctrl Pts',(92.8885988025775,20.9368855988426,6.78935577966848));
#29713=CARTESIAN_POINT('Ctrl Pts',(89.9203369264657,21.5818852000316,6.63137261441985));
#29714=CARTESIAN_POINT('Ctrl Pts',(88.8384004407904,24.4201974641658,6.47338944917122));
#29715=CARTESIAN_POINT('Ctrl Pts',(90.624142667791,26.8773762841363,6.31540628392259));
#29716=CARTESIAN_POINT('Ctrl Pts',(93.6578344559174,26.7246766043172,6.15742311867394));
#29717=CARTESIAN_POINT('Ctrl Pts',(95.1878138071549,24.1006022448672,5.99943995342532));
#29718=CARTESIAN_POINT('Ctrl Pts',(93.8263372283497,21.3852782157794,5.84145678817669));
#29719=CARTESIAN_POINT('Ctrl Pts',(90.8083104466419,21.0415960909264,5.68347362292804));
#29720=CARTESIAN_POINT('Ctrl Pts',(88.8711867647448,23.3812872883291,5.52549045767941));
#29721=CARTESIAN_POINT('Ctrl Pts',(89.7720034803222,26.2821720331725,5.36750729243078));
#29722=CARTESIAN_POINT('Ctrl Pts',(92.693689085561,27.1130488485372,5.20952412718214));
#29723=CARTESIAN_POINT('Ctrl Pts',(94.9861750130637,25.120284103202,5.05154096193351));
#29724=CARTESIAN_POINT('Ctrl Pts',(94.5700982792398,22.1113834386491,4.89355779668487));
#29725=CARTESIAN_POINT('Ctrl Pts',(91.8228546830244,20.8155224576056,4.73557463143624));
#29726=CARTESIAN_POINT('Ctrl Pts',(89.2362879359766,22.4080913008987,4.57759146618761));
#29727=CARTESIAN_POINT('Ctrl Pts',(89.1565023617591,25.4445756688399,4.41960830093897));
#29728=CARTESIAN_POINT('Ctrl Pts',(91.6558662014358,27.1707806000943,4.26162513569034));
#29729=CARTESIAN_POINT('Ctrl Pts',(94.4673711396979,26.0209792986337,4.1036419704417));
#29730=CARTESIAN_POINT('Ctrl Pts',(95.0408862431775,23.0380807988606,3.94565880519307));
#29731=CARTESIAN_POINT('Ctrl Pts',(92.8562137207113,20.9276758348255,3.78767563994443));
#29732=CARTESIAN_POINT('Ctrl Pts',(89.8949261524727,21.6039737782472,3.6296924746958));
#29733=CARTESIAN_POINT('Ctrl Pts',(88.8430123669848,24.4535492359919,3.47170930944716));
#29734=CARTESIAN_POINT('Ctrl Pts',(90.6545942167075,26.8917401588657,3.31372614419853));
#29735=CARTESIAN_POINT('Ctrl Pts',(93.6865048346898,26.7070238464122,3.15574297894989));
#29736=CARTESIAN_POINT('Ctrl Pts',(95.1886984095997,24.0669449375797,2.99775981370126));
#29737=CARTESIAN_POINT('Ctrl Pts',(93.7986328605434,21.3661438094138,2.83977664845263));
#29738=CARTESIAN_POINT('Ctrl Pts',(90.7771476098394,21.0543419345702,2.68179348320399));
#29739=CARTESIAN_POINT('Ctrl Pts',(88.864827755224,23.4143488117893,2.52381031795536));
#29740=CARTESIAN_POINT('Ctrl Pts',(89.7962232050506,26.305568771914,2.36582715270672));
#29741=CARTESIAN_POINT('Ctrl Pts',(92.72650498955,27.1055439122155,2.20784398745809));
#29742=CARTESIAN_POINT('Ctrl Pts',(94.9978514429748,25.0887158749415,2.04986082220945));
#29743=CARTESIAN_POINT('Ctrl Pts',(94.5499840736793,22.0843217512249,1.89187765696082));
#29744=CARTESIAN_POINT('Ctrl Pts',(91.7893171636885,20.8176431540805,1.73389449171218));
#29745=CARTESIAN_POINT('Ctrl Pts',(89.2194954283924,22.4372053558113,1.57591132646355));
#29746=CARTESIAN_POINT('Ctrl Pts',(89.1721996661856,25.4748179647818,1.41792816121491));
#29747=CARTESIAN_POINT('Ctrl Pts',(91.6887664255746,27.173612300243,1.25994499596628));
#29748=CARTESIAN_POINT('Ctrl Pts',(94.4897764706037,25.9961074987865,1.10196183071765));
#29749=CARTESIAN_POINT('Ctrl Pts',(95.0280472863242,23.0033826130449,0.943978665469013));
#29750=CARTESIAN_POINT('Ctrl Pts',(93.5620356702265,21.6198434520492,0.838656555303256));
#29751=CARTESIAN_POINT('Ctrl Pts',(92.698066426161,21.3888678140614,0.785995500220377));
#29752=CARTESIAN_POINT('Ctrl Pts',(94.1951971040191,25.8768634390787,10.2140044997796));
#29753=CARTESIAN_POINT('Ctrl Pts',(94.8162121163602,25.1505184486767,10.1613434446967));
#29754=CARTESIAN_POINT('Ctrl Pts',(95.2697656148731,23.0448081051897,10.056021334531));
#29755=CARTESIAN_POINT('Ctrl Pts',(92.9843148750919,20.7351886045054,9.89803816928235));
#29756=CARTESIAN_POINT('Ctrl Pts',(89.8049926986913,21.3936674697073,9.74005500403372));
#29757=CARTESIAN_POINT('Ctrl Pts',(88.6171275819614,24.4128774226463,9.58207183878508));
#29758=CARTESIAN_POINT('Ctrl Pts',(90.4973902181116,27.0592040940823,9.42408867353646));
#29759=CARTESIAN_POINT('Ctrl Pts',(93.7406950798199,26.9299398938708,9.26610550828781));
#29760=CARTESIAN_POINT('Ctrl Pts',(95.4050694409666,24.1435061272778,9.10812234303919));
#29761=CARTESIAN_POINT('Ctrl Pts',(93.9809592886795,21.2267184728917,8.95013917779054));
#29762=CARTESIAN_POINT('Ctrl Pts',(90.7600369111488,20.8254843155585,8.79215601254192));
#29763=CARTESIAN_POINT('Ctrl Pts',(88.6638104940886,23.3035989555453,8.63417284729328));
#29764=CARTESIAN_POINT('Ctrl Pts',(89.5936183463281,26.4133952806053,8.47618968204464));
#29765=CARTESIAN_POINT('Ctrl Pts',(92.7060981989779,27.3341488591493,8.31820651679601));
#29766=CARTESIAN_POINT('Ctrl Pts',(95.1781220495298,25.2307209338419,8.16022335154737));
#29767=CARTESIAN_POINT('Ctrl Pts',(94.7674811338141,22.010984513332,8.00224018629874));
#29768=CARTESIAN_POINT('Ctrl Pts',(91.8466401695451,20.5953543019742,7.84425702105011));
#29769=CARTESIAN_POINT('Ctrl Pts',(89.0649019039696,22.2678533231826,7.68627385580147));
#29770=CARTESIAN_POINT('Ctrl Pts',(88.9453977447207,25.5114688073361,7.52829069055284));
#29771=CARTESIAN_POINT('Ctrl Pts',(91.5965221146138,27.3841303441547,7.3703075253042));
#29772=CARTESIAN_POINT('Ctrl Pts',(94.613614686622,26.1872702243476,7.21232436005557));
#29773=CARTESIAN_POINT('Ctrl Pts',(95.2600695352199,23.0064813190265,7.05434119480693));
#29774=CARTESIAN_POINT('Ctrl Pts',(92.9495300394564,20.7268477858015,6.8963580295583));
#29775=CARTESIAN_POINT('Ctrl Pts',(89.7777343897591,21.4160750219737,6.73837486430966));
#29776=CARTESIAN_POINT('Ctrl Pts',(88.621609498579,24.449010412316,6.58039169906103));
#29777=CARTESIAN_POINT('Ctrl Pts',(90.529800104221,27.0746780309427,6.42240853381239));
#29778=CARTESIAN_POINT('Ctrl Pts',(93.7715121962504,26.9115077311595,6.26442536856376));
#29779=CARTESIAN_POINT('Ctrl Pts',(95.406402260849,24.1075005427208,6.10644220331512));
#29780=CARTESIAN_POINT('Ctrl Pts',(93.9515692070094,21.205986693053,5.94845903806649));
#29781=CARTESIAN_POINT('Ctrl Pts',(90.7265962711881,20.8387382783291,5.79047587281786));
#29782=CARTESIAN_POINT('Ctrl Pts',(88.6566439813937,23.3388621458627,5.63249270756922));
#29783=CARTESIAN_POINT('Ctrl Pts',(89.6192297163781,26.4386606131126,5.47450954232059));
#29784=CARTESIAN_POINT('Ctrl Pts',(92.7412553594183,27.3265106675896,5.31652637707196));
#29785=CARTESIAN_POINT('Ctrl Pts',(95.1909370907925,25.1971020055736,5.15854321182332));
#29786=CARTESIAN_POINT('Ctrl Pts',(94.7463299673765,21.9818809649349,5.00056004657469));
#29787=CARTESIAN_POINT('Ctrl Pts',(91.8107078252533,20.59716277165,4.84257688132604));
#29788=CARTESIAN_POINT('Ctrl Pts',(89.046780146916,22.2989340909708,4.68459371607742));
#29789=CARTESIAN_POINT('Ctrl Pts',(88.9615236743494,25.5436302500664,4.52661055082878));
#29790=CARTESIAN_POINT('Ctrl Pts',(91.6322689402898,27.3882010864546,4.36862738558015));
#29791=CARTESIAN_POINT('Ctrl Pts',(94.6365588259127,26.1595578877736,4.21064422033151));
#29792=CARTESIAN_POINT('Ctrl Pts',(95.249399871001,22.9721219808507,4.05266105508288));
#29793=CARTESIAN_POINT('Ctrl Pts',(92.9149243119076,20.7170065080898,3.89467788983424));
#29794=CARTESIAN_POINT('Ctrl Pts',(89.7505811985077,21.4396782144198,3.73669472458561));
#29795=CARTESIAN_POINT('Ctrl Pts',(88.6265376646408,24.4846491157739,3.57871155933697));
#29796=CARTESIAN_POINT('Ctrl Pts',(90.5623397164288,27.0900268368369,3.42072839408834));
#29797=CARTESIAN_POINT('Ctrl Pts',(93.8021485034431,26.8926445233075,3.2627452288397));
#29798=CARTESIAN_POINT('Ctrl Pts',(95.4073475205004,24.0715353532293,3.10476206359107));
#29799=CARTESIAN_POINT('Ctrl Pts',(93.9219651501729,21.1855402400771,2.94677889834244));
#29800=CARTESIAN_POINT('Ctrl Pts',(90.6932965980705,20.8523581047152,2.7887957330938));
#29801=CARTESIAN_POINT('Ctrl Pts',(88.6498489344685,23.3741906986185,2.63081256784517));
#29802=CARTESIAN_POINT('Ctrl Pts',(89.645110188094,26.4636616666768,2.47282940259653));
#29803=CARTESIAN_POINT('Ctrl Pts',(92.776321450571,27.3184911176409,2.3148462373479));
#29804=CARTESIAN_POINT('Ctrl Pts',(95.2034141737259,25.1633691432978,2.15686307209926));
#29805=CARTESIAN_POINT('Ctrl Pts',(94.7248365303563,21.9529636570868,1.99887990685063));
#29806=CARTESIAN_POINT('Ctrl Pts',(91.7748706375752,20.5994288843227,1.84089674160199));
#29807=CARTESIAN_POINT('Ctrl Pts',(89.0288361767659,22.3300444971853,1.68291357635336));
#29808=CARTESIAN_POINT('Ctrl Pts',(88.9782973432405,25.5759462608191,1.52493041110473));
#29809=CARTESIAN_POINT('Ctrl Pts',(91.6674251334267,27.3912269563367,1.36694724585609));
#29810=CARTESIAN_POINT('Ctrl Pts',(94.660500490787,26.1329806281354,1.20896408060746));
#29811=CARTESIAN_POINT('Ctrl Pts',(95.2356805466308,22.9350445397703,1.05098091535882));
#29812=CARTESIAN_POINT('Ctrl Pts',(93.6691444859934,21.4566360720578,0.945658805193066));
#29813=CARTESIAN_POINT('Ctrl Pts',(92.7459328543469,21.2098224301578,0.892997750110188));
#29814=CARTESIAN_POINT('Ctrl Pts',(94.3360626576961,25.9973015569306,10.3210067496694));
#29815=CARTESIAN_POINT('Ctrl Pts',(94.9969281342143,25.2243470893904,10.2683456945866));
#29816=CARTESIAN_POINT('Ctrl Pts',(95.4795861102126,22.9835135476832,10.1630235844208));
#29817=CARTESIAN_POINT('Ctrl Pts',(93.0474782509995,20.5256860208715,10.0050404191722));
#29818=CARTESIAN_POINT('Ctrl Pts',(89.664139324633,21.2264194015161,9.84705725392353));
#29819=CARTESIAN_POINT('Ctrl Pts',(88.4000490356599,24.4393717208737,9.68907408867489));
#29820=CARTESIAN_POINT('Ctrl Pts',(90.4009679157595,27.2555128800837,9.53109092342627));
#29821=CARTESIAN_POINT('Ctrl Pts',(93.8523952892238,27.1179538105414,9.37310775817762));
#29822=CARTESIAN_POINT('Ctrl Pts',(95.6235723677572,24.1527148994824,9.215124592929));
#29823=CARTESIAN_POINT('Ctrl Pts',(94.1080772256066,21.0487573061686,9.05714142768035));
#29824=CARTESIAN_POINT('Ctrl Pts',(90.6804686178369,20.6217759976464,8.89915826243173));
#29825=CARTESIAN_POINT('Ctrl Pts',(88.4497275850589,23.2589109780836,8.74117509718308));
#29826=CARTESIAN_POINT('Ctrl Pts',(89.4392011036202,26.5682625869723,8.58319193193445));
#29827=CARTESIAN_POINT('Ctrl Pts',(92.7514084417654,27.5481008201034,8.42520876668582));
#29828=CARTESIAN_POINT('Ctrl Pts',(95.382061787488,25.3096961590962,8.26722560143718));
#29829=CARTESIAN_POINT('Ctrl Pts',(94.9450700899456,21.8833496110771,8.10924243618856));
#29830=CARTESIAN_POINT('Ctrl Pts',(91.8367990863051,20.3768785667209,7.95125927093992));
#29831=CARTESIAN_POINT('Ctrl Pts',(88.876556986041,22.1567016638473,7.79327610569128));
#29832=CARTESIAN_POINT('Ctrl Pts',(88.7493842582027,25.6084595923645,7.63529294044265));
#29833=CARTESIAN_POINT('Ctrl Pts',(91.5706309836454,27.601289611435,7.47730977519401));
#29834=CARTESIAN_POINT('Ctrl Pts',(94.781330049974,26.327627111039,7.31932660994538));
#29835=CARTESIAN_POINT('Ctrl Pts',(95.4692678342078,22.9427273359205,7.16134344469674));
#29836=CARTESIAN_POINT('Ctrl Pts',(93.0104612763355,20.5168099727604,7.00336027944811));
#29837=CARTESIAN_POINT('Ctrl Pts',(89.6351318530524,21.2502648439158,6.84537711419948));
#29838=CARTESIAN_POINT('Ctrl Pts',(88.4048185563678,24.4778233604662,6.68739394895084));
#29839=CARTESIAN_POINT('Ctrl Pts',(90.4354575406507,27.2719797777491,6.5294107837022));
#29840=CARTESIAN_POINT('Ctrl Pts',(93.8851899365835,27.0983388580017,6.37142761845357));
#29841=CARTESIAN_POINT('Ctrl Pts',(95.624990714543,24.1143988405745,6.21344445320494));
#29842=CARTESIAN_POINT('Ctrl Pts',(94.0768011856692,21.0266951703267,6.0554612879563));
#29843=CARTESIAN_POINT('Ctrl Pts',(90.6448820957342,20.6358804657318,5.89747812270767));
#29844=CARTESIAN_POINT('Ctrl Pts',(88.4421011980427,23.2964370033963,5.73949495745903));
#29845=CARTESIAN_POINT('Ctrl Pts',(89.4664559524339,26.5951491930526,5.5815117922104));
#29846=CARTESIAN_POINT('Ctrl Pts',(92.7888216332755,27.5399724866421,5.42352862696176));
#29847=CARTESIAN_POINT('Ctrl Pts',(95.3956991685213,25.2739199079453,5.26554546171313));
#29848=CARTESIAN_POINT('Ctrl Pts',(94.9225616555133,21.8523784912208,5.1075622964645));
#29849=CARTESIAN_POINT('Ctrl Pts',(91.798560967482,20.3788030856943,4.94957913121586));
#29850=CARTESIAN_POINT('Ctrl Pts',(88.8572723578556,22.189776881043,4.79159596596723));
#29851=CARTESIAN_POINT('Ctrl Pts',(88.7665449869396,25.642684831293,4.63361280071859));
#29852=CARTESIAN_POINT('Ctrl Pts',(91.608671679144,27.6056215728149,4.47562963546996));
#29853=CARTESIAN_POINT('Ctrl Pts',(94.8057465121273,26.2981364769134,4.31764647022132));
#29854=CARTESIAN_POINT('Ctrl Pts',(95.4579134988245,22.9061631628408,4.15966330497269));
#29855=CARTESIAN_POINT('Ctrl Pts',(92.973634903104,20.506337181354,4.00168013972405));
#29856=CARTESIAN_POINT('Ctrl Pts',(89.6062362445426,21.2753826505923,3.84369697447542));
#29857=CARTESIAN_POINT('Ctrl Pts',(88.4100629622968,24.5157489955558,3.68571380922678));
#29858=CARTESIAN_POINT('Ctrl Pts',(90.47008521615,27.2883135148081,3.52773064397815));
#29859=CARTESIAN_POINT('Ctrl Pts',(93.9177921721967,27.0782652002028,3.36974747872952));
#29860=CARTESIAN_POINT('Ctrl Pts',(95.6259966314009,24.0761257688788,3.21176431348088));
#29861=CARTESIAN_POINT('Ctrl Pts',(94.0452974398027,21.0049366707405,3.05378114823225));
#29862=CARTESIAN_POINT('Ctrl Pts',(90.6094455863014,20.6503742748602,2.89579798298361));
#29863=CARTESIAN_POINT('Ctrl Pts',(88.434870113713,23.3340325854478,2.73781481773498));
#29864=CARTESIAN_POINT('Ctrl Pts',(89.4939971711376,26.6217545614397,2.57983165248634));
#29865=CARTESIAN_POINT('Ctrl Pts',(92.8261379115921,27.5314383230663,2.42184848723771));
#29866=CARTESIAN_POINT('Ctrl Pts',(95.4089769044768,25.2380224116542,2.26386532198907));
#29867=CARTESIAN_POINT('Ctrl Pts',(94.8996889870333,21.8216055629487,2.10588215674044));
#29868=CARTESIAN_POINT('Ctrl Pts',(91.760424111462,20.3812146145649,1.94789899149181));
#29869=CARTESIAN_POINT('Ctrl Pts',(88.8381769251393,22.2228836385593,1.78991582624317));
#29870=CARTESIAN_POINT('Ctrl Pts',(88.7843950202953,25.6770745568565,1.63193266099454));
#29871=CARTESIAN_POINT('Ctrl Pts',(91.6460838412789,27.6088416124303,1.47394949574591));
#29872=CARTESIAN_POINT('Ctrl Pts',(94.8312245109702,26.2698537574842,1.31596633049727));
#29873=CARTESIAN_POINT('Ctrl Pts',(95.4433138069375,22.8667064664957,1.15798316524863));
#29874=CARTESIAN_POINT('Ctrl Pts',(93.7762533017603,21.2934286920664,1.05266105508288));
#29875=CARTESIAN_POINT('Ctrl Pts',(92.7937992825328,21.0307770462543,0.999999999999999));
#29876=CARTESIAN_POINT('Ctrl Pts',(93.9134659966651,25.6359872033749,10.));
#29877=CARTESIAN_POINT('Ctrl Pts',(93.9750770243691,25.5780879660668,10.));
#29878=CARTESIAN_POINT('Ctrl Pts',(94.0333189464364,25.5170381633454,10.));
#29879=CARTESIAN_POINT('Ctrl Pts',(94.088194094267,25.4532225723848,10.));
#29880=CARTESIAN_POINT('Ctrl Pts',(94.1445219524055,25.3877175906808,10.));
#29881=CARTESIAN_POINT('Ctrl Pts',(94.1973028564882,25.3192980131866,10.));
#29882=CARTESIAN_POINT('Ctrl Pts',(94.2465138207336,25.2483314405892,10.));
#29883=CARTESIAN_POINT('Ctrl Pts',(94.2970863146417,25.1754014215296,10.));
#29884=CARTESIAN_POINT('Ctrl Pts',(94.3438891300174,25.0997809660001,10.));
#29885=CARTESIAN_POINT('Ctrl Pts',(94.3868632217433,25.0218260241029,10.));
#29886=CARTESIAN_POINT('Ctrl Pts',(94.4057547014815,24.9875569064508,10.));
#29887=CARTESIAN_POINT('Ctrl Pts',(94.4239057978348,24.9528361527832,10.));
#29888=CARTESIAN_POINT('Ctrl Pts',(94.4413090769948,24.9176919312935,10.));
#29889=CARTESIAN_POINT('Ctrl Pts',(94.4512341001083,24.8976493170607,10.));
#29890=CARTESIAN_POINT('Ctrl Pts',(94.4609158766235,24.8774689544396,10.));
#29891=CARTESIAN_POINT('Ctrl Pts',(94.4703527940363,24.8571559201793,10.));
#29892=CARTESIAN_POINT('Ctrl Pts',(94.4788698089046,24.8388229829234,10.));
#29893=CARTESIAN_POINT('Ctrl Pts',(94.48718975873,24.8203762304135,10.));
#29894=CARTESIAN_POINT('Ctrl Pts',(94.4952977634445,24.8018512256524,10.));
#29895=CARTESIAN_POINT('Ctrl Pts',(94.5318624413391,24.7183089910421,10.));
#29896=CARTESIAN_POINT('Ctrl Pts',(94.5641668037087,24.6330832595078,10.));
#29897=CARTESIAN_POINT('Ctrl Pts',(94.5921857513385,24.5465727477908,10.));
#29898=CARTESIAN_POINT('Ctrl Pts',(94.6206673939169,24.4586336322127,10.));
#29899=CARTESIAN_POINT('Ctrl Pts',(94.6447214108873,24.3693661982349,10.));
#29900=CARTESIAN_POINT('Ctrl Pts',(94.6642823633474,24.279152120929,10.));
#29901=CARTESIAN_POINT('Ctrl Pts',(94.683262749204,24.1916155860673,10.));
#29902=CARTESIAN_POINT('Ctrl Pts',(94.6980129804155,24.1031868495632,10.));
#29903=CARTESIAN_POINT('Ctrl Pts',(94.7084324536937,24.0141926985119,10.));
#29904=CARTESIAN_POINT('Ctrl Pts',(94.7127917941012,23.976958973894,10.));
#29905=CARTESIAN_POINT('Ctrl Pts',(94.7163925414667,23.9396260845753,10.));
#29906=CARTESIAN_POINT('Ctrl Pts',(94.7192250066991,23.9022173486862,10.));
#29907=CARTESIAN_POINT('Ctrl Pts',(94.7209955764803,23.8788332038215,10.));
#29908=CARTESIAN_POINT('Ctrl Pts',(94.7224659134476,23.8554194166543,10.));
#29909=CARTESIAN_POINT('Ctrl Pts',(94.7236333606835,23.8319816504978,10.));
#29910=CARTESIAN_POINT('Ctrl Pts',(94.724317620347,23.818244397549,10.));
#29911=CARTESIAN_POINT('Ctrl Pts',(94.7248975539046,23.8045034755981,10.));
#29912=CARTESIAN_POINT('Ctrl Pts',(94.7253726391635,23.7907682591662,10.));
#29913=CARTESIAN_POINT('Ctrl Pts',(94.7287304225261,23.6936911969805,10.));
#29914=CARTESIAN_POINT('Ctrl Pts',(94.7268610241325,23.596778684182,10.));
#29915=CARTESIAN_POINT('Ctrl Pts',(94.7196996503297,23.5004529825499,10.));
#29916=CARTESIAN_POINT('Ctrl Pts',(94.7125382765269,23.4041272809177,10.));
#29917=CARTESIAN_POINT('Ctrl Pts',(94.7000853621774,23.3083873359331,10.));
#29918=CARTESIAN_POINT('Ctrl Pts',(94.6822232210626,23.2136364705516,10.));
#29919=CARTESIAN_POINT('Ctrl Pts',(94.6651456877563,23.12304760727,10.));
#29920=CARTESIAN_POINT('Ctrl Pts',(94.6431238131852,23.0333618679134,10.));
#29921=CARTESIAN_POINT('Ctrl Pts',(94.6164322917056,22.9448185902262,10.));
#29922=CARTESIAN_POINT('Ctrl Pts',(94.6074974122224,22.9151790840711,10.));
#29923=CARTESIAN_POINT('Ctrl Pts',(94.5980388404184,22.885667632781,10.));
#29924=CARTESIAN_POINT('Ctrl Pts',(94.588065604527,22.8562933928181,10.));
#29925=CARTESIAN_POINT('Ctrl Pts',(94.5815842777681,22.8372038967343,10.));
#29926=CARTESIAN_POINT('Ctrl Pts',(94.5748855784168,22.8181723520541,10.));
#29927=CARTESIAN_POINT('Ctrl Pts',(94.5679718479818,22.7992013069027,10.));
#29928=CARTESIAN_POINT('Ctrl Pts',(94.5613824030787,22.7811200904081,10.));
#29929=CARTESIAN_POINT('Ctrl Pts',(94.5545958744184,22.7630896215814,10.));
#29930=CARTESIAN_POINT('Ctrl Pts',(94.5476250811124,22.7451392560728,10.));
#29931=CARTESIAN_POINT('Ctrl Pts',(94.5137816042513,22.6579895224528,10.));
#29932=CARTESIAN_POINT('Ctrl Pts',(94.4755597867714,22.5726140967881,10.));
#29933=CARTESIAN_POINT('Ctrl Pts',(94.4332908111416,22.4892465922063,10.));
#29934=CARTESIAN_POINT('Ctrl Pts',(94.3894525927547,22.4027840551381,10.));
#29935=CARTESIAN_POINT('Ctrl Pts',(94.3412610125979,22.3184805709375,10.));
#29936=CARTESIAN_POINT('Ctrl Pts',(94.2890295505398,22.2365997560127,10.));
#29937=CARTESIAN_POINT('Ctrl Pts',(94.2362096760877,22.1537965145573,10.));
#29938=CARTESIAN_POINT('Ctrl Pts',(94.1792579755655,22.0734700151482,10.));
#29939=CARTESIAN_POINT('Ctrl Pts',(94.1184468579888,21.9959077298342,10.));
#29940=CARTESIAN_POINT('Ctrl Pts',(94.0767843459049,21.9427687681127,10.));
#29941=CARTESIAN_POINT('Ctrl Pts',(94.0333092171587,21.8909275801965,10.));
#29942=CARTESIAN_POINT('Ctrl Pts',(93.9880968596546,21.8404836536314,10.));
#29943=CARTESIAN_POINT('Ctrl Pts',(93.9759899524546,21.8269758435669,10.));
#29944=CARTESIAN_POINT('Ctrl Pts',(93.9637571446612,21.8135670091799,10.));
#29945=CARTESIAN_POINT('Ctrl Pts',(93.951413501835,21.8002735576985,10.));
#29946=CARTESIAN_POINT('Ctrl Pts',(93.882752721598,21.7263295232182,10.));
#29947=CARTESIAN_POINT('Ctrl Pts',(93.810578049503,21.6558533764537,10.));
#29948=CARTESIAN_POINT('Ctrl Pts',(93.7351999444248,21.5891349259443,10.));
#29949=CARTESIAN_POINT('Ctrl Pts',(93.6722950971385,21.5334567693214,10.));
#29950=CARTESIAN_POINT('Ctrl Pts',(93.6071581999104,21.4803955991654,10.));
#29951=CARTESIAN_POINT('Ctrl Pts',(93.5399460223894,21.4301336195356,10.));
#29952=CARTESIAN_POINT('Ctrl Pts',(93.5180637926007,21.4137698558775,10.));
#29953=CARTESIAN_POINT('Ctrl Pts',(93.4959614384794,21.3977029162792,10.));
#29954=CARTESIAN_POINT('Ctrl Pts',(93.4736439440714,21.3819394740093,10.));
#29955=CARTESIAN_POINT('Ctrl Pts',(93.4508750631855,21.3658572054161,10.));
#29956=CARTESIAN_POINT('Ctrl Pts',(93.4278768370864,21.3500874072995,10.));
#29957=CARTESIAN_POINT('Ctrl Pts',(93.4046836949952,21.3346563933178,10.));
#29958=CARTESIAN_POINT('Ctrl Pts',(93.3197384270806,21.2781400484554,10.));
#29959=CARTESIAN_POINT('Ctrl Pts',(93.2321268832175,21.226124130751,10.));
#29960=CARTESIAN_POINT('Ctrl Pts',(93.1421393261376,21.1789167035699,10.));
#29961=CARTESIAN_POINT('Ctrl Pts',(93.0588657605654,21.1352314329567,10.));
#29962=CARTESIAN_POINT('Ctrl Pts',(92.9735566878419,21.0956636399515,10.));
#29963=CARTESIAN_POINT('Ctrl Pts',(92.8864147107142,21.0604862982088,10.));
#29964=CARTESIAN_POINT('Ctrl Pts',(92.856390770472,21.048366279348,10.));
#29965=CARTESIAN_POINT('Ctrl Pts',(92.8261490486008,21.0367677258533,10.));
#29966=CARTESIAN_POINT('Ctrl Pts',(92.7957019287907,21.0256870573369,10.));
#29967=CARTESIAN_POINT('Ctrl Pts',(89.481789046694,23.9978055657336,8.38741669750803));
#29968=CARTESIAN_POINT('Ctrl Pts',(89.480223059461,23.8252749393967,8.39833391417657));
#29969=CARTESIAN_POINT('Ctrl Pts',(89.4964590311695,23.6530372319079,8.40925113084511));
#29970=CARTESIAN_POINT('Ctrl Pts',(89.5315885963512,23.4847435435215,8.42016834751366));
#29971=CARTESIAN_POINT('Ctrl Pts',(89.7010420406894,22.67295025744,8.47282940259653));
#29972=CARTESIAN_POINT('Ctrl Pts',(90.3101077692311,21.9529256044114,8.52549045767941));
#29973=CARTESIAN_POINT('Ctrl Pts',(91.0825656196773,21.6512032537229,8.57815151276229));
#29974=CARTESIAN_POINT('Ctrl Pts',(91.8550234701235,21.3494809030344,8.63081256784517));
#29975=CARTESIAN_POINT('Ctrl Pts',(92.7908734424743,21.4660608546861,8.68347362292805));
#29976=CARTESIAN_POINT('Ctrl Pts',(93.4656884574097,21.9480921266005,8.73613467801093));
#29977=CARTESIAN_POINT('Ctrl Pts',(94.1405034723451,22.4301233985148,8.78879573309381));
#29978=CARTESIAN_POINT('Ctrl Pts',(94.5542835298652,23.2776059906917,8.84145678817668));
#29979=CARTESIAN_POINT('Ctrl Pts',(94.5193787375631,24.1061511997237,8.89411784325956));
#29980=CARTESIAN_POINT('Ctrl Pts',(94.4844739452609,24.9346964087557,8.94677889834243));
#29981=CARTESIAN_POINT('Ctrl Pts',(94.0008843031365,25.7443042346427,8.99943995342532));
#29982=CARTESIAN_POINT('Ctrl Pts',(93.2879128423749,26.1678872245111,9.0521010085082));
#29983=CARTESIAN_POINT('Ctrl Pts',(92.5749413816133,26.5914702143796,9.10476206359107));
#29984=CARTESIAN_POINT('Ctrl Pts',(91.6325881022146,26.6290283682294,9.15742311867395));
#29985=CARTESIAN_POINT('Ctrl Pts',(90.8882531044733,26.2633578291731,9.21008417375683));
#29986=CARTESIAN_POINT('Ctrl Pts',(90.1439181067321,25.8976872901167,9.2627452288397));
#29987=CARTESIAN_POINT('Ctrl Pts',(89.5976013906482,25.1287880581541,9.31540628392258));
#29988=CARTESIAN_POINT('Ctrl Pts',(89.4970121613135,24.3057175721558,9.36806733900546));
#29989=CARTESIAN_POINT('Ctrl Pts',(89.484692259653,24.2049100849695,9.37451712517298));
#29990=CARTESIAN_POINT('Ctrl Pts',(89.4790585822288,24.1032899910618,9.3809669113405));
#29991=CARTESIAN_POINT('Ctrl Pts',(89.4798237559162,24.0015869167785,9.38741669750802));
#29992=CARTESIAN_POINT('Ctrl Pts',(91.2062007174671,21.0307770462543,10.));
#29993=CARTESIAN_POINT('Ctrl Pts',(90.2237466982397,21.2934286920664,9.94733894491712));
#29994=CARTESIAN_POINT('Ctrl Pts',(88.5566850319539,22.8666986268703,9.84201683475137));
#29995=CARTESIAN_POINT('Ctrl Pts',(89.1687764925373,26.2698561140492,9.68403366950273));
#29996=CARTESIAN_POINT('Ctrl Pts',(92.3539160756187,27.6088391884301,9.5260505042541));
#29997=CARTESIAN_POINT('Ctrl Pts',(95.2156041936735,25.6770751085581,9.36806733900546));
#29998=CARTESIAN_POINT('Ctrl Pts',(95.1618224985938,22.2228835192268,9.21008417375683));
#29999=CARTESIAN_POINT('Ctrl Pts',(92.2395757642924,20.3812156575975,9.05210100850819));
#30000=CARTESIAN_POINT('Ctrl Pts',(89.1003116800245,21.8216058830164,8.89411784325956));
#30001=CARTESIAN_POINT('Ctrl Pts',(88.5910237941293,25.238022224588,8.73613467801092));
#30002=CARTESIAN_POINT('Ctrl Pts',(91.1738622820844,27.531437528054,8.57815151276229));
#30003=CARTESIAN_POINT('Ctrl Pts',(94.5060022838614,26.6217540231211,8.42016834751365));
#30004=CARTESIAN_POINT('Ctrl Pts',(95.5651291305171,23.3340327163824,8.26218518226502));
#30005=CARTESIAN_POINT('Ctrl Pts',(93.3905541137143,20.6503749960184,8.10420201701639));
#30006=CARTESIAN_POINT('Ctrl Pts',(89.9547029986071,21.0049373072501,7.94621885176775));
#30007=CARTESIAN_POINT('Ctrl Pts',(88.3740041419999,24.0761257542051,7.78823568651913));
#30008=CARTESIAN_POINT('Ctrl Pts',(90.0822082378052,27.0782645420543,7.63025252127047));
#30009=CARTESIAN_POINT('Ctrl Pts',(93.5299144568995,27.2883128130434,7.47226935602186));
#30010=CARTESIAN_POINT('Ctrl Pts',(95.5899362712428,24.5157488852068,7.31428619077321));
#30011=CARTESIAN_POINT('Ctrl Pts',(94.3937632442239,21.2753832325168,7.15630302552458));
#30012=CARTESIAN_POINT('Ctrl Pts',(91.0263653048422,20.5063379273329,6.99831986027594));
#30013=CARTESIAN_POINT('Ctrl Pts',(88.542087239558,22.9061633964473,6.84033669502731));
#30014=CARTESIAN_POINT('Ctrl Pts',(89.1942540870206,26.2981359861554,6.68235352977868));
#30015=CARTESIAN_POINT('Ctrl Pts',(92.3913282372869,27.6056208028793,6.52437036453004));
#30016=CARTESIAN_POINT('Ctrl Pts',(95.2334543225921,25.6426844805108,6.36638719928141));
#30017=CARTESIAN_POINT('Ctrl Pts',(95.1427269710462,22.1897772675992,6.20840403403277));
#30018=CARTESIAN_POINT('Ctrl Pts',(92.2014389895034,20.3788038589624,6.05042086878414));
#30019=CARTESIAN_POINT('Ctrl Pts',(89.0774389685691,21.8523789498236,5.89243770353551));
#30020=CARTESIAN_POINT('Ctrl Pts',(88.6043015565952,25.2739196359127,5.73445453828687));
#30021=CARTESIAN_POINT('Ctrl Pts',(91.2111785351691,27.5399717307178,5.57647137303823));
#30022=CARTESIAN_POINT('Ctrl Pts',(94.533543506554,26.5951486388853,5.41848820778961));
#30023=CARTESIAN_POINT('Ctrl Pts',(95.5578980422049,23.2964371536349,5.26050504254096));
#30024=CARTESIAN_POINT('Ctrl Pts',(93.3551176148942,20.6358811841045,5.10252187729233));
#30025=CARTESIAN_POINT('Ctrl Pts',(89.9231992578103,21.0266958052455,4.9445387120437));
#30026=CARTESIAN_POINT('Ctrl Pts',(88.3750100595362,24.1143988161452,4.78655554679507));
#30027=CARTESIAN_POINT('Ctrl Pts',(90.1148104659794,27.0983381963848,4.62857238154643));
#30028=CARTESIAN_POINT('Ctrl Pts',(93.5645421252575,27.2719790790494,4.4705892162978));
#30029=CARTESIAN_POINT('Ctrl Pts',(95.5951806759186,24.4778232584366,4.31260605104916));
#30030=CARTESIAN_POINT('Ctrl Pts',(94.3648676419543,21.2502654310841,4.15462288580052));
#30031=CARTESIAN_POINT('Ctrl Pts',(90.9895389394379,20.5168107165773,3.99663972055189));
#30032=CARTESIAN_POINT('Ctrl Pts',(88.530732906619,22.9427275616555,3.83865655530326));
#30033=CARTESIAN_POINT('Ctrl Pts',(89.2186705439483,26.3276266140658,3.68067339005462));
#30034=CARTESIAN_POINT('Ctrl Pts',(92.4293689246723,27.6012888422859,3.52269022480599));
#30035=CARTESIAN_POINT('Ctrl Pts',(95.2506150476497,25.6084592491483,3.36470705955735));
#30036=CARTESIAN_POINT('Ctrl Pts',(95.1234423470095,22.1567020569745,3.20672389430872));
#30037=CARTESIAN_POINT('Ctrl Pts',(92.1632008787758,20.3768793413443,3.04874072906008));
#30038=CARTESIAN_POINT('Ctrl Pts',(89.0549305391036,21.8833500612562,2.89075756381145));
#30039=CARTESIAN_POINT('Ctrl Pts',(88.617938934352,25.309695882881,2.73277439856282));
#30040=CARTESIAN_POINT('Ctrl Pts',(91.2485917195107,27.5481000558719,2.57479123331418));
#30041=CARTESIAN_POINT('Ctrl Pts',(94.5607983477153,26.5682620509694,2.41680806806555));
#30042=CARTESIAN_POINT('Ctrl Pts',(95.5502716608786,23.2589111130017,2.25882490281691));
#30043=CARTESIAN_POINT('Ctrl Pts',(93.3195310914442,20.621776762524,2.10084173756828));
#30044=CARTESIAN_POINT('Ctrl Pts',(89.8919232441541,21.0487578560498,1.94285857231964));
#30045=CARTESIAN_POINT('Ctrl Pts',(88.3764283632659,24.1527150135632,1.78487540707101));
#30046=CARTESIAN_POINT('Ctrl Pts',(90.1476051992024,27.1179528805983,1.62689224182238));
#30047=CARTESIAN_POINT('Ctrl Pts',(93.5990315417431,27.2555126520044,1.46890907657374));
#30048=CARTESIAN_POINT('Ctrl Pts',(95.5999506290772,24.4393708209746,1.3109259113251));
#30049=CARTESIAN_POINT('Ctrl Pts',(94.3358592338276,21.2264213520667,1.15294274607647));
#30050=CARTESIAN_POINT('Ctrl Pts',(90.9525239108494,20.5256846472501,0.994959580827838));
#30051=CARTESIAN_POINT('Ctrl Pts',(88.5204084922262,22.9835193506337,0.836976415579203));
#30052=CARTESIAN_POINT('Ctrl Pts',(89.0030718657857,25.2243470893904,0.731654305413447));
#30053=CARTESIAN_POINT('Ctrl Pts',(89.6639373423039,25.9973015569306,0.678993250330568));
#30054=CARTESIAN_POINT('Ctrl Pts',(91.254067145653,21.2098224301579,10.1070022498898));
#30055=CARTESIAN_POINT('Ctrl Pts',(90.3308555140066,21.4566360720578,10.0543411948069));
#30056=CARTESIAN_POINT('Ctrl Pts',(88.7643183622759,22.9350371728776,9.94901908464117));
#30057=CARTESIAN_POINT('Ctrl Pts',(89.3395004522086,26.1329828425985,9.79103591939254));
#30058=CARTESIAN_POINT('Ctrl Pts',(92.3325747884819,27.3912246785047,9.6330527541439));
#30059=CARTESIAN_POINT('Ctrl Pts',(95.0217019181265,25.575946779253,9.47506958889527));
#30060=CARTESIAN_POINT('Ctrl Pts',(94.9711632817164,22.3300443850486,9.31708642364663));
#30061=CARTESIAN_POINT('Ctrl Pts',(92.2251292456713,20.59942986446,9.15910325839801));
#30062=CARTESIAN_POINT('Ctrl Pts',(89.2751640964777,21.9529639578543,9.00112009314937));
#30063=CARTESIAN_POINT('Ctrl Pts',(88.7965864827541,25.1633689675118,8.84313692790073));
#30064=CARTESIAN_POINT('Ctrl Pts',(91.2236787314268,27.3184903705682,8.6851537626521));
#30065=CARTESIAN_POINT('Ctrl Pts',(94.3548892997688,26.4636611608191,8.52717059740346));
#30066=CARTESIAN_POINT('Ctrl Pts',(95.3501503553349,23.3741908216578,8.36918743215484));
#30067=CARTESIAN_POINT('Ctrl Pts',(93.3067031200343,20.8523587823872,8.21120426690619));
#30068=CARTESIAN_POINT('Ctrl Pts',(90.0780352618006,21.1855408382049,8.05322110165756));
#30069=CARTESIAN_POINT('Ctrl Pts',(88.5926532062641,24.0715353394404,7.89523793640892));
#30070=CARTESIAN_POINT('Ctrl Pts',(90.1978518818355,26.8926439048457,7.73725477116029));
#30071=CARTESIAN_POINT('Ctrl Pts',(93.4376599763359,27.0900261773889,7.57927160591167));
#30072=CARTESIAN_POINT('Ctrl Pts',(95.3734616151168,24.484649012079,7.42128844066302));
#30073=CARTESIAN_POINT('Ctrl Pts',(94.2494183210864,21.439678761254,7.26330527541439));
#30074=CARTESIAN_POINT('Ctrl Pts',(91.0850758834994,20.7170072090858,7.10532211016575));
#30075=CARTESIAN_POINT('Ctrl Pts',(88.7506008228567,22.9721222003706,6.94733894491712));
#30076=CARTESIAN_POINT('Ctrl Pts',(89.3634417371065,26.1595574266085,6.78935577966849));
#30077=CARTESIAN_POINT('Ctrl Pts',(92.3677309811802,27.3882003629464,6.63137261441985));
#30078=CARTESIAN_POINT('Ctrl Pts',(95.038475676818,25.5436299204366,6.47338944917122));
#30079=CARTESIAN_POINT('Ctrl Pts',(94.9532192224532,22.2989344542176,6.31540628392258));
#30080=CARTESIAN_POINT('Ctrl Pts',(92.1892921343259,20.5971634982897,6.15742311867395));
#30081=CARTESIAN_POINT('Ctrl Pts',(89.2536706190735,21.9818813958838,5.99943995342532));
#30082=CARTESIAN_POINT('Ctrl Pts',(88.8090635905991,25.1971017499447,5.84145678817668));
#30083=CARTESIAN_POINT('Ctrl Pts',(91.258744798869,27.3265099572479,5.68347362292805));
#30084=CARTESIAN_POINT('Ctrl Pts',(94.3807697752332,26.4386600923617,5.52549045767941));
#30085=CARTESIAN_POINT('Ctrl Pts',(95.3433553046672,23.3388622870419,5.36750729243078));
#30086=CARTESIAN_POINT('Ctrl Pts',(93.2734034568898,20.8387389533836,5.20952412718214));
#30087=CARTESIAN_POINT('Ctrl Pts',(90.048431209728,21.2059872896859,5.05154096193352));
#30088=CARTESIAN_POINT('Ctrl Pts',(88.5935984665529,24.1075005197647,4.89355779668487));
#30089=CARTESIAN_POINT('Ctrl Pts',(90.2284881820376,26.9115071094383,4.73557463143624));
#30090=CARTESIAN_POINT('Ctrl Pts',(93.4701995818332,27.0746773743749,4.5775914661876));
#30091=CARTESIAN_POINT('Ctrl Pts',(95.3783897800006,24.4490103164388,4.41960830093897));
#30092=CARTESIAN_POINT('Ctrl Pts',(94.2222651356991,21.4160755737355,4.26162513569033));
#30093=CARTESIAN_POINT('Ctrl Pts',(91.0504701633057,20.7268484847659,4.10364197044171));
#30094=CARTESIAN_POINT('Ctrl Pts',(88.7399311609349,23.0064815311496,3.94565880519306));
#30095=CARTESIAN_POINT('Ctrl Pts',(89.3863858714864,26.1872697573421,3.78767563994444));
#30096=CARTESIAN_POINT('Ctrl Pts',(92.4034777992323,27.3841296213857,3.6296924746958));
#30097=CARTESIAN_POINT('Ctrl Pts',(95.0546016029891,25.5114684848159,3.47170930944717));
#30098=CARTESIAN_POINT('Ctrl Pts',(94.9350974692982,22.2678536926041,3.31372614419853));
#30099=CARTESIAN_POINT('Ctrl Pts',(92.1533597976414,20.5953550298875,3.1557429789499));
#30100=CARTESIAN_POINT('Ctrl Pts',(89.2325194573032,22.0109849363651,2.99775981370126));
#30101=CARTESIAN_POINT('Ctrl Pts',(88.8218786287828,25.2307206742826,2.83977664845263));
#30102=CARTESIAN_POINT('Ctrl Pts',(91.2939019525732,27.3341481410013,2.68179348320399));
#30103=CARTESIAN_POINT('Ctrl Pts',(94.4063811380922,26.4133947769236,2.52381031795536));
#30104=CARTESIAN_POINT('Ctrl Pts',(95.3361887973194,23.3035990823278,2.36582715270672));
#30105=CARTESIAN_POINT('Ctrl Pts',(93.2399628156628,20.8254850343137,2.20784398745809));
#30106=CARTESIAN_POINT('Ctrl Pts',(90.0190411527545,21.2267189896148,2.04986082220946));
#30107=CARTESIAN_POINT('Ctrl Pts',(88.5949312459757,24.1435062344795,1.89187765696082));
#30108=CARTESIAN_POINT('Ctrl Pts',(90.2593053791538,26.9299390200037,1.73389449171219));
#30109=CARTESIAN_POINT('Ctrl Pts',(93.5026092721039,27.0592038797562,1.57591132646355));
#30110=CARTESIAN_POINT('Ctrl Pts',(95.382872102992,24.4128765770115,1.41792816121492));
#30111=CARTESIAN_POINT('Ctrl Pts',(94.1950059466948,21.3936693026389,1.25994499596628));
#30112=CARTESIAN_POINT('Ctrl Pts',(91.0156871563966,20.7351873137138,1.10196183071765));
#30113=CARTESIAN_POINT('Ctrl Pts',(88.7302293130409,23.0448135582198,0.943978665469014));
#30114=CARTESIAN_POINT('Ctrl Pts',(89.1837878836397,25.1505184486767,0.838656555303258));
#30115=CARTESIAN_POINT('Ctrl Pts',(89.8048028959809,25.8768634390787,0.785995500220379));
#30116=CARTESIAN_POINT('Ctrl Pts',(91.301933573839,21.3888678140614,10.2140044997796));
#30117=CARTESIAN_POINT('Ctrl Pts',(90.4379643297735,21.6198434520493,10.1613434446967));
#30118=CARTESIAN_POINT('Ctrl Pts',(88.9719516925979,23.0033757188848,10.056021334531));
#30119=CARTESIAN_POINT('Ctrl Pts',(89.5102244118798,25.9961095711478,9.89803816928235));
#30120=CARTESIAN_POINT('Ctrl Pts',(92.3112335013454,27.1736101685792,9.74005500403371));
#30121=CARTESIAN_POINT('Ctrl Pts',(94.8277996425791,25.4748184499478,9.58207183878508));
#30122=CARTESIAN_POINT('Ctrl Pts',(94.7805040648391,22.4372052508704,9.42408867353645));
#30123=CARTESIAN_POINT('Ctrl Pts',(92.2106827270499,20.8176440713226,9.26610550828781));
#30124=CARTESIAN_POINT('Ctrl Pts',(89.4500165129309,22.0843220326922,9.10812234303918));
#30125=CARTESIAN_POINT('Ctrl Pts',(89.0021491713788,25.0887157104356,8.95013917779055));
#30126=CARTESIAN_POINT('Ctrl Pts',(91.273495180769,27.1055432130824,8.79215601254192));
#30127=CARTESIAN_POINT('Ctrl Pts',(94.2037763156761,26.3055682985171,8.63417284729327));
#30128=CARTESIAN_POINT('Ctrl Pts',(95.1351715801526,23.4143489269332,8.47618968204465));
#30129=CARTESIAN_POINT('Ctrl Pts',(93.2228521263546,21.0543425687561,8.31820651679601));
#30130=CARTESIAN_POINT('Ctrl Pts',(90.2013675249939,21.3661443691598,8.16022335154737));
#30131=CARTESIAN_POINT('Ctrl Pts',(88.8113022705282,24.0669449246757,8.00224018629874));
#30132=CARTESIAN_POINT('Ctrl Pts',(90.3134955258656,26.707023267637,7.84425702105011));
#30133=CARTESIAN_POINT('Ctrl Pts',(93.3454054957724,26.8917395417344,7.68627385580147));
#30134=CARTESIAN_POINT('Ctrl Pts',(95.1569869589906,24.4535491389512,7.52829069055285));
#30135=CARTESIAN_POINT('Ctrl Pts',(94.105073397949,21.6039742899911,7.37030752530419));
#30136=CARTESIAN_POINT('Ctrl Pts',(91.1437864621564,20.9276764908387,7.21232436005558));
#30137=CARTESIAN_POINT('Ctrl Pts',(88.9591144061554,23.038081004294,7.05434119480692));
#30138=CARTESIAN_POINT('Ctrl Pts',(89.5326293871924,26.0209788670616,6.89635802955831));
#30139=CARTESIAN_POINT('Ctrl Pts',(92.3441337250735,27.1707799230136,6.73837486430966));
#30140=CARTESIAN_POINT('Ctrl Pts',(94.8434970310438,25.4445753603624,6.58039169906103));
#30141=CARTESIAN_POINT('Ctrl Pts',(94.7637114738601,22.408091640836,6.4224085338124));
#30142=CARTESIAN_POINT('Ctrl Pts',(92.1771452791484,20.8155231376169,6.26442536856376));
#30143=CARTESIAN_POINT('Ctrl Pts',(89.4299022695779,22.111383841944,6.10644220331513));
#30144=CARTESIAN_POINT('Ctrl Pts',(89.013825624603,25.1202838639768,5.94845903806649));
#30145=CARTESIAN_POINT('Ctrl Pts',(91.3063110625691,27.113048183778,5.79047587281786));
#30146=CARTESIAN_POINT('Ctrl Pts',(94.2279960439123,26.2821715458382,5.63249270756923));
#30147=CARTESIAN_POINT('Ctrl Pts',(95.1288125671295,23.3812874204489,5.47450954232059));
#30148=CARTESIAN_POINT('Ctrl Pts',(93.1916892988852,21.0415967226627,5.31652637707195));
#30149=CARTESIAN_POINT('Ctrl Pts',(90.1736631616457,21.3852787741264,5.15854321182332));
#30150=CARTESIAN_POINT('Ctrl Pts',(88.8121868735697,24.1006022233841,5.00056004657469));
#30151=CARTESIAN_POINT('Ctrl Pts',(90.3421658980959,26.7246760224918,4.84257688132605));
#30152=CARTESIAN_POINT('Ctrl Pts',(93.375857038409,26.8773756697003,4.68459371607742));
#30153=CARTESIAN_POINT('Ctrl Pts',(95.1615988840827,24.420197374441,4.52661055082878));
#30154=CARTESIAN_POINT('Ctrl Pts',(94.0796626294438,21.5818857163869,4.36862738558015));
#30155=CARTESIAN_POINT('Ctrl Pts',(91.1114013871734,20.9368862529545,4.21064422033151));
#30156=CARTESIAN_POINT('Ctrl Pts',(88.9491294152508,23.0702355006436,4.05266105508288));
#30157=CARTESIAN_POINT('Ctrl Pts',(89.5541011990245,26.0469129006185,3.89467788983424));
#30158=CARTESIAN_POINT('Ctrl Pts',(92.3775866737925,27.1669704004854,3.73669472458561));
#30159=CARTESIAN_POINT('Ctrl Pts',(94.8585881583285,25.4144777204836,3.57871155933698));
#30160=CARTESIAN_POINT('Ctrl Pts',(94.746752591587,22.3790053282336,3.42072839408834));
#30161=CARTESIAN_POINT('Ctrl Pts',(92.1435187165069,20.8138307184307,3.26274522883971));
#30162=CARTESIAN_POINT('Ctrl Pts',(89.4101083755027,22.138619811474,3.10476206359107));
#30163=CARTESIAN_POINT('Ctrl Pts',(89.0258183232137,25.1517454656841,2.94677889834244));
#30164=CARTESIAN_POINT('Ctrl Pts',(91.3392121856356,27.1201962261306,2.7887957330938));
#30165=CARTESIAN_POINT('Ctrl Pts',(94.2519639284692,26.2585275028778,2.63081256784517));
#30166=CARTESIAN_POINT('Ctrl Pts',(95.12210593376,23.3482870516539,2.47282940259653));
#30167=CARTESIAN_POINT('Ctrl Pts',(93.1603945398814,21.0291933061033,2.3148462373479));
#30168=CARTESIAN_POINT('Ctrl Pts',(90.146159061355,21.4046801231798,2.15686307209927));
#30169=CARTESIAN_POINT('Ctrl Pts',(88.8134341286852,24.1342974553958,1.99887990685063));
#30170=CARTESIAN_POINT('Ctrl Pts',(90.3710055591055,26.7419251594091,1.840896741602));
#30171=CARTESIAN_POINT('Ctrl Pts',(93.4061870024645,26.862895107508,1.68291357635336));
#30172=CARTESIAN_POINT('Ctrl Pts',(95.1657935769071,24.3863823330484,1.52493041110473));
#30173=CARTESIAN_POINT('Ctrl Pts',(94.054152659562,21.560917253211,1.36694724585609));
#30174=CARTESIAN_POINT('Ctrl Pts',(91.0788504019437,20.9446899801776,1.20896408060746));
#30175=CARTESIAN_POINT('Ctrl Pts',(88.9400501338556,23.1061077658059,1.05098091535882));
#30176=CARTESIAN_POINT('Ctrl Pts',(89.3645039014938,25.0766898079629,0.945658805193069));
#30177=CARTESIAN_POINT('Ctrl Pts',(89.9456684496579,25.7564253212268,0.89299775011019));
#30178=CARTESIAN_POINT('Ctrl Pts',(91.3498000020249,21.5679131979649,10.3210067496694));
#30179=CARTESIAN_POINT('Ctrl Pts',(90.5450731455404,21.7830508320407,10.2683456945866));
#30180=CARTESIAN_POINT('Ctrl Pts',(89.1795850229198,23.0717142648921,10.1630235844208));
#30181=CARTESIAN_POINT('Ctrl Pts',(89.6809483715512,25.8592362996971,10.0050404191722));
#30182=CARTESIAN_POINT('Ctrl Pts',(92.2898922142085,26.9559956586539,9.84705725392353));
#30183=CARTESIAN_POINT('Ctrl Pts',(94.6338973670321,25.3736901206426,9.68907408867489));
#30184=CARTESIAN_POINT('Ctrl Pts',(94.5898448479616,22.5443661166922,9.53109092342627));
#30185=CARTESIAN_POINT('Ctrl Pts',(92.1962362084289,21.035858278185,9.37310775817761));
#30186=CARTESIAN_POINT('Ctrl Pts',(89.624868929384,22.2156801075302,9.21512459292901));
#30187=CARTESIAN_POINT('Ctrl Pts',(89.2077118600035,25.0140624533594,9.05714142768035));
#30188=CARTESIAN_POINT('Ctrl Pts',(91.3233116301113,26.8925960555965,8.89915826243173));
#30189=CARTESIAN_POINT('Ctrl Pts',(94.0526633315834,26.1474754362151,8.74117509718308));
#30190=CARTESIAN_POINT('Ctrl Pts',(94.9201928049705,23.4545070322085,8.58319193193445));
#30191=CARTESIAN_POINT('Ctrl Pts',(93.1390011326746,21.2563263551249,8.42520876668582));
#30192=CARTESIAN_POINT('Ctrl Pts',(90.3246997881873,21.5467479001146,8.26722560143718));
#30193=CARTESIAN_POINT('Ctrl Pts',(89.0299513347925,24.0623545099109,8.10924243618856));
#30194=CARTESIAN_POINT('Ctrl Pts',(90.4291391698957,26.5214026304284,7.9512592709399));
#30195=CARTESIAN_POINT('Ctrl Pts',(93.2531510152089,26.6934529060799,7.79327610569129));
#30196=CARTESIAN_POINT('Ctrl Pts',(94.9405123028644,24.4224492658234,7.63529294044264));
#30197=CARTESIAN_POINT('Ctrl Pts',(93.9607284748116,21.7682698187282,7.47730977519402));
#30198=CARTESIAN_POINT('Ctrl Pts',(91.2024970408135,21.1383457725917,7.31932660994538));
#30199=CARTESIAN_POINT('Ctrl Pts',(89.1676279894541,23.1040398082173,7.16134344469674));
#30200=CARTESIAN_POINT('Ctrl Pts',(89.7018170372782,25.8824003075147,7.00336027944811));
#30201=CARTESIAN_POINT('Ctrl Pts',(92.3205364689669,26.9533594830807,6.84537711419947));
#30202=CARTESIAN_POINT('Ctrl Pts',(94.6485183852694,25.3455208002882,6.68739394895084));
#30203=CARTESIAN_POINT('Ctrl Pts',(94.5742037252673,22.5172488274544,6.5294107837022));
#30204=CARTESIAN_POINT('Ctrl Pts',(92.1649984239708,21.0338827769442,6.37142761845357));
#30205=CARTESIAN_POINT('Ctrl Pts',(89.6061339200824,22.2408862880042,6.21344445320493));
#30206=CARTESIAN_POINT('Ctrl Pts',(89.2185876586068,25.0434659780088,6.05546128795631));
#30207=CARTESIAN_POINT('Ctrl Pts',(91.3538773262692,26.8995864103081,5.89747812270766));
#30208=CARTESIAN_POINT('Ctrl Pts',(94.0752223125914,26.1256829993147,5.73949495745904));
#30209=CARTESIAN_POINT('Ctrl Pts',(94.914269829592,23.4237125538558,5.5815117922104));
#30210=CARTESIAN_POINT('Ctrl Pts',(93.1099751408806,21.2444544919418,5.42352862696176));
#30211=CARTESIAN_POINT('Ctrl Pts',(90.2988951135634,21.5645702585669,5.26554546171313));
#30212=CARTESIAN_POINT('Ctrl Pts',(89.0307752805864,24.0937039270036,5.10756229646449));
#30213=CARTESIAN_POINT('Ctrl Pts',(90.4558436141542,26.5378449355454,4.94957913121586));
#30214=CARTESIAN_POINT('Ctrl Pts',(93.2815144949848,26.6800739650258,4.79159596596723));
#30215=CARTESIAN_POINT('Ctrl Pts',(94.9448079881648,24.3913844324432,4.63361280071859));
#30216=CARTESIAN_POINT('Ctrl Pts',(93.9370601231887,21.7476958590383,4.47562963546996));
#30217=CARTESIAN_POINT('Ctrl Pts',(91.1723326110411,21.1469240211431,4.31764647022133));
#30218=CARTESIAN_POINT('Ctrl Pts',(89.1583276695668,23.1339894701376,4.15966330497269));
#30219=CARTESIAN_POINT('Ctrl Pts',(89.7218165265625,25.9065560438948,4.00168013972405));
#30220=CARTESIAN_POINT('Ctrl Pts',(92.3516955483528,26.9498111795851,3.84369697447543));
#30221=CARTESIAN_POINT('Ctrl Pts',(94.6625747136678,25.3174869561513,3.68571380922678));
#30222=CARTESIAN_POINT('Ctrl Pts',(94.5584077138757,22.4901569638631,3.52773064397815));
#30223=CARTESIAN_POINT('Ctrl Pts',(92.1336776353725,21.0323064069739,3.36974747872952));
#30224=CARTESIAN_POINT('Ctrl Pts',(89.5876972937022,22.2662546865829,3.21176431348088));
#30225=CARTESIAN_POINT('Ctrl Pts',(89.2297580176446,25.0727702570857,3.05378114823225));
#30226=CARTESIAN_POINT('Ctrl Pts',(91.3845224186981,26.90624431126,2.89579798298361));
#30227=CARTESIAN_POINT('Ctrl Pts',(94.097546718846,26.103660228832,2.73781481773498));
#30228=CARTESIAN_POINT('Ctrl Pts',(94.9080230702007,23.39297502098,2.57983165248635));
#30229=CARTESIAN_POINT('Ctrl Pts',(93.0808262640999,21.232901577893,2.42184848723771));
#30230=CARTESIAN_POINT('Ctrl Pts',(90.2732769699554,21.5826412567448,2.26386532198908));
#30231=CARTESIAN_POINT('Ctrl Pts',(89.0319370113948,24.1250886763121,2.10588215674044));
#30232=CARTESIAN_POINT('Ctrl Pts',(90.4827057390571,26.5539112988144,1.94789899149181));
#30233=CARTESIAN_POINT('Ctrl Pts',(93.3097647328252,26.6665863352599,1.78991582624318));
#30234=CARTESIAN_POINT('Ctrl Pts',(94.9487150508221,24.3598880890852,1.63193266099454));
#30235=CARTESIAN_POINT('Ctrl Pts',(93.9132993724291,21.7281652037832,1.47394949574591));
#30236=CARTESIAN_POINT('Ctrl Pts',(91.1420136474909,21.1541926466413,1.31596633049727));
#30237=CARTESIAN_POINT('Ctrl Pts',(89.1498709546703,23.167401973392,1.15798316524864));
#30238=CARTESIAN_POINT('Ctrl Pts',(89.5452199193478,25.0028611672492,1.05266105508288));
#30239=CARTESIAN_POINT('Ctrl Pts',(90.0865340033349,25.6359872033749,1.));
#30240=CARTESIAN_POINT('Ctrl Pts',(89.4850510509789,24.0017493960693,9.11258330249199));
#30241=CARTESIAN_POINT('Ctrl Pts',(89.4831440162074,24.294775221213,9.09410267755477));
#30242=CARTESIAN_POINT('Ctrl Pts',(89.5304974072669,24.5872051529597,9.07562205261756));
#30243=CARTESIAN_POINT('Ctrl Pts',(89.6298379999183,24.8607543294274,9.05714142768035));
#30244=CARTESIAN_POINT('Ctrl Pts',(89.9129117833728,25.6402403207718,9.00448037259747));
#30245=CARTESIAN_POINT('Ctrl Pts',(90.6181117067421,26.2664181881842,8.9518193175146));
#30246=CARTESIAN_POINT('Ctrl Pts',(91.425603618672,26.4553203519934,8.89915826243172));
#30247=CARTESIAN_POINT('Ctrl Pts',(92.233095530602,26.6442225158027,8.84649720734885));
#30248=CARTESIAN_POINT('Ctrl Pts',(93.1428794310927,26.3958489760089,8.79383615226596));
#30249=CARTESIAN_POINT('Ctrl Pts',(93.7423596269025,25.8228341387776,8.74117509718308));
#30250=CARTESIAN_POINT('Ctrl Pts',(94.3418398227124,25.2498193015463,8.6885140421002));
#30251=CARTESIAN_POINT('Ctrl Pts',(94.6310163138415,24.3521631668774,8.63585298701733));
#30252=CARTESIAN_POINT('Ctrl Pts',(94.47873928069,23.5369716533623,8.58319193193445));
#30253=CARTESIAN_POINT('Ctrl Pts',(94.3264622475385,22.7217801398473,8.53053087685158));
#30254=CARTESIAN_POINT('Ctrl Pts',(93.7327316901066,21.9890532474861,8.4778698217687));
#30255=CARTESIAN_POINT('Ctrl Pts',(92.9668161873094,21.6710933921371,8.42520876668582));
#30256=CARTESIAN_POINT('Ctrl Pts',(92.2009006845122,21.3531335367881,8.37254771160294));
#30257=CARTESIAN_POINT('Ctrl Pts',(91.2628002363497,21.4499407184514,8.31988665652006));
#30258=CARTESIAN_POINT('Ctrl Pts',(90.5779586033694,21.9176120775824,8.26722560143718));
#30259=CARTESIAN_POINT('Ctrl Pts',(89.9075993003969,22.3753936014113,8.21567816845545));
#30260=CARTESIAN_POINT('Ctrl Pts',(89.4799007520942,23.1885198389857,8.16413073547372));
#30261=CARTESIAN_POINT('Ctrl Pts',(89.4784369335473,24.0003195913806,8.11258330249199));
#30262=CARTESIAN_POINT('Ctrl Pts',(91.2062007174671,21.0307770462543,10.));
#30263=CARTESIAN_POINT('Ctrl Pts',(91.1131475235304,21.0648163202623,10.));
#30264=CARTESIAN_POINT('Ctrl Pts',(91.0221596064764,21.1036239095812,10.));
#30265=CARTESIAN_POINT('Ctrl Pts',(90.9334454653294,21.1468715855109,10.));
#30266=CARTESIAN_POINT('Ctrl Pts',(90.8427656611035,21.1910775118246,10.));
#30267=CARTESIAN_POINT('Ctrl Pts',(90.7544608424801,21.2399230814569,10.));
#30268=CARTESIAN_POINT('Ctrl Pts',(90.6687825963679,21.2931033001222,10.));
#30269=CARTESIAN_POINT('Ctrl Pts',(90.5863301108167,21.3442812993236,10.));
#30270=CARTESIAN_POINT('Ctrl Pts',(90.5063098561185,21.399474570675,10.));
#30271=CARTESIAN_POINT('Ctrl Pts',(90.4289790559023,21.4584413586066,10.));
#30272=CARTESIAN_POINT('Ctrl Pts',(90.3613146057131,21.5100372980466,10.));
#30273=CARTESIAN_POINT('Ctrl Pts',(90.295709559598,21.5645230341409,10.));
#30274=CARTESIAN_POINT('Ctrl Pts',(90.2323608843392,21.6217493205763,10.));
#30275=CARTESIAN_POINT('Ctrl Pts',(90.2182621164007,21.6344855006012,10.));
#30276=CARTESIAN_POINT('Ctrl Pts',(90.2042725067479,21.6473601252806,10.));
#30277=CARTESIAN_POINT('Ctrl Pts',(90.1904136996612,21.6603531214757,10.));
#30278=CARTESIAN_POINT('Ctrl Pts',(90.1179829795585,21.7282588268378,10.));
#30279=CARTESIAN_POINT('Ctrl Pts',(90.0490179328352,21.7994862853565,10.));
#30280=CARTESIAN_POINT('Ctrl Pts',(89.9837585062133,21.8737448951322,10.));
#30281=CARTESIAN_POINT('Ctrl Pts',(89.9188587596277,21.9475942255005,10.));
#30282=CARTESIAN_POINT('Ctrl Pts',(89.8576234119932,22.0244421833297,10.));
#30283=CARTESIAN_POINT('Ctrl Pts',(89.8003320729523,22.1040297129063,10.));
#30284=CARTESIAN_POINT('Ctrl Pts',(89.7451392508881,22.1807020412544,10.));
#30285=CARTESIAN_POINT('Ctrl Pts',(89.6936066323768,22.25991765928,10.));
#30286=CARTESIAN_POINT('Ctrl Pts',(89.6460291433843,22.3414585598246,10.));
#30287=CARTESIAN_POINT('Ctrl Pts',(89.6260403806384,22.37571639372,10.));
#30288=CARTESIAN_POINT('Ctrl Pts',(89.6067503090227,22.4103847699375,10.));
#30289=CARTESIAN_POINT('Ctrl Pts',(89.5881834031273,22.4454478212108,10.));
#30290=CARTESIAN_POINT('Ctrl Pts',(89.575146838384,22.4700669871933,10.));
#30291=CARTESIAN_POINT('Ctrl Pts',(89.5624668273212,22.4948807309457,10.));
#30292=CARTESIAN_POINT('Ctrl Pts',(89.55015232839,22.5198835658164,10.));
#30293=CARTESIAN_POINT('Ctrl Pts',(89.54239983886,22.5356238908298,10.));
#30294=CARTESIAN_POINT('Ctrl Pts',(89.5347913334004,22.5514412806442,10.));
#30295=CARTESIAN_POINT('Ctrl Pts',(89.5273387128366,22.5673132395119,10.));
#30296=CARTESIAN_POINT('Ctrl Pts',(89.4852181501773,22.6570180396273,10.));
#30297=CARTESIAN_POINT('Ctrl Pts',(89.4479997999157,22.7486075345407,10.));
#30298=CARTESIAN_POINT('Ctrl Pts',(89.4159753088237,22.8418092601417,10.));
#30299=CARTESIAN_POINT('Ctrl Pts',(89.3861128448231,22.9287187809694,10.));
#30300=CARTESIAN_POINT('Ctrl Pts',(89.3607667972627,23.0170309840461,10.));
#30301=CARTESIAN_POINT('Ctrl Pts',(89.340224189406,23.1065336320398,10.));
#30302=CARTESIAN_POINT('Ctrl Pts',(89.3387369151237,23.1130135778911,10.));
#30303=CARTESIAN_POINT('Ctrl Pts',(89.3372748417248,23.119499764847,10.));
#30304=CARTESIAN_POINT('Ctrl Pts',(89.3358380889382,23.125992112682,10.));
#30305=CARTESIAN_POINT('Ctrl Pts',(89.3152524900327,23.2190135912048,10.));
#30306=CARTESIAN_POINT('Ctrl Pts',(89.2998606756261,23.3133008086003,10.));
#30307=CARTESIAN_POINT('Ctrl Pts',(89.2895856382548,23.4084457389669,10.));
#30308=CARTESIAN_POINT('Ctrl Pts',(89.2837680062693,23.4623159265052,10.));
#30309=CARTESIAN_POINT('Ctrl Pts',(89.2795916051027,23.5164608839161,10.));
#30310=CARTESIAN_POINT('Ctrl Pts',(89.2770493497674,23.5708038567141,10.));
#30311=CARTESIAN_POINT('Ctrl Pts',(89.2764020101009,23.5846413188308,10.));
#30312=CARTESIAN_POINT('Ctrl Pts',(89.275860775699,23.5984902138897,10.));
#30313=CARTESIAN_POINT('Ctrl Pts',(89.275425710371,23.6123370392804,10.));
#30314=CARTESIAN_POINT('Ctrl Pts',(89.2724969038993,23.7055521709181,10.));
#30315=CARTESIAN_POINT('Ctrl Pts',(89.274367487553,23.7988245804704,10.));
#30316=CARTESIAN_POINT('Ctrl Pts',(89.2809025930419,23.891778995953,10.));
#30317=CARTESIAN_POINT('Ctrl Pts',(89.2874481362156,23.9848818755864,10.));
#30318=CARTESIAN_POINT('Ctrl Pts',(89.2986734920106,24.0776667241966,10.));
#30319=CARTESIAN_POINT('Ctrl Pts',(89.3144940517011,24.1697443147494,10.));
#30320=CARTESIAN_POINT('Ctrl Pts',(89.3300874445373,24.2604997664527,10.));
#30321=CARTESIAN_POINT('Ctrl Pts',(89.3501454854825,24.3505689688124,10.));
#30322=CARTESIAN_POINT('Ctrl Pts',(89.3746301441576,24.4395539724182,10.));
#30323=CARTESIAN_POINT('Ctrl Pts',(89.3838722153721,24.4731425860586,10.));
#30324=CARTESIAN_POINT('Ctrl Pts',(89.3937453934005,24.5065763998858,10.));
#30325=CARTESIAN_POINT('Ctrl Pts',(89.4042490565665,24.5398326838582,10.));
#30326=CARTESIAN_POINT('Ctrl Pts',(89.4119449769147,24.5641992032794,10.));
#30327=CARTESIAN_POINT('Ctrl Pts',(89.4199793786913,24.5884704030463,10.));
#30328=CARTESIAN_POINT('Ctrl Pts',(89.4283522643419,24.6126370463772,10.));
#30329=CARTESIAN_POINT('Ctrl Pts',(89.433519789665,24.6275520645202,10.));
#30330=CARTESIAN_POINT('Ctrl Pts',(89.4388132540751,24.642418569377,10.));
#30331=CARTESIAN_POINT('Ctrl Pts',(89.4442314704579,24.657232470925,10.));
#30332=CARTESIAN_POINT('Ctrl Pts',(89.4759375176245,24.7439197178007,10.));
#30333=CARTESIAN_POINT('Ctrl Pts',(89.511920335377,24.828832792636,10.));
#30334=CARTESIAN_POINT('Ctrl Pts',(89.5521196218609,24.9115708704841,10.));
#30335=CARTESIAN_POINT('Ctrl Pts',(89.5822690867238,24.9736244288701,10.));
#30336=CARTESIAN_POINT('Ctrl Pts',(89.6147913043791,25.0344540665882,10.));
#30337=CARTESIAN_POINT('Ctrl Pts',(89.6496759249085,25.0938756897438,10.));
#30338=CARTESIAN_POINT('Ctrl Pts',(89.6654547888551,25.1207530268921,10.));
#30339=CARTESIAN_POINT('Ctrl Pts',(89.6817171405451,25.1473421001399,10.));
#30340=CARTESIAN_POINT('Ctrl Pts',(89.6984628025478,25.1736248045378,10.));
#30341=CARTESIAN_POINT('Ctrl Pts',(89.7075848155659,25.1879420152656,10.));
#30342=CARTESIAN_POINT('Ctrl Pts',(89.7168450675973,25.2021601543536,10.));
#30343=CARTESIAN_POINT('Ctrl Pts',(89.726242878983,25.2162762092358,10.));
#30344=CARTESIAN_POINT('Ctrl Pts',(89.7738179411261,25.2877366972872,10.));
#30345=CARTESIAN_POINT('Ctrl Pts',(89.82491820811,25.3565879238984,10.));
#30346=CARTESIAN_POINT('Ctrl Pts',(89.8795126225196,25.4224764001538,10.));
#30347=CARTESIAN_POINT('Ctrl Pts',(89.9256431150503,25.4781500051302,10.));
#30348=CARTESIAN_POINT('Ctrl Pts',(89.9742689995433,25.5317079390387,10.));
#30349=CARTESIAN_POINT('Ctrl Pts',(90.0253878321675,25.58291282293,10.));
#30350=CARTESIAN_POINT('Ctrl Pts',(90.0442196215672,25.6017763129624,10.));
#30351=CARTESIAN_POINT('Ctrl Pts',(90.0633898808657,25.6203202151646,10.));
#30352=CARTESIAN_POINT('Ctrl Pts',(90.0828884583321,25.6385402287509,10.));
#30353=CARTESIAN_POINT('Origin',(92.,24.,5.));
#30354=CARTESIAN_POINT('Origin',(-92.,-24.,1.));
#30355=CARTESIAN_POINT('Ctrl Pts',(-93.913465996665,-22.364012796625,0.999999999999999));
#30356=CARTESIAN_POINT('Ctrl Pts',(-93.9756062673219,-22.422409392352,0.999999999999999));
#30357=CARTESIAN_POINT('Ctrl Pts',(-94.0343712367569,-22.4840596836639,
0.999999999999998));
#30358=CARTESIAN_POINT('Ctrl Pts',(-94.0897488672685,-22.548587241387,0.999999999999999));
#30359=CARTESIAN_POINT('Ctrl Pts',(-94.1464812232377,-22.6146933629517,
1.));
#30360=CARTESIAN_POINT('Ctrl Pts',(-94.1996589497715,-22.6838197394786,
1.));
#30361=CARTESIAN_POINT('Ctrl Pts',(-94.2492402162377,-22.7556079093562,
1.));
#30362=CARTESIAN_POINT('Ctrl Pts',(-94.2621838800318,-22.7743488976672,
0.999999999999999));
#30363=CARTESIAN_POINT('Ctrl Pts',(-94.2748822665715,-22.793271509596,0.999999999999998));
#30364=CARTESIAN_POINT('Ctrl Pts',(-94.2873342556749,-22.8123698012048,
0.999999999999998));
#30365=CARTESIAN_POINT('Ctrl Pts',(-94.2974953331826,-22.8279543973438,
0.999999999999998));
#30366=CARTESIAN_POINT('Ctrl Pts',(-94.307492770427,-22.8436568723813,1.));
#30367=CARTESIAN_POINT('Ctrl Pts',(-94.3173171317856,-22.8594594356799,
1.));
#30368=CARTESIAN_POINT('Ctrl Pts',(-94.3647643840587,-22.9357787179241,
1.));
#30369=CARTESIAN_POINT('Ctrl Pts',(-94.4082280613636,-23.0145052251332,
1.));
#30370=CARTESIAN_POINT('Ctrl Pts',(-94.4476734134146,-23.0952464698073,
1.));
#30371=CARTESIAN_POINT('Ctrl Pts',(-94.4795142529548,-23.1604219311045,
1.));
#30372=CARTESIAN_POINT('Ctrl Pts',(-94.5087362743067,-23.2269112726343,
0.999999999999997));
#30373=CARTESIAN_POINT('Ctrl Pts',(-94.5353040218407,-23.2945258806355,
0.999999999999997));
#30374=CARTESIAN_POINT('Ctrl Pts',(-94.5460285882024,-23.3218197771016,
0.999999999999996));
#30375=CARTESIAN_POINT('Ctrl Pts',(-94.5563204579687,-23.3492971889389,
0.999999999999999));
#30376=CARTESIAN_POINT('Ctrl Pts',(-94.566176508671,-23.3769462763436,0.999999999999998));
#30377=CARTESIAN_POINT('Ctrl Pts',(-94.5713946946775,-23.3915848050349,
0.999999999999998));
#30378=CARTESIAN_POINT('Ctrl Pts',(-94.5764901608952,-23.4062701280322,
1.));
#30379=CARTESIAN_POINT('Ctrl Pts',(-94.5814586868804,-23.4209886699613,
1.));
#30380=CARTESIAN_POINT('Ctrl Pts',(-94.6109727420549,-23.5084198034374,
1.));
#30381=CARTESIAN_POINT('Ctrl Pts',(-94.6360505254107,-23.5971308207555,
1.));
#30382=CARTESIAN_POINT('Ctrl Pts',(-94.6566592714401,-23.6867240276082,
1.));
#30383=CARTESIAN_POINT('Ctrl Pts',(-94.6775869561989,-23.7777037692606,
1.));
#30384=CARTESIAN_POINT('Ctrl Pts',(-94.6939067088653,-23.8695940231595,
0.999999999999999));
#30385=CARTESIAN_POINT('Ctrl Pts',(-94.705542374548,-23.9620114812617,0.999999999999998));
#30386=CARTESIAN_POINT('Ctrl Pts',(-94.7170868819221,-24.0537049052259,
0.999999999999998));
#30387=CARTESIAN_POINT('Ctrl Pts',(-94.7240207525125,-24.1459182348717,
0.999999999999998));
#30388=CARTESIAN_POINT('Ctrl Pts',(-94.7262226529554,-24.2382962599632,
0.999999999999998));
#30389=CARTESIAN_POINT('Ctrl Pts',(-94.7273178683594,-24.2842446752959,
0.999999999999998));
#30390=CARTESIAN_POINT('Ctrl Pts',(-94.7272416202326,-24.3302340487982,
0.999999999999996));
#30391=CARTESIAN_POINT('Ctrl Pts',(-94.7259741875425,-24.3762213626827,
0.999999999999996));
#30392=CARTESIAN_POINT('Ctrl Pts',(-94.7255574256381,-24.3913430813046,
0.999999999999996));
#30393=CARTESIAN_POINT('Ctrl Pts',(-94.7250117558556,-24.4064664273217,
0.999999999999996));
#30394=CARTESIAN_POINT('Ctrl Pts',(-94.7243366614637,-24.4215840497042,
0.999999999999996));
#30395=CARTESIAN_POINT('Ctrl Pts',(-94.7200628102785,-24.5172898785549,
0.999999999999996));
#30396=CARTESIAN_POINT('Ctrl Pts',(-94.7106219290546,-24.6124285315491,
0.999999999999999));
#30397=CARTESIAN_POINT('Ctrl Pts',(-94.6959498471788,-24.7066016789508,
0.999999999999998));
#30398=CARTESIAN_POINT('Ctrl Pts',(-94.6917951385598,-24.7332687866252,
0.999999999999998));
#30399=CARTESIAN_POINT('Ctrl Pts',(-94.6872206686445,-24.7598586042627,
1.));
#30400=CARTESIAN_POINT('Ctrl Pts',(-94.682224266105,-24.7863623464053,1.));
#30401=CARTESIAN_POINT('Ctrl Pts',(-94.665259332382,-24.8763539404189,1.));
#30402=CARTESIAN_POINT('Ctrl Pts',(-94.6434341104636,-24.9653530573486,
0.999999999999997));
#30403=CARTESIAN_POINT('Ctrl Pts',(-94.617051236814,-25.0531274604659,0.999999999999997));
#30404=CARTESIAN_POINT('Ctrl Pts',(-94.5900718918312,-25.1428862916612,
0.999999999999996));
#30405=CARTESIAN_POINT('Ctrl Pts',(-94.5583262747353,-25.2313651060452,
0.999999999999996));
#30406=CARTESIAN_POINT('Ctrl Pts',(-94.522083774644,-25.3183118483838,0.999999999999997));
#30407=CARTESIAN_POINT('Ctrl Pts',(-94.5094168709612,-25.3487000944476,
0.999999999999997));
#30408=CARTESIAN_POINT('Ctrl Pts',(-94.4962001982363,-25.3789011100916,
0.999999999999999));
#30409=CARTESIAN_POINT('Ctrl Pts',(-94.4824438244244,-25.4089037784715,
0.999999999999999));
#30410=CARTESIAN_POINT('Ctrl Pts',(-94.4754968108625,-25.4240552236835,
0.999999999999999));
#30411=CARTESIAN_POINT('Ctrl Pts',(-94.4684121470112,-25.4391560809515,
0.999999999999999));
#30412=CARTESIAN_POINT('Ctrl Pts',(-94.4611910621987,-25.4542048928028,
0.999999999999999));
#30413=CARTESIAN_POINT('Ctrl Pts',(-94.455180892849,-25.4667301449065,0.999999999999998));
#30414=CARTESIAN_POINT('Ctrl Pts',(-94.449078063724,-25.4792154077161,0.999999999999999));
#30415=CARTESIAN_POINT('Ctrl Pts',(-94.4428871733088,-25.4916526565279,
0.999999999999999));
#30416=CARTESIAN_POINT('Ctrl Pts',(-94.3999238161019,-25.577964305988,0.999999999999999));
#30417=CARTESIAN_POINT('Ctrl Pts',(-94.3526734205402,-25.6620692721598,
1.));
#30418=CARTESIAN_POINT('Ctrl Pts',(-94.3014780528836,-25.7437174772354,
1.));
#30419=CARTESIAN_POINT('Ctrl Pts',(-94.2492778933731,-25.8269681603301,
1.));
#30420=CARTESIAN_POINT('Ctrl Pts',(-94.1929760719894,-25.907665474163,0.999999999999999));
#30421=CARTESIAN_POINT('Ctrl Pts',(-94.1328802769678,-25.9855370030581,
1.));
#30422=CARTESIAN_POINT('Ctrl Pts',(-94.0723164763602,-26.0640149689011,
1.));
#30423=CARTESIAN_POINT('Ctrl Pts',(-94.0078989170008,-26.1396238030331,
1.));
#30424=CARTESIAN_POINT('Ctrl Pts',(-93.9398933824888,-26.2120650887426,
1.));
#30425=CARTESIAN_POINT('Ctrl Pts',(-93.9029668413288,-26.2514002125325,
1.));
#30426=CARTESIAN_POINT('Ctrl Pts',(-93.8649816076841,-26.2898009990597,
0.999999999999999));
#30427=CARTESIAN_POINT('Ctrl Pts',(-93.8259749923962,-26.3272159157843,
0.999999999999999));
#30428=CARTESIAN_POINT('Ctrl Pts',(-93.8138410590721,-26.3388547134989,
0.999999999999999));
#30429=CARTESIAN_POINT('Ctrl Pts',(-93.8016082652093,-26.3503980889207,
0.999999999999998));
#30430=CARTESIAN_POINT('Ctrl Pts',(-93.7892776690852,-26.3618444261323,
0.999999999999998));
#30431=CARTESIAN_POINT('Ctrl Pts',(-93.7779940519145,-26.372318865957,0.999999999999998));
#30432=CARTESIAN_POINT('Ctrl Pts',(-93.7666342733719,-26.3827066803521,
0.999999999999997));
#30433=CARTESIAN_POINT('Ctrl Pts',(-93.7552037473516,-26.3930030342907,
0.999999999999997));
#30434=CARTESIAN_POINT('Ctrl Pts',(-93.6793946848277,-26.4612900875824,
0.999999999999996));
#30435=CARTESIAN_POINT('Ctrl Pts',(-93.6004193335679,-26.5256101176591,
0.999999999999996));
#30436=CARTESIAN_POINT('Ctrl Pts',(-93.5186038562927,-26.5856805003819,
0.999999999999995));
#30437=CARTESIAN_POINT('Ctrl Pts',(-93.4367174573237,-26.6458029550773,
0.999999999999995));
#30438=CARTESIAN_POINT('Ctrl Pts',(-93.351985429421,-26.7016692287801,0.999999999999997));
#30439=CARTESIAN_POINT('Ctrl Pts',(-93.2646898210428,-26.752969758348,0.999999999999996));
#30440=CARTESIAN_POINT('Ctrl Pts',(-93.1791579830026,-26.8032337827119,
0.999999999999996));
#30441=CARTESIAN_POINT('Ctrl Pts',(-93.0911644456872,-26.8491153709103,
0.999999999999998));
#30442=CARTESIAN_POINT('Ctrl Pts',(-93.0009407547904,-26.8902872130475,
0.999999999999999));
#30443=CARTESIAN_POINT('Ctrl Pts',(-92.963151738466,-26.9075315022044,0.999999999999999));
#30444=CARTESIAN_POINT('Ctrl Pts',(-92.9249711428035,-26.9239490878333,
1.));
#30445=CARTESIAN_POINT('Ctrl Pts',(-92.8864145873394,-26.9395135460181,
1.));
#30446=CARTESIAN_POINT('Ctrl Pts',(-92.8564008951788,-26.9516294326938,
1.));
#30447=CARTESIAN_POINT('Ctrl Pts',(-92.8261593691066,-26.9632283272652,
0.999999999999999));
#30448=CARTESIAN_POINT('Ctrl Pts',(-92.7957017813268,-26.9743128096466,
0.999999999999999));
#30449=CARTESIAN_POINT('Ctrl Pts',(-91.2062007174671,-26.9692229537457,
1.));
#30450=CARTESIAN_POINT('Ctrl Pts',(-91.1113643951071,-26.9345314033953,
1.));
#30451=CARTESIAN_POINT('Ctrl Pts',(-91.0185713035755,-26.8948494397933,
1.));
#30452=CARTESIAN_POINT('Ctrl Pts',(-90.9280623762692,-26.8504973089265,
1.));
#30453=CARTESIAN_POINT('Ctrl Pts',(-90.8362819518266,-26.805522105739,1.));
#30454=CARTESIAN_POINT('Ctrl Pts',(-90.7468496512692,-26.755743896015,0.999999999999998));
#30455=CARTESIAN_POINT('Ctrl Pts',(-90.6600507311862,-26.7014559325823,
0.999999999999998));
#30456=CARTESIAN_POINT('Ctrl Pts',(-90.6355419727628,-26.6861270485386,
0.999999999999997));
#30457=CARTESIAN_POINT('Ctrl Pts',(-90.6112434098825,-26.6704383986501,
0.999999999999998));
#30458=CARTESIAN_POINT('Ctrl Pts',(-90.5871620603007,-26.6543961292597,
0.999999999999998));
#30459=CARTESIAN_POINT('Ctrl Pts',(-90.5678313682138,-26.6415186047294,
0.999999999999998));
#30460=CARTESIAN_POINT('Ctrl Pts',(-90.5486385360232,-26.6284115929408,
0.999999999999998));
#30461=CARTESIAN_POINT('Ctrl Pts',(-90.5296064824045,-26.6150920391085,
0.999999999999998));
#30462=CARTESIAN_POINT('Ctrl Pts',(-90.4468988471007,-26.5572092261004,
0.999999999999999));
#30463=CARTESIAN_POINT('Ctrl Pts',(-90.3671460463151,-26.4952646296917,
1.));
#30464=CARTESIAN_POINT('Ctrl Pts',(-90.2906144358446,-26.4295554859959,
1.));
#30465=CARTESIAN_POINT('Ctrl Pts',(-90.2316015873974,-26.3788877460298,
1.));
#30466=CARTESIAN_POINT('Ctrl Pts',(-90.1745046339107,-26.3259807644008,
0.999999999999999));
#30467=CARTESIAN_POINT('Ctrl Pts',(-90.1194632797683,-26.2709590345817,
0.999999999999998));
#30468=CARTESIAN_POINT('Ctrl Pts',(-90.0901431566793,-26.241649365225,0.999999999999998));
#30469=CARTESIAN_POINT('Ctrl Pts',(-90.0614066103864,-26.211739462745,1.));
#30470=CARTESIAN_POINT('Ctrl Pts',(-90.0332767877765,-26.18124731084,1.));
#30471=CARTESIAN_POINT('Ctrl Pts',(-90.0236428023317,-26.1708042678209,
1.));
#30472=CARTESIAN_POINT('Ctrl Pts',(-90.0140807815228,-26.1602937103339,
1.));
#30473=CARTESIAN_POINT('Ctrl Pts',(-90.0045982120972,-26.1497238889479,
1.));
#30474=CARTESIAN_POINT('Ctrl Pts',(-89.938805722262,-26.0763877671762,1.));
#30475=CARTESIAN_POINT('Ctrl Pts',(-89.876745482153,-26.0001052971121,1.));
#30476=CARTESIAN_POINT('Ctrl Pts',(-89.8186612830851,-25.9211548961491,
1.));
#30477=CARTESIAN_POINT('Ctrl Pts',(-89.7610834896514,-25.8428928222785,
1.));
#30478=CARTESIAN_POINT('Ctrl Pts',(-89.7074122724075,-25.762008351304,1.));
#30479=CARTESIAN_POINT('Ctrl Pts',(-89.6579309060241,-25.678750276668,1.));
#30480=CARTESIAN_POINT('Ctrl Pts',(-89.6098825260779,-25.5979033660816,
1.));
#30481=CARTESIAN_POINT('Ctrl Pts',(-89.5657846284712,-25.5148176410515,
1.));
#30482=CARTESIAN_POINT('Ctrl Pts',(-89.5259443770766,-25.4297105806844,
1.));
#30483=CARTESIAN_POINT('Ctrl Pts',(-89.5051331098887,-25.3852533869951,
1.));
#30484=CARTESIAN_POINT('Ctrl Pts',(-89.4854844375302,-25.340244525694,1.));
#30485=CARTESIAN_POINT('Ctrl Pts',(-89.4670478470478,-25.2947147599898,
1.));
#30486=CARTESIAN_POINT('Ctrl Pts',(-89.4599071766988,-25.277080640044,1.));
#30487=CARTESIAN_POINT('Ctrl Pts',(-89.4529483729289,-25.2593683810712,
1.));
#30488=CARTESIAN_POINT('Ctrl Pts',(-89.4461744795067,-25.2415797795319,
1.));
#30489=CARTESIAN_POINT('Ctrl Pts',(-89.4410205926902,-25.2280454008159,
1.));
#30490=CARTESIAN_POINT('Ctrl Pts',(-89.4359737884854,-25.2144667084508,
1.));
#30491=CARTESIAN_POINT('Ctrl Pts',(-89.4310402378581,-25.2008583977092,
1.));
#30492=CARTESIAN_POINT('Ctrl Pts',(-89.3993683880461,-25.1134973049451,
1.));
#30493=CARTESIAN_POINT('Ctrl Pts',(-89.3723052489148,-25.0247752781117,
1.));
#30494=CARTESIAN_POINT('Ctrl Pts',(-89.3501021061037,-24.9349157228039,
1.));
#30495=CARTESIAN_POINT('Ctrl Pts',(-89.3450995089376,-24.9146694378273,
1.));
#30496=CARTESIAN_POINT('Ctrl Pts',(-89.3403438330582,-24.8943653665978,
1.));
#30497=CARTESIAN_POINT('Ctrl Pts',(-89.3358383183128,-24.8740060081578,
1.));
#30498=CARTESIAN_POINT('Ctrl Pts',(-89.3154927915306,-24.7820693714308,
1.));
#30499=CARTESIAN_POINT('Ctrl Pts',(-89.3002442665944,-24.6890050257332,
1.));
#30500=CARTESIAN_POINT('Ctrl Pts',(-89.2899828336273,-24.5952047143853,
1.));
#30501=CARTESIAN_POINT('Ctrl Pts',(-89.2792696952268,-24.4972753393461,
1.));
#30502=CARTESIAN_POINT('Ctrl Pts',(-89.2739923846863,-24.3985425391207,
1.));
#30503=CARTESIAN_POINT('Ctrl Pts',(-89.2740833202269,-24.2994667952368,
1.));
#30504=CARTESIAN_POINT('Ctrl Pts',(-89.2741184401281,-24.2612030942728,
1.));
#30505=CARTESIAN_POINT('Ctrl Pts',(-89.2749548502661,-24.2228884940833,
1.));
#30506=CARTESIAN_POINT('Ctrl Pts',(-89.2765907919855,-24.1845506991706,
1.));
#30507=CARTESIAN_POINT('Ctrl Pts',(-89.2771783957763,-24.170780383667,1.));
#30508=CARTESIAN_POINT('Ctrl Pts',(-89.2778691417581,-24.1570088738121,
0.999999999999999));
#30509=CARTESIAN_POINT('Ctrl Pts',(-89.2786620584242,-24.1432491218723,
0.999999999999999));
#30510=CARTESIAN_POINT('Ctrl Pts',(-89.2840136676959,-24.0503808304004,
0.999999999999999));
#30511=CARTESIAN_POINT('Ctrl Pts',(-89.2940209876791,-23.9578996294849,
1.));
#30512=CARTESIAN_POINT('Ctrl Pts',(-89.308560961015,-23.8661774184892,1.));
#30513=CARTESIAN_POINT('Ctrl Pts',(-89.3230638861899,-23.7746889176356,
1.));
#30514=CARTESIAN_POINT('Ctrl Pts',(-89.3420768069923,-23.683954599498,1.));
#30515=CARTESIAN_POINT('Ctrl Pts',(-89.3655261935074,-23.5943606394727,
1.));
#30516=CARTESIAN_POINT('Ctrl Pts',(-89.3885742801647,-23.5062999410276,
0.999999999999999));
#30517=CARTESIAN_POINT('Ctrl Pts',(-89.415908753375,-23.41934012046,0.999999999999997));
#30518=CARTESIAN_POINT('Ctrl Pts',(-89.4475001290534,-23.3338770863052,
0.999999999999997));
#30519=CARTESIAN_POINT('Ctrl Pts',(-89.4633626084254,-23.2909648804505,
0.999999999999997));
#30520=CARTESIAN_POINT('Ctrl Pts',(-89.4802989283759,-23.2484305779728,
0.999999999999998));
#30521=CARTESIAN_POINT('Ctrl Pts',(-89.4983087451776,-23.2063280775901,
0.999999999999998));
#30522=CARTESIAN_POINT('Ctrl Pts',(-89.5036080599323,-23.1939395894702,
0.999999999999997));
#30523=CARTESIAN_POINT('Ctrl Pts',(-89.5090003327764,-23.1815885059394,
0.999999999999996));
#30524=CARTESIAN_POINT('Ctrl Pts',(-89.5144855894355,-23.1692762489132,
0.999999999999995));
#30525=CARTESIAN_POINT('Ctrl Pts',(-89.5200790131214,-23.1567211991945,
0.999999999999995));
#30526=CARTESIAN_POINT('Ctrl Pts',(-89.5257654438863,-23.1442148109042,
0.999999999999999));
#30527=CARTESIAN_POINT('Ctrl Pts',(-89.5315435926943,-23.1317604191048,
0.999999999999999));
#30528=CARTESIAN_POINT('Ctrl Pts',(-89.5690289714347,-23.0509633318206,
0.999999999999999));
#30529=CARTESIAN_POINT('Ctrl Pts',(-89.6103840527349,-22.9723231040759,
0.999999999999997));
#30530=CARTESIAN_POINT('Ctrl Pts',(-89.6555390131612,-22.8961874416404,
0.999999999999998));
#30531=CARTESIAN_POINT('Ctrl Pts',(-89.69993578728,-22.8213301551846,0.999999999999999));
#30532=CARTESIAN_POINT('Ctrl Pts',(-89.748006360481,-22.7488933635223,1.));
#30533=CARTESIAN_POINT('Ctrl Pts',(-89.7997205683589,-22.6792417324263,
1.));
#30534=CARTESIAN_POINT('Ctrl Pts',(-89.8498548288956,-22.6117180641064,
1.));
#30535=CARTESIAN_POINT('Ctrl Pts',(-89.9034139310733,-22.5468115334525,
1.));
#30536=CARTESIAN_POINT('Ctrl Pts',(-89.9603980832495,-22.4848946770453,
1.));
#30537=CARTESIAN_POINT('Ctrl Pts',(-89.9815871696769,-22.4618714052826,
1.));
#30538=CARTESIAN_POINT('Ctrl Pts',(-90.0032500737241,-22.439261946639,0.999999999999998));
#30539=CARTESIAN_POINT('Ctrl Pts',(-90.0253876448586,-22.417087121357,0.999999999999998));
#30540=CARTESIAN_POINT('Ctrl Pts',(-90.0442144350809,-22.3982286485253,
0.999999999999998));
#30541=CARTESIAN_POINT('Ctrl Pts',(-90.0633845524044,-22.3796845518288,
0.999999999999999));
#30542=CARTESIAN_POINT('Ctrl Pts',(-90.0828882653787,-22.3614597476137,
0.999999999999999));
#30543=CARTESIAN_POINT('Origin',(-92.,-24.,12.2084234471775));
#30544=CARTESIAN_POINT('Ctrl Pts',(-95.0767669904684,-23.998062685181,9.70842344717746));
#30545=CARTESIAN_POINT('Ctrl Pts',(-95.0777011675186,-23.8738981078454,
9.70197366100994));
#30546=CARTESIAN_POINT('Ctrl Pts',(-95.0146668802256,-22.7368860788636,
9.64286281975954));
#30547=CARTESIAN_POINT('Ctrl Pts',(-93.5990318095031,-20.7444872358932,
9.53109092342626));
#30548=CARTESIAN_POINT('Ctrl Pts',(-90.1476049582096,-20.8820466605266,
9.37310775817762));
#30549=CARTESIAN_POINT('Ctrl Pts',(-88.3764280027803,-23.8472850428361,
9.21512459292899));
#30550=CARTESIAN_POINT('Ctrl Pts',(-89.8919230124438,-26.9512424150719,
9.05714142768036));
#30551=CARTESIAN_POINT('Ctrl Pts',(-93.3195312348388,-27.3782236147545,
8.89915826243172));
#30552=CARTESIAN_POINT('Ctrl Pts',(-94.9608441448919,-25.4378981546874,
8.78291893559742));
#30553=CARTESIAN_POINT('Ctrl Pts',(-95.0762794797313,-24.2133137737379,
8.719340663846));
#30554=CARTESIAN_POINT('Ctrl Pts',(-95.0743676381347,-24.0026790873961,
8.70842344717746));
#30555=CARTESIAN_POINT('Ctrl Pts',(-95.0702887490763,-24.0031018432153,
9.79157655282255));
#30556=CARTESIAN_POINT('Ctrl Pts',(-95.0652853033504,-23.3096184359042,
9.75572892504928));
#30557=CARTESIAN_POINT('Ctrl Pts',(-94.4922441588307,-21.5876431146109,
9.66722024219312));
#30558=CARTESIAN_POINT('Ctrl Pts',(-91.6460838755241,-20.3911593875009,
9.5260505042541));
#30559=CARTESIAN_POINT('Ctrl Pts',(-88.7843953448966,-22.3229252160129,
9.36806733900546));
#30560=CARTESIAN_POINT('Ctrl Pts',(-88.8381771631846,-25.7771164103053,
9.21008417375683));
#30561=CARTESIAN_POINT('Ctrl Pts',(-91.7604241627304,-27.6187849549088,
9.05210100850819));
#30562=CARTESIAN_POINT('Ctrl Pts',(-94.5324624275929,-26.346888962543,8.91259846819677));
#30563=CARTESIAN_POINT('Ctrl Pts',(-95.0660798384141,-24.6595176403422,
8.82575698296822));
#30564=CARTESIAN_POINT('Ctrl Pts',(-95.0703859251749,-23.9978642356407,
8.79157655282255));
#30565=CARTESIAN_POINT('Ctrl Pts',(-90.0865340033349,-22.3640127966251,
10.));
#30566=CARTESIAN_POINT('Ctrl Pts',(-89.5452199193478,-22.9971388327508,
9.94733894491712));
#30567=CARTESIAN_POINT('Ctrl Pts',(-89.1498731367062,-24.8326003723509,
9.84201683475137));
#30568=CARTESIAN_POINT('Ctrl Pts',(-91.1420127726733,-26.8458067969655,
9.68403366950273));
#30569=CARTESIAN_POINT('Ctrl Pts',(-93.9132999553889,-26.2718355849706,
9.5260505042541));
#30570=CARTESIAN_POINT('Ctrl Pts',(-94.948715185934,-23.6401115468636,9.36806733900547));
#30571=CARTESIAN_POINT('Ctrl Pts',(-93.309764952147,-21.3334135729172,9.21008417375683));
#30572=CARTESIAN_POINT('Ctrl Pts',(-90.4827055416602,-21.4460883253215,
9.05210100850819));
#30573=CARTESIAN_POINT('Ctrl Pts',(-89.0319367161215,-23.8749113698845,
8.89411784325956));
#30574=CARTESIAN_POINT('Ctrl Pts',(-90.2732767801618,-26.4173589653305,
8.73613467801093));
#30575=CARTESIAN_POINT('Ctrl Pts',(-93.0808263815541,-26.7670987311353,
8.57815151276229));
#30576=CARTESIAN_POINT('Ctrl Pts',(-94.9080233748186,-24.6070250335036,
8.42016834751366));
#30577=CARTESIAN_POINT('Ctrl Pts',(-94.0975469404961,-21.8963395546466,
8.26218518226502));
#30578=CARTESIAN_POINT('Ctrl Pts',(-91.3845223535449,-21.0937553800026,
8.10420201701639));
#30579=CARTESIAN_POINT('Ctrl Pts',(-89.2297577260391,-22.9272296313332,
7.94621885176776));
#30580=CARTESIAN_POINT('Ctrl Pts',(-89.587697039581,-25.733745495277,7.78823568651912));
#30581=CARTESIAN_POINT('Ctrl Pts',(-92.1336776494793,-26.9676939059565,
7.63025252127048));
#30582=CARTESIAN_POINT('Ctrl Pts',(-94.5584079833073,-25.5098431949504,
7.47226935602185));
#30583=CARTESIAN_POINT('Ctrl Pts',(-94.662574994087,-22.6825129051978,7.31428619077321));
#30584=CARTESIAN_POINT('Ctrl Pts',(-92.3516955853902,-21.0501885096968,
7.15630302552458));
#30585=CARTESIAN_POINT('Ctrl Pts',(-89.7218162866321,-22.0934437553399,
6.99831986027595));
#30586=CARTESIAN_POINT('Ctrl Pts',(-89.1583273702903,-24.866010621054,6.84033669502731));
#30587=CARTESIAN_POINT('Ctrl Pts',(-91.1723325238739,-26.8530762793412,
6.68235352977868));
#30588=CARTESIAN_POINT('Ctrl Pts',(-93.9370603271938,-26.2523043781637,
6.52437036453004));
#30589=CARTESIAN_POINT('Ctrl Pts',(-94.944808298303,-23.6086155263393,6.36638719928141));
#30590=CARTESIAN_POINT('Ctrl Pts',(-93.2815146299498,-21.3199257527161,
6.20840403403277));
#30591=CARTESIAN_POINT('Ctrl Pts',(-90.4558434515285,-21.4621547971772,
6.05042086878414));
#30592=CARTESIAN_POINT('Ctrl Pts',(-89.0307749678768,-23.9062960631276,
5.8924377035355));
#30593=CARTESIAN_POINT('Ctrl Pts',(-90.2988949344083,-26.4354299979252,
5.73445453828687));
#30594=CARTESIAN_POINT('Ctrl Pts',(-93.1099752577798,-26.7555457982637,
5.57647137303824));
#30595=CARTESIAN_POINT('Ctrl Pts',(-94.9142701365137,-24.576287506837,5.4184882077896));
#30596=CARTESIAN_POINT('Ctrl Pts',(-94.0752225311475,-21.8743167768149,
5.26050504254097));
#30597=CARTESIAN_POINT('Ctrl Pts',(-91.3538772582215,-21.1004132843165,
5.10252187729234));
#30598=CARTESIAN_POINT('Ctrl Pts',(-89.218587365677,-22.9565339120964,4.94453871204369));
#30599=CARTESIAN_POINT('Ctrl Pts',(-89.6061336679679,-25.7591138972605,
4.78655554679507));
#30600=CARTESIAN_POINT('Ctrl Pts',(-92.1649984413478,-26.9661175354377,
4.62857238154642));
#30601=CARTESIAN_POINT('Ctrl Pts',(-94.574203996375,-25.4827513287052,4.4705892162978));
#30602=CARTESIAN_POINT('Ctrl Pts',(-94.6485186642022,-22.6544790580041,
4.31260605104916));
#30603=CARTESIAN_POINT('Ctrl Pts',(-92.3205365027268,-21.0466402058836,
4.15462288580052));
#30604=CARTESIAN_POINT('Ctrl Pts',(-89.7018167952366,-22.1175994942308,
3.99663972055189));
#30605=CARTESIAN_POINT('Ctrl Pts',(-89.1676276911652,-24.8959602861542,
3.83865655530326));
#30606=CARTESIAN_POINT('Ctrl Pts',(-91.2024969568081,-26.861654528766,3.68067339005462));
#30607=CARTESIAN_POINT('Ctrl Pts',(-93.960728681338,-26.2317304163556,3.52269022480599));
#30608=CARTESIAN_POINT('Ctrl Pts',(-94.9405126124961,-23.577550689598,3.36470705955735));
#30609=CARTESIAN_POINT('Ctrl Pts',(-93.2531511472893,-21.3065468104243,
3.20672389430872));
#30610=CARTESIAN_POINT('Ctrl Pts',(-90.4291390042645,-21.4785971036944,
3.04874072906008));
#30611=CARTESIAN_POINT('Ctrl Pts',(-89.0299510223576,-23.9376454841629,
2.89075756381145));
#30612=CARTESIAN_POINT('Ctrl Pts',(-90.3246996110788,-26.453252357017,2.73277439856282));
#30613=CARTESIAN_POINT('Ctrl Pts',(-93.1390012538637,-26.7436739362116,
2.57479123331418));
#30614=CARTESIAN_POINT('Ctrl Pts',(-94.9201931102794,-24.5454930206753,
2.41680806806555));
#30615=CARTESIAN_POINT('Ctrl Pts',(-94.0526635517577,-21.8525243463366,
2.25882490281691));
#30616=CARTESIAN_POINT('Ctrl Pts',(-91.3233115518592,-21.1074036232017,
2.10084173756828));
#30617=CARTESIAN_POINT('Ctrl Pts',(-89.2077115778014,-22.9859374711348,
1.94285857231964));
#30618=CARTESIAN_POINT('Ctrl Pts',(-89.624868659881,-25.7843200216543,1.78487540707101));
#30619=CARTESIAN_POINT('Ctrl Pts',(-92.1962362586587,-26.964142143379,1.62689224182237));
#30620=CARTESIAN_POINT('Ctrl Pts',(-94.5898450807176,-25.4556338347462,
1.46890907657374));
#30621=CARTESIAN_POINT('Ctrl Pts',(-94.6338976845917,-22.6263101028395,
1.3109259113251));
#30622=CARTESIAN_POINT('Ctrl Pts',(-92.2898922478439,-21.04400336112,1.15294274607647));
#30623=CARTESIAN_POINT('Ctrl Pts',(-89.6809479657765,-22.1407646543606,
0.994959580827837));
#30624=CARTESIAN_POINT('Ctrl Pts',(-89.1795854924137,-24.928282565981,0.836976415579201));
#30625=CARTESIAN_POINT('Ctrl Pts',(-90.5450731455404,-26.2169491679593,
0.731654305413445));
#30626=CARTESIAN_POINT('Ctrl Pts',(-91.3498000020249,-26.4320868020351,
0.678993250330566));
#30627=CARTESIAN_POINT('Ctrl Pts',(-89.9456684496579,-22.2435746787732,
10.1070022498898));
#30628=CARTESIAN_POINT('Ctrl Pts',(-89.3645039014938,-22.9233101920371,
10.0543411948069));
#30629=CARTESIAN_POINT('Ctrl Pts',(-88.9400524765287,-24.8938947526259,
9.94901908464118));
#30630=CARTESIAN_POINT('Ctrl Pts',(-91.0788494627237,-27.0553094224687,
9.79103591939254));
#30631=CARTESIAN_POINT('Ctrl Pts',(-94.0541532854381,-26.4390835936093,
9.63305275414391));
#30632=CARTESIAN_POINT('Ctrl Pts',(-95.1657937219657,-23.6136172760998,
9.47506958889528));
#30633=CARTESIAN_POINT('Ctrl Pts',(-93.4061872379324,-21.1371047939092,
9.31708642364664));
#30634=CARTESIAN_POINT('Ctrl Pts',(-90.3710053471766,-21.2580744370565,
9.159103258398));
#30635=CARTESIAN_POINT('Ctrl Pts',(-88.8134338116745,-23.8657025942017,
9.00112009314937));
#30636=CARTESIAN_POINT('Ctrl Pts',(-90.1461588575891,-26.5953201152443,
8.84313692790073));
#30637=CARTESIAN_POINT('Ctrl Pts',(-93.1603946659823,-26.970807025675,8.68515376265211));
#30638=CARTESIAN_POINT('Ctrl Pts',(-95.1221062608034,-24.6517130068407,
8.52717059740346));
#30639=CARTESIAN_POINT('Ctrl Pts',(-94.2519641664366,-21.741472264661,8.36918743215484));
#30640=CARTESIAN_POINT('Ctrl Pts',(-91.3392121156861,-20.8798034424033,
8.21120426690619));
#30641=CARTESIAN_POINT('Ctrl Pts',(-89.0258180101408,-22.8482544145205,
8.05322110165756));
#30642=CARTESIAN_POINT('Ctrl Pts',(-89.4101081026736,-25.861380383774,7.89523793640894));
#30643=CARTESIAN_POINT('Ctrl Pts',(-92.1435187316521,-27.186169617537,7.73725477116029));
#30644=CARTESIAN_POINT('Ctrl Pts',(-94.7467528808537,-25.6209948422715,
7.57927160591167));
#30645=CARTESIAN_POINT('Ctrl Pts',(-94.8585884593915,-22.5855221306583,
7.42128844066302));
#30646=CARTESIAN_POINT('Ctrl Pts',(-92.3775867135567,-20.8330292659221,
7.26330527541439));
#30647=CARTESIAN_POINT('Ctrl Pts',(-89.5541009414307,-21.9530868838363,
7.10532211016575));
#30648=CARTESIAN_POINT('Ctrl Pts',(-88.9491290939423,-24.9297645972614,
6.94733894491712));
#30649=CARTESIAN_POINT('Ctrl Pts',(-91.111401293589,-27.0631140696509,6.78935577966849));
#30650=CARTESIAN_POINT('Ctrl Pts',(-94.0796628484676,-26.4181145382775,
6.63137261441986));
#30651=CARTESIAN_POINT('Ctrl Pts',(-95.1615992170526,-23.5798025813071,
6.47338944917121));
#30652=CARTESIAN_POINT('Ctrl Pts',(-93.37585718331,-21.1226240272623,6.31540628392259));
#30653=CARTESIAN_POINT('Ctrl Pts',(-90.342165723498,-21.2753236905543,6.15742311867395));
#30654=CARTESIAN_POINT('Ctrl Pts',(-88.812186537839,-23.8993977660205,5.99943995342531));
#30655=CARTESIAN_POINT('Ctrl Pts',(-90.1736629693015,-26.6147215012481,
5.84145678817668));
#30656=CARTESIAN_POINT('Ctrl Pts',(-93.1916894243903,-26.9584035889072,
5.68347362292805));
#30657=CARTESIAN_POINT('Ctrl Pts',(-95.1288128966464,-24.618712644712,5.52549045767941));
#30658=CARTESIAN_POINT('Ctrl Pts',(-94.227996278558,-21.7178282138105,5.36750729243077));
#30659=CARTESIAN_POINT('Ctrl Pts',(-91.306310989512,-20.8869514883654,5.20952412718215));
#30660=CARTESIAN_POINT('Ctrl Pts',(-89.0138253101082,-22.8797160180383,
5.05154096193351));
#30661=CARTESIAN_POINT('Ctrl Pts',(-89.4299019989034,-25.8886163569595,
4.89355779668488));
#30662=CARTESIAN_POINT('Ctrl Pts',(-92.1771452978045,-27.1844771977619,
4.73557463143624));
#30663=CARTESIAN_POINT('Ctrl Pts',(-94.7637117649265,-25.5919085268197,
4.5775914661876));
#30664=CARTESIAN_POINT('Ctrl Pts',(-94.8434973305108,-22.5554244874977,
4.41960830093897));
#30665=CARTESIAN_POINT('Ctrl Pts',(-92.3441337613189,-20.8292197430529,
4.26162513569033));
#30666=CARTESIAN_POINT('Ctrl Pts',(-89.5326291273321,-21.9790209200887,
4.10364197044171));
#30667=CARTESIAN_POINT('Ctrl Pts',(-88.9591140859071,-24.961919097025,3.94565880519306));
#30668=CARTESIAN_POINT('Ctrl Pts',(-91.1437863719667,-27.0723238327043,
3.78767563994443));
#30669=CARTESIAN_POINT('Ctrl Pts',(-94.1050736196794,-26.3960259623991,
3.6296924746958));
#30670=CARTESIAN_POINT('Ctrl Pts',(-95.1569872914167,-23.5464508131884,
3.47170930944716));
#30671=CARTESIAN_POINT('Ctrl Pts',(-93.3454056375763,-21.1082601538994,
3.31372614419853));
#30672=CARTESIAN_POINT('Ctrl Pts',(-90.3134953480409,-21.2929764469124,
3.15574297894989));
#30673=CARTESIAN_POINT('Ctrl Pts',(-88.8113019350925,-23.933055068962,2.99775981370126));
#30674=CARTESIAN_POINT('Ctrl Pts',(-90.2013673348471,-26.6338559069013,
2.83977664845262));
#30675=CARTESIAN_POINT('Ctrl Pts',(-93.2228522564652,-26.9456577440281,
2.68179348320399));
#30676=CARTESIAN_POINT('Ctrl Pts',(-95.1351719079378,-24.5856511298438,
2.52381031795535));
#30677=CARTESIAN_POINT('Ctrl Pts',(-94.2037765520592,-21.6944314680265,
2.36582715270672));
#30678=CARTESIAN_POINT('Ctrl Pts',(-91.2734950967561,-20.8944564420696,
2.20784398745809));
#30679=CARTESIAN_POINT('Ctrl Pts',(-89.0021488684016,-22.9112842085,2.04986082220945));
#30680=CARTESIAN_POINT('Ctrl Pts',(-89.4500162235876,-25.9156781060025,
1.89187765696082));
#30681=CARTESIAN_POINT('Ctrl Pts',(-92.2106827809777,-27.1823563812762,
1.73389449171218));
#30682=CARTESIAN_POINT('Ctrl Pts',(-94.78050431473,-25.562794696993,1.57591132646355));
#30683=CARTESIAN_POINT('Ctrl Pts',(-94.8277999835169,-22.5251817899866,
1.41792816121491));
#30684=CARTESIAN_POINT('Ctrl Pts',(-92.3112335374568,-20.8263887790323,
1.25994499596628));
#30685=CARTESIAN_POINT('Ctrl Pts',(-89.5102239762328,-22.0038914531457,
1.10196183071765));
#30686=CARTESIAN_POINT('Ctrl Pts',(-88.971952196655,-24.9966208786834,0.943978665469012));
#30687=CARTESIAN_POINT('Ctrl Pts',(-90.4379643297735,-26.3801565479508,
0.838656555303256));
#30688=CARTESIAN_POINT('Ctrl Pts',(-91.301933573839,-26.6111321859386,0.785995500220377));
#30689=CARTESIAN_POINT('Ctrl Pts',(-89.8048028959809,-22.1231365609213,
10.2140044997796));
#30690=CARTESIAN_POINT('Ctrl Pts',(-89.1837878836397,-22.8494815513233,
10.1613434446967));
#30691=CARTESIAN_POINT('Ctrl Pts',(-88.7302318163511,-24.9551891329009,
10.056021334531));
#30692=CARTESIAN_POINT('Ctrl Pts',(-91.0156861527742,-27.2648120479719,
9.89803816928236));
#30693=CARTESIAN_POINT('Ctrl Pts',(-94.1950066154872,-26.606331602248,9.74005500403371));
#30694=CARTESIAN_POINT('Ctrl Pts',(-95.3828722579974,-23.587123005336,9.58207183878509));
#30695=CARTESIAN_POINT('Ctrl Pts',(-93.5026095237177,-20.9407960149012,
9.42408867353644));
#30696=CARTESIAN_POINT('Ctrl Pts',(-90.2593051526931,-21.0700605487915,
9.26610550828782));
#30697=CARTESIAN_POINT('Ctrl Pts',(-88.5949309072274,-23.8564938185189,
9.10812234303918));
#30698=CARTESIAN_POINT('Ctrl Pts',(-90.0190409350164,-26.7732812651581,
8.95013917779055));
#30699=CARTESIAN_POINT('Ctrl Pts',(-93.2399629504105,-27.1745153202148,
8.79215601254192));
#30700=CARTESIAN_POINT('Ctrl Pts',(-95.336189146788,-24.6964009801777,8.63417284729328));
#30701=CARTESIAN_POINT('Ctrl Pts',(-94.4063813923771,-21.5866049746754,
8.47618968204465));
#30702=CARTESIAN_POINT('Ctrl Pts',(-91.2939018778273,-20.665851504804,8.31820651679601));
#30703=CARTESIAN_POINT('Ctrl Pts',(-88.8218782942424,-22.7692791977076,
8.16022335154738));
#30704=CARTESIAN_POINT('Ctrl Pts',(-89.2325191657663,-25.9890152722711,
8.00224018629874));
#30705=CARTESIAN_POINT('Ctrl Pts',(-92.1533598138249,-27.4046453291175,
7.8442570210501));
#30706=CARTESIAN_POINT('Ctrl Pts',(-94.9350977784,-25.7321464895925,7.68627385580147));
#30707=CARTESIAN_POINT('Ctrl Pts',(-95.0546019246959,-22.4885313561187,
7.52829069055284));
#30708=CARTESIAN_POINT('Ctrl Pts',(-92.4034778417231,-20.6158700221474,
7.3703075253042));
#30709=CARTESIAN_POINT('Ctrl Pts',(-89.3863855962295,-21.8127300123327,
7.21232436005556));
#30710=CARTESIAN_POINT('Ctrl Pts',(-88.7399308175942,-24.9935185734687,
7.05434119480694));
#30711=CARTESIAN_POINT('Ctrl Pts',(-91.0504700633043,-27.2731518599606,
6.89635802955829));
#30712=CARTESIAN_POINT('Ctrl Pts',(-94.2222653697412,-26.5839246983912,
6.73837486430967));
#30713=CARTESIAN_POINT('Ctrl Pts',(-95.3783901358023,-23.5509896362749,
6.58039169906103));
#30714=CARTESIAN_POINT('Ctrl Pts',(-93.47019973667,-20.9253223018085,6.4224085338124));
#30715=CARTESIAN_POINT('Ctrl Pts',(-90.2284879954676,-21.0884925839313,
6.26442536856376));
#30716=CARTESIAN_POINT('Ctrl Pts',(-88.5935981078011,-23.8924994689134,
6.10644220331513));
#30717=CARTESIAN_POINT('Ctrl Pts',(-90.0484310041948,-26.794013004571,5.94845903806649));
#30718=CARTESIAN_POINT('Ctrl Pts',(-93.2734035910007,-27.1612613795506,
5.79047587281786));
#30719=CARTESIAN_POINT('Ctrl Pts',(-95.343355656779,-24.6611377825871,5.63249270756922));
#30720=CARTESIAN_POINT('Ctrl Pts',(-94.3807700259685,-21.561339650806,5.47450954232059));
#30721=CARTESIAN_POINT('Ctrl Pts',(-91.2587447208024,-20.6734896924144,
5.31652637707195));
#30722=CARTESIAN_POINT('Ctrl Pts',(-88.8090632545394,-22.8028981239801,
5.15854321182332));
#30723=CARTESIAN_POINT('Ctrl Pts',(-89.2536703298387,-26.0181188166585,
5.00056004657469));
#30724=CARTESIAN_POINT('Ctrl Pts',(-92.1892921542613,-27.4028368600861,
4.84257688132605));
#30725=CARTESIAN_POINT('Ctrl Pts',(-94.9532195334778,-25.7010657249343,
4.68459371607742));
#30726=CARTESIAN_POINT('Ctrl Pts',(-95.0384759968196,-22.4563699169912,
4.52661055082878));
#30727=CARTESIAN_POINT('Ctrl Pts',(-92.3677310199108,-20.6117992802222,
4.36862738558014));
#30728=CARTESIAN_POINT('Ctrl Pts',(-89.3634414594277,-21.8404423459467,
4.21064422033152));
#30729=CARTESIAN_POINT('Ctrl Pts',(-88.7506004806488,-25.0278779078958,
4.05266105508288));
#30730=CARTESIAN_POINT('Ctrl Pts',(-91.0850757871254,-27.2829931366426,
3.89467788983424));
#30731=CARTESIAN_POINT('Ctrl Pts',(-94.2494185580209,-26.5603215084426,
3.73669472458561));
#30732=CARTESIAN_POINT('Ctrl Pts',(-95.3734619703373,-23.5153509367788,
3.57871155933698));
#30733=CARTESIAN_POINT('Ctrl Pts',(-93.4376601278633,-20.9099734973745,
3.42072839408834));
#30734=CARTESIAN_POINT('Ctrl Pts',(-90.1978516918172,-21.1073557901305,
3.26274522883971));
#30735=CARTESIAN_POINT('Ctrl Pts',(-88.5926528478276,-23.9284646537609,
3.10476206359107));
#30736=CARTESIAN_POINT('Ctrl Pts',(-90.0780350586153,-26.8144594567857,
2.94677889834244));
#30737=CARTESIAN_POINT('Ctrl Pts',(-93.3067032590667,-27.1476415518445,
2.7887957330938));
#30738=CARTESIAN_POINT('Ctrl Pts',(-95.3501507055962,-24.6258092390124,
2.63081256784517));
#30739=CARTESIAN_POINT('Ctrl Pts',(-94.3548895523608,-21.5363385897164,
2.47282940259653));
#30740=CARTESIAN_POINT('Ctrl Pts',(-91.2236786416529,-20.6815092609376,
2.3148462373479));
#30741=CARTESIAN_POINT('Ctrl Pts',(-88.7965861590017,-22.8366309458653,
2.15686307209926));
#30742=CARTESIAN_POINT('Ctrl Pts',(-89.2751637872942,-26.0470361903507,
1.99887990685063));
#30743=CARTESIAN_POINT('Ctrl Pts',(-92.2251293032968,-27.4005706191735,
1.84089674160199));
#30744=CARTESIAN_POINT('Ctrl Pts',(-94.9711635487424,-25.6699555592398,
1.68291357635336));
#30745=CARTESIAN_POINT('Ctrl Pts',(-95.0217022824422,-22.4240534771338,
1.52493041110472));
#30746=CARTESIAN_POINT('Ctrl Pts',(-92.3325748270696,-20.6087741969446,
1.36694724585609));
#30747=CARTESIAN_POINT('Ctrl Pts',(-89.3394999866892,-21.8670182519308,
1.20896408060746));
#30748=CARTESIAN_POINT('Ctrl Pts',(-88.7643189008962,-25.0649591913859,
1.05098091535882));
#30749=CARTESIAN_POINT('Ctrl Pts',(-90.3308555140066,-26.5433639279422,
0.945658805193066));
#30750=CARTESIAN_POINT('Ctrl Pts',(-91.2540671456531,-26.7901775698422,
0.892997750110188));
#30751=CARTESIAN_POINT('Ctrl Pts',(-89.6639373423038,-22.0026984430694,
10.3210067496694));
#30752=CARTESIAN_POINT('Ctrl Pts',(-89.0030718657857,-22.7756529106096,
10.2683456945866));
#30753=CARTESIAN_POINT('Ctrl Pts',(-88.5204111561735,-25.0164835131759,
10.1630235844208));
#30754=CARTESIAN_POINT('Ctrl Pts',(-90.9525228428247,-27.4743146734751,
10.0050404191722));
#30755=CARTESIAN_POINT('Ctrl Pts',(-94.3358599455364,-26.7735796108866,
9.84705725392353));
#30756=CARTESIAN_POINT('Ctrl Pts',(-95.599950794029,-23.5606287345722,9.6890740886749));
#30757=CARTESIAN_POINT('Ctrl Pts',(-93.5990318095031,-20.7444872358932,
9.53109092342626));
#30758=CARTESIAN_POINT('Ctrl Pts',(-90.1476049582096,-20.8820466605266,
9.37310775817762));
#30759=CARTESIAN_POINT('Ctrl Pts',(-88.3764280027803,-23.8472850428361,
9.21512459292899));
#30760=CARTESIAN_POINT('Ctrl Pts',(-89.8919230124438,-26.9512424150719,
9.05714142768036));
#30761=CARTESIAN_POINT('Ctrl Pts',(-93.3195312348388,-27.3782236147545,
8.89915826243172));
#30762=CARTESIAN_POINT('Ctrl Pts',(-95.5502720327727,-24.7410889535148,
8.74117509718309));
#30763=CARTESIAN_POINT('Ctrl Pts',(-94.5607986183176,-21.4317376846898,
8.58319193193445));
#30764=CARTESIAN_POINT('Ctrl Pts',(-91.2485916399685,-20.4518995672047,
8.42520876668582));
#30765=CARTESIAN_POINT('Ctrl Pts',(-88.6179385783441,-22.6903039808949,
8.26722560143718));
#30766=CARTESIAN_POINT('Ctrl Pts',(-89.0549302288588,-26.1166501607681,
8.10924243618856));
#30767=CARTESIAN_POINT('Ctrl Pts',(-92.1632008959979,-27.623121040698,7.95125927093991));
#30768=CARTESIAN_POINT('Ctrl Pts',(-95.1234426759463,-25.8432981369136,
7.79327610569129));
#30769=CARTESIAN_POINT('Ctrl Pts',(-95.2506153900005,-22.3915405815791,
7.63529294044264));
#30770=CARTESIAN_POINT('Ctrl Pts',(-92.4293689698895,-20.3987107783727,
7.47730977519402));
#30771=CARTESIAN_POINT('Ctrl Pts',(-89.2186702510282,-21.6723731408291,
7.31932660994537));
#30772=CARTESIAN_POINT('Ctrl Pts',(-88.5307325412461,-25.0572725496761,
7.16134344469675));
#30773=CARTESIAN_POINT('Ctrl Pts',(-90.9895388330194,-27.4831896502702,
7.0033602794481));
#30774=CARTESIAN_POINT('Ctrl Pts',(-94.364867891015,-26.749734858505,6.84537711419948));
#30775=CARTESIAN_POINT('Ctrl Pts',(-95.5951810545519,-23.5221766912428,
6.68739394895083));
#30776=CARTESIAN_POINT('Ctrl Pts',(-93.5645422900301,-20.7280205763547,
6.52941078370221));
#30777=CARTESIAN_POINT('Ctrl Pts',(-90.1148102674372,-20.9016614773084,
6.37142761845357));
#30778=CARTESIAN_POINT('Ctrl Pts',(-88.3750096777633,-23.8856011718064,
6.21344445320494));
#30779=CARTESIAN_POINT('Ctrl Pts',(-89.9231990390881,-26.973304507894,6.0554612879563));
#30780=CARTESIAN_POINT('Ctrl Pts',(-93.3551177576112,-27.364119170194,5.89747812270767));
#30781=CARTESIAN_POINT('Ctrl Pts',(-95.5578984169116,-24.7035629204622,
5.73949495745903));
#30782=CARTESIAN_POINT('Ctrl Pts',(-94.5335437733791,-21.4048510878016,
5.5815117922104));
#30783=CARTESIAN_POINT('Ctrl Pts',(-91.2111784520928,-20.4600278964634,
5.42352862696177));
#30784=CARTESIAN_POINT('Ctrl Pts',(-88.6043011989707,-22.7260802299219,
5.26554546171313));
#30785=CARTESIAN_POINT('Ctrl Pts',(-89.0774386607742,-26.1476212763575,
5.1075622964645));
#30786=CARTESIAN_POINT('Ctrl Pts',(-92.201439010718,-27.6211965224103,4.94957913121586));
#30787=CARTESIAN_POINT('Ctrl Pts',(-95.1427273020293,-25.8102229230488,
4.79159596596723));
#30788=CARTESIAN_POINT('Ctrl Pts',(-95.2334546631283,-22.3573153464848,
4.63361280071859));
#30789=CARTESIAN_POINT('Ctrl Pts',(-92.3913282785029,-20.3943788173916,
4.47562963546995));
#30790=CARTESIAN_POINT('Ctrl Pts',(-89.1942537915232,-21.7018637718047,
4.31764647022133));
#30791=CARTESIAN_POINT('Ctrl Pts',(-88.5420868753907,-25.0938367187666,
4.15966330497269));
#30792=CARTESIAN_POINT('Ctrl Pts',(-91.0263652022841,-27.4936624405808,
4.00168013972406));
#30793=CARTESIAN_POINT('Ctrl Pts',(-94.3937634963622,-26.7246170544862,
3.84369697447542));
#30794=CARTESIAN_POINT('Ctrl Pts',(-95.589936649258,-23.4842510603692,3.68571380922678));
#30795=CARTESIAN_POINT('Ctrl Pts',(-93.5299146181504,-20.7116868408496,
3.52773064397815));
#30796=CARTESIAN_POINT('Ctrl Pts',(-90.0822080355936,-20.9217351333484,
3.36974747872952));
#30797=CARTESIAN_POINT('Ctrl Pts',(-88.3740037605625,-23.92387423856,3.21176431348088));
#30798=CARTESIAN_POINT('Ctrl Pts',(-89.9547027823836,-26.99506300667,3.05378114823225));
#30799=CARTESIAN_POINT('Ctrl Pts',(-93.3905542616683,-27.349625359661,2.89579798298362));
#30800=CARTESIAN_POINT('Ctrl Pts',(-95.5651295032547,-24.6659673481809,
2.73781481773498));
#30801=CARTESIAN_POINT('Ctrl Pts',(-94.5060025526623,-21.3782457114063,
2.57983165248635));
#30802=CARTESIAN_POINT('Ctrl Pts',(-91.1738621865499,-20.4685620798055,
2.42184848723771));
#30803=CARTESIAN_POINT('Ctrl Pts',(-88.5910234496018,-22.7619776832305,
2.26386532198907));
#30804=CARTESIAN_POINT('Ctrl Pts',(-89.1003113510008,-26.1783942746989,
2.10588215674044));
#30805=CARTESIAN_POINT('Ctrl Pts',(-92.2395758256157,-27.6187848570707,
1.94789899149181));
#30806=CARTESIAN_POINT('Ctrl Pts',(-95.1618227827549,-25.7771164214866,
1.78991582624317));
#30807=CARTESIAN_POINT('Ctrl Pts',(-95.2156045813675,-22.3229251642809,
1.63193266099454));
#30808=CARTESIAN_POINT('Ctrl Pts',(-92.3539161166825,-20.3911596148569,
1.4739494957459));
#30809=CARTESIAN_POINT('Ctrl Pts',(-89.1687759971456,-21.7301450507159,
1.31596633049727));
#30810=CARTESIAN_POINT('Ctrl Pts',(-88.5566856051374,-25.1332975040883,
1.15798316524863));
#30811=CARTESIAN_POINT('Ctrl Pts',(-90.2237466982397,-26.7065713079336,
1.05266105508288));
#30812=CARTESIAN_POINT('Ctrl Pts',(-91.2062007174672,-26.9692229537457,
0.999999999999999));
#30813=CARTESIAN_POINT('Ctrl Pts',(-90.0865340033349,-22.3640127966251,
10.));
#30814=CARTESIAN_POINT('Ctrl Pts',(-90.0249229041799,-22.4219121010796,
10.));
#30815=CARTESIAN_POINT('Ctrl Pts',(-89.9666809070904,-22.4829619660083,
10.));
#30816=CARTESIAN_POINT('Ctrl Pts',(-89.9118056829848,-22.546777615348,10.));
#30817=CARTESIAN_POINT('Ctrl Pts',(-89.8554777542744,-22.6122826479962,
10.));
#30818=CARTESIAN_POINT('Ctrl Pts',(-89.8026967773227,-22.6807022716026,
10.));
#30819=CARTESIAN_POINT('Ctrl Pts',(-89.753485740358,-22.7516688868598,10.));
#30820=CARTESIAN_POINT('Ctrl Pts',(-89.7029132366753,-22.8245988560865,
10.));
#30821=CARTESIAN_POINT('Ctrl Pts',(-89.6561104020014,-22.9002192512329,
10.));
#30822=CARTESIAN_POINT('Ctrl Pts',(-89.6131362838785,-22.9781741250528,
10.));
#30823=CARTESIAN_POINT('Ctrl Pts',(-89.5942448480481,-23.0124431120793,
10.));
#30824=CARTESIAN_POINT('Ctrl Pts',(-89.5760937898788,-23.0471637309785,
10.));
#30825=CARTESIAN_POINT('Ctrl Pts',(-89.5586905433103,-23.0823078140373,
10.));
#30826=CARTESIAN_POINT('Ctrl Pts',(-89.5487655216206,-23.1023503839827,
10.));
#30827=CARTESIAN_POINT('Ctrl Pts',(-89.539083745551,-23.1225307016013,10.));
#30828=CARTESIAN_POINT('Ctrl Pts',(-89.5296468276356,-23.1428436902047,
10.));
#30829=CARTESIAN_POINT('Ctrl Pts',(-89.521129801935,-23.1611766085942,10.));
#30830=CARTESIAN_POINT('Ctrl Pts',(-89.512809840989,-23.1796233419582,10.));
#30831=CARTESIAN_POINT('Ctrl Pts',(-89.504701824908,-23.1981483273657,10.));
#30832=CARTESIAN_POINT('Ctrl Pts',(-89.4681370588538,-23.2816905590052,
10.));
#30833=CARTESIAN_POINT('Ctrl Pts',(-89.4358326118623,-23.3669162866866,
10.));
#30834=CARTESIAN_POINT('Ctrl Pts',(-89.4078135857242,-23.4534267953981,
10.));
#30835=CARTESIAN_POINT('Ctrl Pts',(-89.3793318743352,-23.5413658739758,
10.));
#30836=CARTESIAN_POINT('Ctrl Pts',(-89.3552777914497,-23.6306332708035,
10.));
#30837=CARTESIAN_POINT('Ctrl Pts',(-89.3357167786194,-23.7208473130613,
10.));
#30838=CARTESIAN_POINT('Ctrl Pts',(-89.316736346674,-23.8083837563144,10.));
#30839=CARTESIAN_POINT('Ctrl Pts',(-89.301986069027,-23.8968124020132,10.));
#30840=CARTESIAN_POINT('Ctrl Pts',(-89.2915665512199,-23.9858064657529,
10.));
#30841=CARTESIAN_POINT('Ctrl Pts',(-89.2872071979636,-24.0230401044627,
10.));
#30842=CARTESIAN_POINT('Ctrl Pts',(-89.2836064360708,-24.0603729082217,
10.));
#30843=CARTESIAN_POINT('Ctrl Pts',(-89.2807739547576,-24.0977815591893,
10.));
#30844=CARTESIAN_POINT('Ctrl Pts',(-89.2790033727378,-24.1211656798468,
10.));
#30845=CARTESIAN_POINT('Ctrl Pts',(-89.2775330236662,-24.1445794431293,
10.));
#30846=CARTESIAN_POINT('Ctrl Pts',(-89.2763655644993,-24.1680171857739,
10.));
#30847=CARTESIAN_POINT('Ctrl Pts',(-89.275681297243,-24.181754436983,10.));
#30848=CARTESIAN_POINT('Ctrl Pts',(-89.2751013563383,-24.1954953573145,
10.));
#30849=CARTESIAN_POINT('Ctrl Pts',(-89.2746262639892,-24.2092305722781,
10.));
#30850=CARTESIAN_POINT('Ctrl Pts',(-89.2712684324413,-24.3063075683927,
10.));
#30851=CARTESIAN_POINT('Ctrl Pts',(-89.2731377894335,-24.4032200225579,
10.));
#30852=CARTESIAN_POINT('Ctrl Pts',(-89.2802991313706,-24.4995456759757,
10.));
#30853=CARTESIAN_POINT('Ctrl Pts',(-89.2874604733076,-24.5958713293936,
10.));
#30854=CARTESIAN_POINT('Ctrl Pts',(-89.2999133653215,-24.6916112365764,
10.));
#30855=CARTESIAN_POINT('Ctrl Pts',(-89.3177754963829,-24.7863620775548,
10.));
#30856=CARTESIAN_POINT('Ctrl Pts',(-89.3348530128177,-24.8769508789953,
10.));
#30857=CARTESIAN_POINT('Ctrl Pts',(-89.3568748775387,-24.9666365695192,
10.));
#30858=CARTESIAN_POINT('Ctrl Pts',(-89.383566394629,-25.0551798098077,10.));
#30859=CARTESIAN_POINT('Ctrl Pts',(-89.3925012626259,-25.0848192702146,
10.));
#30860=CARTESIAN_POINT('Ctrl Pts',(-89.4019598223816,-25.1143306773261,
10.));
#30861=CARTESIAN_POINT('Ctrl Pts',(-89.4119330456345,-25.1437048746548,
10.));
#30862=CARTESIAN_POINT('Ctrl Pts',(-89.4184142793766,-25.1627940932605,
10.));
#30863=CARTESIAN_POINT('Ctrl Pts',(-89.425112879774,-25.1818253626315,10.));
#30864=CARTESIAN_POINT('Ctrl Pts',(-89.4320265054004,-25.2007961347361,
10.));
#30865=CARTESIAN_POINT('Ctrl Pts',(-89.4386160834063,-25.218877730323,10.));
#30866=CARTESIAN_POINT('Ctrl Pts',(-89.4454027538168,-25.2369085767948,
10.));
#30867=CARTESIAN_POINT('Ctrl Pts',(-89.4523736969164,-25.254859317182,10.));
#30868=CARTESIAN_POINT('Ctrl Pts',(-89.4862171782651,-25.342009009671,10.));
#30869=CARTESIAN_POINT('Ctrl Pts',(-89.524439002612,-25.4273844054574,10.));
#30870=CARTESIAN_POINT('Ctrl Pts',(-89.5667079861147,-25.5107518898734,
10.));
#30871=CARTESIAN_POINT('Ctrl Pts',(-89.6105462295904,-25.5972144394055,
10.));
#30872=CARTESIAN_POINT('Ctrl Pts',(-89.6587378392776,-25.6815179448506,
10.));
#30873=CARTESIAN_POINT('Ctrl Pts',(-89.7109693334073,-25.763398787929,10.));
#30874=CARTESIAN_POINT('Ctrl Pts',(-89.7637892526335,-25.846202077202,10.));
#30875=CARTESIAN_POINT('Ctrl Pts',(-89.8207410024605,-25.9265286303401,
10.));
#30876=CARTESIAN_POINT('Ctrl Pts',(-89.8815521717527,-26.004090973277,10.));
#30877=CARTESIAN_POINT('Ctrl Pts',(-89.923214641541,-26.0572298753393,10.));
#30878=CARTESIAN_POINT('Ctrl Pts',(-89.9666897223643,-26.1090710102662,
10.));
#30879=CARTESIAN_POINT('Ctrl Pts',(-90.011902026058,-26.1595148904434,10.));
#30880=CARTESIAN_POINT('Ctrl Pts',(-90.0240091589916,-26.1730229560162,
10.));
#30881=CARTESIAN_POINT('Ctrl Pts',(-90.0362421971691,-26.1864320425439,
10.));
#30882=CARTESIAN_POINT('Ctrl Pts',(-90.0485860743795,-26.1997257420871,
10.));
#30883=CARTESIAN_POINT('Ctrl Pts',(-90.1172469210647,-26.2736698238907,
10.));
#30884=CARTESIAN_POINT('Ctrl Pts',(-90.1894216590749,-26.3441460197638,
10.));
#30885=CARTESIAN_POINT('Ctrl Pts',(-90.2647998274612,-26.410864519058,10.));
#30886=CARTESIAN_POINT('Ctrl Pts',(-90.3277047217017,-26.4665427111901,
10.));
#30887=CARTESIAN_POINT('Ctrl Pts',(-90.3928416636536,-26.5196039171212,
10.));
#30888=CARTESIAN_POINT('Ctrl Pts',(-90.4600538825085,-26.569865931641,10.));
#30889=CARTESIAN_POINT('Ctrl Pts',(-90.4819361594316,-26.5862297318424,
10.));
#30890=CARTESIAN_POINT('Ctrl Pts',(-90.5040385610053,-26.6022967069767,
10.));
#30891=CARTESIAN_POINT('Ctrl Pts',(-90.5263561031203,-26.6180601837049,
10.));
#30892=CARTESIAN_POINT('Ctrl Pts',(-90.5491249077408,-26.6341423992068,
10.));
#30893=CARTESIAN_POINT('Ctrl Pts',(-90.5721230553218,-26.6499121465391,
10.));
#30894=CARTESIAN_POINT('Ctrl Pts',(-90.5953161168769,-26.6653431122229,
10.));
#30895=CARTESIAN_POINT('Ctrl Pts',(-90.680261445699,-26.7218595169649,10.));
#30896=CARTESIAN_POINT('Ctrl Pts',(-90.7678730457073,-26.7738754900865,
10.));
#30897=CARTESIAN_POINT('Ctrl Pts',(-90.8578606519112,-26.8210829660107,
10.));
#30898=CARTESIAN_POINT('Ctrl Pts',(-90.9411342810838,-26.8647682912474,
10.));
#30899=CARTESIAN_POINT('Ctrl Pts',(-91.0264434122842,-26.9043361313708,
10.));
#30900=CARTESIAN_POINT('Ctrl Pts',(-91.1135854408295,-26.9395135107767,
10.));
#30901=CARTESIAN_POINT('Ctrl Pts',(-91.1436093918511,-26.9516335398141,
10.));
#30902=CARTESIAN_POINT('Ctrl Pts',(-91.173851123563,-26.9632321026033,10.));
#30903=CARTESIAN_POINT('Ctrl Pts',(-91.2042982523172,-26.9743127795766,
10.));
#30904=CARTESIAN_POINT('Ctrl Pts',(-94.5182106813093,-24.0021944371302,
8.38741669750803));
#30905=CARTESIAN_POINT('Ctrl Pts',(-94.5197766683662,-24.1747250448626,
8.39833391417657));
#30906=CARTESIAN_POINT('Ctrl Pts',(-94.5035406983691,-24.3469627335709,
8.40925113084511));
#30907=CARTESIAN_POINT('Ctrl Pts',(-94.4684111368875,-24.5152564032994,
8.42016834751366));
#30908=CARTESIAN_POINT('Ctrl Pts',(-94.2989577103971,-25.3270495993809,
8.47282940259654));
#30909=CARTESIAN_POINT('Ctrl Pts',(-93.6898920459757,-26.0470741652581,
8.52549045767941));
#30910=CARTESIAN_POINT('Ctrl Pts',(-92.9174342801995,-26.3487964872292,
8.57815151276229));
#30911=CARTESIAN_POINT('Ctrl Pts',(-92.1449765144234,-26.6505188092004,
8.63081256784517));
#30912=CARTESIAN_POINT('Ctrl Pts',(-91.2091266472926,-26.5339388872655,
8.68347362292805));
#30913=CARTESIAN_POINT('Ctrl Pts',(-90.5343117030538,-26.0519076603903,
8.73613467801093));
#30914=CARTESIAN_POINT('Ctrl Pts',(-89.859496758815,-25.5698764335152,8.7887957330938));
#30915=CARTESIAN_POINT('Ctrl Pts',(-89.4457167374682,-24.7223939016998,
8.84145678817668));
#30916=CARTESIAN_POINT('Ctrl Pts',(-89.4806215310513,-23.8938487950316,
8.89411784325956));
#30917=CARTESIAN_POINT('Ctrl Pts',(-89.5155263246344,-23.0653036883635,
8.94677889834244));
#30918=CARTESIAN_POINT('Ctrl Pts',(-89.9991159331473,-22.2556960068425,
8.99943995342531));
#30919=CARTESIAN_POINT('Ctrl Pts',(-90.7120873058182,-21.8321130406813,
9.05210100850819));
#30920=CARTESIAN_POINT('Ctrl Pts',(-91.4250586784891,-21.4085300745201,
9.10476206359107));
#30921=CARTESIAN_POINT('Ctrl Pts',(-92.3674118153181,-21.3709718237187,
9.15742311867395));
#30922=CARTESIAN_POINT('Ctrl Pts',(-93.1117467560304,-21.7366423606423,
9.21008417375683));
#30923=CARTESIAN_POINT('Ctrl Pts',(-93.8560816967427,-22.102312897566,9.26274522883971));
#30924=CARTESIAN_POINT('Ctrl Pts',(-94.4023984413383,-22.8712122222148,
9.31540628392259));
#30925=CARTESIAN_POINT('Ctrl Pts',(-94.5029876085453,-23.6942825575571,
9.36806733900547));
#30926=CARTESIAN_POINT('Ctrl Pts',(-94.5153075025967,-23.7950900262915,
9.37451712517299));
#30927=CARTESIAN_POINT('Ctrl Pts',(-94.520941171052,-23.8967100980969,9.38096691134051));
#30928=CARTESIAN_POINT('Ctrl Pts',(-94.5201759878003,-23.9984131478585,
9.38741669750803));
#30929=CARTESIAN_POINT('Ctrl Pts',(-92.7937992825329,-26.9692229537457,
10.));
#30930=CARTESIAN_POINT('Ctrl Pts',(-93.7762533017603,-26.7065713079336,
9.94733894491712));
#30931=CARTESIAN_POINT('Ctrl Pts',(-95.4433142859563,-25.1332967687399,
9.84201683475136));
#30932=CARTESIAN_POINT('Ctrl Pts',(-94.8312240969781,-21.7301452717063,
9.68403366950273));
#30933=CARTESIAN_POINT('Ctrl Pts',(-91.6460838755241,-20.3911593875009,
9.5260505042541));
#30934=CARTESIAN_POINT('Ctrl Pts',(-88.7843953448966,-22.3229252160129,
9.36806733900546));
#30935=CARTESIAN_POINT('Ctrl Pts',(-88.8381771631846,-25.7771164103053,
9.21008417375683));
#30936=CARTESIAN_POINT('Ctrl Pts',(-91.7604241627304,-27.6187849549088,
9.05210100850819));
#30937=CARTESIAN_POINT('Ctrl Pts',(-94.8996887115742,-26.1783943047283,
8.89411784325956));
#30938=CARTESIAN_POINT('Ctrl Pts',(-95.4089766159342,-22.7619776656796,
8.73613467801093));
#30939=CARTESIAN_POINT('Ctrl Pts',(-92.8261378316182,-20.4685620052276,
8.57815151276229));
#30940=CARTESIAN_POINT('Ctrl Pts',(-89.493997396212,-21.3782456609066,8.42016834751365));
#30941=CARTESIAN_POINT('Ctrl Pts',(-88.4348704258472,-24.6659673604642,
8.26218518226502));
#30942=CARTESIAN_POINT('Ctrl Pts',(-90.6094457101907,-27.3496254273118,
8.10420201701639));
#30943=CARTESIAN_POINT('Ctrl Pts',(-94.045297258743,-26.9950630663804,7.94621885176775));
#30944=CARTESIAN_POINT('Ctrl Pts',(-95.6259963119894,-23.9238742371833,
7.78823568651911));
#30945=CARTESIAN_POINT('Ctrl Pts',(-93.9177920028682,-20.9217350716083,
7.63025252127049));
#30946=CARTESIAN_POINT('Ctrl Pts',(-90.4700853511787,-20.7116867750179,
7.47226935602185));
#30947=CARTESIAN_POINT('Ctrl Pts',(-88.4100632788413,-23.4842510500175,
7.31428619077322));
#30948=CARTESIAN_POINT('Ctrl Pts',(-89.6062364556796,-26.7246171090759,
7.15630302552458));
#30949=CARTESIAN_POINT('Ctrl Pts',(-92.9736348172232,-27.4936625105602,
6.99831986027594));
#30950=CARTESIAN_POINT('Ctrl Pts',(-95.4579131938762,-25.0938367406809,
6.84033669502731));
#30951=CARTESIAN_POINT('Ctrl Pts',(-94.805746264682,-21.7018637257672,6.68235352977868));
#30952=CARTESIAN_POINT('Ctrl Pts',(-91.6086717136577,-20.3943787451648,
6.52437036453004));
#30953=CARTESIAN_POINT('Ctrl Pts',(-88.7665452720996,-22.3573153135784,
6.36638719928141));
#30954=CARTESIAN_POINT('Ctrl Pts',(-88.8572726350159,-25.8102229593112,
6.20840403403277));
#30955=CARTESIAN_POINT('Ctrl Pts',(-91.7985609852469,-27.6211965949497,
6.05042086878414));
#30956=CARTESIAN_POINT('Ctrl Pts',(-94.9225613977702,-26.1476213193785,
5.8924377035355));
#30957=CARTESIAN_POINT('Ctrl Pts',(-95.3956988690517,-22.7260802044028,
5.73445453828687));
#30958=CARTESIAN_POINT('Ctrl Pts',(-92.7888215637087,-20.460027825551,5.57647137303824));
#30959=CARTESIAN_POINT('Ctrl Pts',(-89.4664561758693,-21.4048510358159,
5.4184882077896));
#30960=CARTESIAN_POINT('Ctrl Pts',(-88.4421015118167,-24.7035629345559,
5.26050504254097));
#30961=CARTESIAN_POINT('Ctrl Pts',(-90.6448822152433,-27.3641192375838,
5.10252187729233));
#30962=CARTESIAN_POINT('Ctrl Pts',(-94.0768010025145,-26.9733045674549,
4.9445387120437));
#30963=CARTESIAN_POINT('Ctrl Pts',(-95.6249903948519,-23.8856011695146,
4.78655554679506));
#30964=CARTESIAN_POINT('Ctrl Pts',(-93.885189770327,-20.9016614152429,4.62857238154643));
#30965=CARTESIAN_POINT('Ctrl Pts',(-90.435457678629,-20.7280205108105,4.47058921629779));
#30966=CARTESIAN_POINT('Ctrl Pts',(-88.4048188734298,-23.5221766816715,
4.31260605104916));
#30967=CARTESIAN_POINT('Ctrl Pts',(-89.6351320616122,-26.7497349135866,
4.15462288580052));
#30968=CARTESIAN_POINT('Ctrl Pts',(-93.0104611872221,-27.4831897200468,
3.99663972055189));
#30969=CARTESIAN_POINT('Ctrl Pts',(-95.4692675282499,-25.0572725708519,
3.83865655530325));
#30970=CARTESIAN_POINT('Ctrl Pts',(-94.7813298046868,-21.6723730942086,
3.68067339005462));
#30971=CARTESIAN_POINT('Ctrl Pts',(-91.5706310215098,-20.3987107062197,
3.52269022480599));
#30972=CARTESIAN_POINT('Ctrl Pts',(-88.7493845448822,-22.3915405493825,
3.36470705955735));
#30973=CARTESIAN_POINT('Ctrl Pts',(-88.8765572614881,-25.8432981737925,
3.20672389430872));
#30974=CARTESIAN_POINT('Ctrl Pts',(-91.8367991007263,-27.6231211133645,
3.04874072906008));
#30975=CARTESIAN_POINT('Ctrl Pts',(-94.9450698301517,-26.1166502029989,
2.89075756381145));
#30976=CARTESIAN_POINT('Ctrl Pts',(-95.3820614893708,-22.6903039549832,
2.73277439856281));
#30977=CARTESIAN_POINT('Ctrl Pts',(-92.7514083751607,-20.4518994955132,
2.57479123331418));
#30978=CARTESIAN_POINT('Ctrl Pts',(-89.4392013302128,-21.4317376344076,
2.41680806806554));
#30979=CARTESIAN_POINT('Ctrl Pts',(-88.4497278964895,-24.7410889661721,
2.25882490281691));
#30980=CARTESIAN_POINT('Ctrl Pts',(-90.6804687378896,-27.3782236865054,
2.10084173756828));
#30981=CARTESIAN_POINT('Ctrl Pts',(-94.1080770316232,-26.9512424666579,
1.94285857231964));
#30982=CARTESIAN_POINT('Ctrl Pts',(-95.6235720657977,-23.8472850535338,
1.78487540707101));
#30983=CARTESIAN_POINT('Ctrl Pts',(-93.8523950876059,-20.8820465732966,
1.62689224182237));
#30984=CARTESIAN_POINT('Ctrl Pts',(-90.400968139612,-20.7444872144857,1.46890907657374));
#30985=CARTESIAN_POINT('Ctrl Pts',(-88.4000491745082,-23.5606286501727,
1.31092591132511));
#30986=CARTESIAN_POINT('Ctrl Pts',(-89.6641399192572,-26.7735797938367,
1.15294274607647));
#30987=CARTESIAN_POINT('Ctrl Pts',(-93.0474773599211,-27.4743145446721,
0.994959580827837));
#30988=CARTESIAN_POINT('Ctrl Pts',(-95.4795883375448,-25.0164840574889,
0.8369764155792));
#30989=CARTESIAN_POINT('Ctrl Pts',(-94.9969281342143,-22.7756529106095,
0.731654305413444));
#30990=CARTESIAN_POINT('Ctrl Pts',(-94.3360626576961,-22.0026984430693,
0.678993250330566));
#30991=CARTESIAN_POINT('Ctrl Pts',(-92.7459328543469,-26.7901775698421,
10.1070022498898));
#30992=CARTESIAN_POINT('Ctrl Pts',(-93.6691444859934,-26.5433639279422,
10.0543411948069));
#30993=CARTESIAN_POINT('Ctrl Pts',(-95.2356809967647,-25.0649585003793,
9.94901908464118));
#30994=CARTESIAN_POINT('Ctrl Pts',(-94.6605001017588,-21.8670184595954,
9.79103591939254));
#30995=CARTESIAN_POINT('Ctrl Pts',(-91.667425165607,-20.6087739832983,9.63305275414391));
#30996=CARTESIAN_POINT('Ctrl Pts',(-88.9782976482681,-22.4240535257463,
9.47506958889527));
#30997=CARTESIAN_POINT('Ctrl Pts',(-89.0288364004571,-25.6699555487328,
9.31708642364664));
#30998=CARTESIAN_POINT('Ctrl Pts',(-91.774870685752,-27.4005707111119,9.159103258398));
#30999=CARTESIAN_POINT('Ctrl Pts',(-94.7248362715076,-26.0470362185693,
9.00112009314937));
#31000=CARTESIAN_POINT('Ctrl Pts',(-95.2034139025824,-22.8366309293727,
8.84313692790074));
#31001=CARTESIAN_POINT('Ctrl Pts',(-92.7763213754197,-20.6815091908568,
8.6851537626521));
#31002=CARTESIAN_POINT('Ctrl Pts',(-89.6451103995963,-21.5363385422618,
8.52717059740347));
#31003=CARTESIAN_POINT('Ctrl Pts',(-88.6498492277809,-24.625809250555,8.36918743215482));
#31004=CARTESIAN_POINT('Ctrl Pts',(-90.6932967144891,-27.147641615416,8.21120426690621));
#31005=CARTESIAN_POINT('Ctrl Pts',(-93.9219649800314,-26.8144595128955,
8.05322110165755));
#31006=CARTESIAN_POINT('Ctrl Pts',(-95.4073472203493,-23.9284646524673,
7.89523793640893));
#31007=CARTESIAN_POINT('Ctrl Pts',(-93.8021483443254,-21.1073557321132,
7.73725477116029));
#31008=CARTESIAN_POINT('Ctrl Pts',(-90.5623398433152,-20.9099734355125,
7.57927160591166));
#31009=CARTESIAN_POINT('Ctrl Pts',(-88.6265379620975,-23.5153509270513,
7.42128844066302));
#31010=CARTESIAN_POINT('Ctrl Pts',(-89.7505813969129,-26.5603215597406,
7.26330527541439));
#31011=CARTESIAN_POINT('Ctrl Pts',(-92.9149242312055,-27.2829932024021,
7.10532211016575));
#31012=CARTESIAN_POINT('Ctrl Pts',(-95.2493995844411,-25.0278779284887,
6.94733894491713));
#31013=CARTESIAN_POINT('Ctrl Pts',(-94.6365585933884,-21.8404423026853,
6.78935577966848));
#31014=CARTESIAN_POINT('Ctrl Pts',(-91.6322689727223,-20.6117992123508,
6.63137261441986));
#31015=CARTESIAN_POINT('Ctrl Pts',(-88.9615239423142,-22.4563698860691,
6.47338944917121));
#31016=CARTESIAN_POINT('Ctrl Pts',(-89.0467804073635,-25.7010657590101,
6.31540628392258));
#31017=CARTESIAN_POINT('Ctrl Pts',(-91.8107078419469,-27.4028369282513,
6.15742311867395));
#31018=CARTESIAN_POINT('Ctrl Pts',(-94.7463297251755,-26.0181188570852,
5.99943995342532));
#31019=CARTESIAN_POINT('Ctrl Pts',(-95.190936809381,-22.8028980999998,5.84145678817668));
#31020=CARTESIAN_POINT('Ctrl Pts',(-92.7412552940464,-20.6734896257781,
5.68347362292805));
#31021=CARTESIAN_POINT('Ctrl Pts',(-89.6192299263401,-21.561339601955,5.52549045767941));
#31022=CARTESIAN_POINT('Ctrl Pts',(-88.6566442762471,-24.661137795831,5.36750729243077));
#31023=CARTESIAN_POINT('Ctrl Pts',(-90.7265963834906,-27.1612614428767,
5.20952412718214));
#31024=CARTESIAN_POINT('Ctrl Pts',(-93.951569034899,-26.7940130605404,5.05154096193351));
#31025=CARTESIAN_POINT('Ctrl Pts',(-95.4064019604354,-23.8924994667599,
4.89355779668487));
#31026=CARTESIAN_POINT('Ctrl Pts',(-93.7715120400194,-21.0884925256084,
4.73557463143624));
#31027=CARTESIAN_POINT('Ctrl Pts',(-90.5298002338789,-20.9253222402166,
4.5775914661876));
#31028=CARTESIAN_POINT('Ctrl Pts',(-88.6216097965222,-23.5509896272809,
4.41960830093897));
#31029=CARTESIAN_POINT('Ctrl Pts',(-89.7777345857426,-26.5839247501514,
4.26162513569034));
#31030=CARTESIAN_POINT('Ctrl Pts',(-92.9495299557167,-27.2731519255296,
4.1036419704417));
#31031=CARTESIAN_POINT('Ctrl Pts',(-95.2600692477113,-24.9935185933677,
3.94565880519306));
#31032=CARTESIAN_POINT('Ctrl Pts',(-94.6136144561259,-21.8127299685234,
3.78767563994443));
#31033=CARTESIAN_POINT('Ctrl Pts',(-91.5965221501949,-20.6158699543453,
3.6296924746958));
#31034=CARTESIAN_POINT('Ctrl Pts',(-88.9453980141133,-22.4885313258635,
3.47170930944716));
#31035=CARTESIAN_POINT('Ctrl Pts',(-89.0649021628072,-25.7321465242476,
3.31372614419853));
#31036=CARTESIAN_POINT('Ctrl Pts',(-91.8466401830968,-27.4046453974022,
3.1557429789499));
#31037=CARTESIAN_POINT('Ctrl Pts',(-94.7674808896859,-25.9890153119553,
2.99775981370126));
#31038=CARTESIAN_POINT('Ctrl Pts',(-95.1781217693893,-22.7692791733585,
2.83977664845263));
#31039=CARTESIAN_POINT('Ctrl Pts',(-92.7060981363895,-20.6658514374356,
2.68179348320399));
#31040=CARTESIAN_POINT('Ctrl Pts',(-89.5936185592569,-21.5866049274252,
2.52381031795536));
#31041=CARTESIAN_POINT('Ctrl Pts',(-88.6638107867397,-24.6964009920718,
2.36582715270672));
#31042=CARTESIAN_POINT('Ctrl Pts',(-90.7600370239624,-27.1745153876391,
2.20784398745809));
#31043=CARTESIAN_POINT('Ctrl Pts',(-93.9809591063932,-26.7732813136335,
2.04986082220945));
#31044=CARTESIAN_POINT('Ctrl Pts',(-95.4050691572154,-23.8564938285714,
1.89187765696082));
#31045=CARTESIAN_POINT('Ctrl Pts',(-93.7406948903597,-21.0700604668217,
1.73389449171218));
#31046=CARTESIAN_POINT('Ctrl Pts',(-90.4973904284657,-20.9407959947845,
1.57591132646355));
#31047=CARTESIAN_POINT('Ctrl Pts',(-88.6171277124372,-23.5871229260259,
1.41792816121492));
#31048=CARTESIAN_POINT('Ctrl Pts',(-89.8049932574594,-26.6063317741661,
1.25994499596628));
#31049=CARTESIAN_POINT('Ctrl Pts',(-92.9843140377459,-27.2648119269358,
1.10196183071765));
#31050=CARTESIAN_POINT('Ctrl Pts',(-95.2697677078962,-24.9551896443915,
0.943978665469012));
#31051=CARTESIAN_POINT('Ctrl Pts',(-94.8162121163602,-22.8494815513233,
0.838656555303255));
#31052=CARTESIAN_POINT('Ctrl Pts',(-94.1951971040191,-22.1231365609212,
0.785995500220377));
#31053=CARTESIAN_POINT('Ctrl Pts',(-92.698066426161,-26.6111321859386,10.2140044997796));
#31054=CARTESIAN_POINT('Ctrl Pts',(-93.5620356702265,-26.3801565479507,
10.1613434446967));
#31055=CARTESIAN_POINT('Ctrl Pts',(-95.028047707573,-24.9966202320186,10.056021334531));
#31056=CARTESIAN_POINT('Ctrl Pts',(-94.4897761065395,-22.0038916474845,
9.89803816928235));
#31057=CARTESIAN_POINT('Ctrl Pts',(-91.6887664556897,-20.8263885790956,
9.74005500403372));
#31058=CARTESIAN_POINT('Ctrl Pts',(-89.1721999516398,-22.5251818354798,
9.58207183878508));
#31059=CARTESIAN_POINT('Ctrl Pts',(-89.2194956377292,-25.5627946871602,
9.42408867353645));
#31060=CARTESIAN_POINT('Ctrl Pts',(-91.7893172087739,-27.182356467315,9.26610550828781));
#31061=CARTESIAN_POINT('Ctrl Pts',(-94.5499838314406,-25.9156781324103,
9.10812234303918));
#31062=CARTESIAN_POINT('Ctrl Pts',(-94.9978511892309,-22.9112841930658,
8.95013917779054));
#31063=CARTESIAN_POINT('Ctrl Pts',(-92.7265049192209,-20.8944563764859,
8.79215601254192));
#31064=CARTESIAN_POINT('Ctrl Pts',(-89.7962234029809,-21.694431423617,8.63417284729327));
#31065=CARTESIAN_POINT('Ctrl Pts',(-88.8648280297145,-24.5856511406457,
8.47618968204465));
#31066=CARTESIAN_POINT('Ctrl Pts',(-90.7771477187876,-26.9456578035202,
8.318206516796));
#31067=CARTESIAN_POINT('Ctrl Pts',(-93.7986327013197,-26.6338559594106,
8.16022335154738));
#31068=CARTESIAN_POINT('Ctrl Pts',(-95.1886981287094,-23.9330550677513,
8.00224018629873));
#31069=CARTESIAN_POINT('Ctrl Pts',(-93.6865046857825,-21.2929763926182,
7.84425702105011));
#31070=CARTESIAN_POINT('Ctrl Pts',(-90.6545943354517,-21.108260096007,7.68627385580146));
#31071=CARTESIAN_POINT('Ctrl Pts',(-88.8430126453538,-23.5464508040852,
7.52829069055284));
#31072=CARTESIAN_POINT('Ctrl Pts',(-89.8949263381463,-26.3960260104052,
7.3703075253042));
#31073=CARTESIAN_POINT('Ctrl Pts',(-92.8562136451878,-27.0723238942441,
7.21232436005557));
#31074=CARTESIAN_POINT('Ctrl Pts',(-95.0408859750062,-24.9619191162964,
7.05434119480693));
#31075=CARTESIAN_POINT('Ctrl Pts',(-94.4673709220947,-21.9790208796034,
6.8963580295583));
#31076=CARTESIAN_POINT('Ctrl Pts',(-91.6558662317871,-20.8292196795368,
6.73837486430966));
#31077=CARTESIAN_POINT('Ctrl Pts',(-89.1565026125286,-22.5554244585598,
6.58039169906103));
#31078=CARTESIAN_POINT('Ctrl Pts',(-89.2362881797111,-25.5919085587089,
6.42240853381239));
#31079=CARTESIAN_POINT('Ctrl Pts',(-91.822854698647,-27.184477261553,6.26442536856376));
#31080=CARTESIAN_POINT('Ctrl Pts',(-94.5700980525807,-25.8886163947921,
6.10644220331513));
#31081=CARTESIAN_POINT('Ctrl Pts',(-94.9861747497105,-22.8797159955968,
5.94845903806648));
#31082=CARTESIAN_POINT('Ctrl Pts',(-92.6936890243839,-20.8869514260051,
5.79047587281786));
#31083=CARTESIAN_POINT('Ctrl Pts',(-89.7720036768111,-21.7178281680942,
5.63249270756922));
#31084=CARTESIAN_POINT('Ctrl Pts',(-88.8711870406774,-24.6187126571061,
5.47450954232059));
#31085=CARTESIAN_POINT('Ctrl Pts',(-90.808310551738,-26.9584036481696,5.31652637707195));
#31086=CARTESIAN_POINT('Ctrl Pts',(-93.8263370672836,-26.614721553626,5.15854321182333));
#31087=CARTESIAN_POINT('Ctrl Pts',(-95.1878135260188,-23.8993977640051,
5.00056004657468));
#31088=CARTESIAN_POINT('Ctrl Pts',(-93.6578343097117,-21.2753236359739,
4.84257688132605));
#31089=CARTESIAN_POINT('Ctrl Pts',(-90.6241427891289,-21.1226239696228,
4.68459371607742));
#31090=CARTESIAN_POINT('Ctrl Pts',(-88.8384007196145,-23.5798025728902,
4.52661055082878));
#31091=CARTESIAN_POINT('Ctrl Pts',(-89.9203371098729,-26.4181145867162,
4.36862738558015));
#31092=CARTESIAN_POINT('Ctrl Pts',(-92.8885987242112,-27.0631141310124,
4.21064422033151));
#31093=CARTESIAN_POINT('Ctrl Pts',(-95.0508709671726,-24.9297646158834,
4.05266105508288));
#31094=CARTESIAN_POINT('Ctrl Pts',(-94.445899107565,-21.9530868428383,3.89467788983425));
#31095=CARTESIAN_POINT('Ctrl Pts',(-91.62241327888,-20.8330292024708,3.7366947245856));
#31096=CARTESIAN_POINT('Ctrl Pts',(-89.1414114833444,-22.5855221023445,
3.57871155933698));
#31097=CARTESIAN_POINT('Ctrl Pts',(-89.2532470641262,-25.6209948747027,
3.42072839408834));
#31098=CARTESIAN_POINT('Ctrl Pts',(-91.8564812654672,-27.1861696814399,
3.26274522883971));
#31099=CARTESIAN_POINT('Ctrl Pts',(-94.58989194922,-25.8613804209117,3.10476206359107));
#31100=CARTESIAN_POINT('Ctrl Pts',(-94.9741820494077,-22.8482543917338,
2.94677889834244));
#31101=CARTESIAN_POINT('Ctrl Pts',(-92.6607878976182,-20.8798033793579,
2.7887957330938));
#31102=CARTESIAN_POINT('Ctrl Pts',(-89.7480357883012,-21.7414722204429,
2.63081256784517));
#31103=CARTESIAN_POINT('Ctrl Pts',(-88.8778936769897,-24.6517130179715,
2.47282940259654));
#31104=CARTESIAN_POINT('Ctrl Pts',(-90.8396053100351,-26.9708070887728,
2.3148462373479));
#31105=CARTESIAN_POINT('Ctrl Pts',(-93.8538411811633,-26.595320160609,2.15686307209927));
#31106=CARTESIAN_POINT('Ctrl Pts',(-95.186566248633,-23.8657026036092,1.99887990685063));
#31107=CARTESIAN_POINT('Ctrl Pts',(-93.6289946931135,-21.2580743603466,
1.840896741602));
#31108=CARTESIAN_POINT('Ctrl Pts',(-90.5938127173193,-21.1371047750834,
1.68291357635336));
#31109=CARTESIAN_POINT('Ctrl Pts',(-88.8342062503661,-23.6136172018791,
1.52493041110473));
#31110=CARTESIAN_POINT('Ctrl Pts',(-89.9458465956615,-26.4390837544954,
1.36694724585609));
#31111=CARTESIAN_POINT('Ctrl Pts',(-92.9211507155708,-27.0553093091995,
1.20896408060746));
#31112=CARTESIAN_POINT('Ctrl Pts',(-95.0599470782476,-24.8938952312942,
1.05098091535882));
#31113=CARTESIAN_POINT('Ctrl Pts',(-94.6354960985062,-22.923310192037,0.945658805193066));
#31114=CARTESIAN_POINT('Ctrl Pts',(-94.054331550342,-22.2435746787731,0.892997750110188));
#31115=CARTESIAN_POINT('Ctrl Pts',(-92.6501999979751,-26.4320868020351,
10.3210067496694));
#31116=CARTESIAN_POINT('Ctrl Pts',(-93.4549268544596,-26.2169491679593,
10.2683456945866));
#31117=CARTESIAN_POINT('Ctrl Pts',(-94.8204144183814,-24.928281963658,10.1630235844208));
#31118=CARTESIAN_POINT('Ctrl Pts',(-94.3190521113201,-22.1407648353735,
10.0050404191722));
#31119=CARTESIAN_POINT('Ctrl Pts',(-91.7101077457726,-21.044003174893,9.84705725392354));
#31120=CARTESIAN_POINT('Ctrl Pts',(-89.3661022550113,-22.6263101452131,
9.68907408867489));
#31121=CARTESIAN_POINT('Ctrl Pts',(-89.4101548750016,-25.4556338255876,
9.53109092342626));
#31122=CARTESIAN_POINT('Ctrl Pts',(-91.8037637317956,-26.9641422235181,
9.37310775817763));
#31123=CARTESIAN_POINT('Ctrl Pts',(-94.3751313913739,-25.7843200462513,
9.21512459292899));
#31124=CARTESIAN_POINT('Ctrl Pts',(-94.7922884758791,-22.9859374567589,
9.05714142768036));
#31125=CARTESIAN_POINT('Ctrl Pts',(-92.6766884630223,-21.107403562115,8.89915826243172));
#31126=CARTESIAN_POINT('Ctrl Pts',(-89.9473364063652,-21.8525243049723,
8.7411750971831));
#31127=CARTESIAN_POINT('Ctrl Pts',(-89.0798068316481,-24.5454930307365,
8.58319193193445));
#31128=CARTESIAN_POINT('Ctrl Pts',(-90.8609987230861,-26.7436739916243,
8.42520876668582));
#31129=CARTESIAN_POINT('Ctrl Pts',(-93.675300422608,-26.4532524059257,8.26722560143718));
#31130=CARTESIAN_POINT('Ctrl Pts',(-94.9700490370695,-23.9376454830353,
8.10924243618854));
#31131=CARTESIAN_POINT('Ctrl Pts',(-93.5708610272395,-21.4785970531231,
7.95125927093992));
#31132=CARTESIAN_POINT('Ctrl Pts',(-90.7468488275882,-21.3065467565016,
7.79327610569128));
#31133=CARTESIAN_POINT('Ctrl Pts',(-89.05948732861,-23.577550681119,7.63529294044265));
#31134=CARTESIAN_POINT('Ctrl Pts',(-90.0392712793796,-26.2317304610699,
7.47730977519401));
#31135=CARTESIAN_POINT('Ctrl Pts',(-92.7975030591701,-26.861654586086,7.31932660994538));
#31136=CARTESIAN_POINT('Ctrl Pts',(-94.8323723655712,-24.8959603041042,
7.16134344469674));
#31137=CARTESIAN_POINT('Ctrl Pts',(-94.298183250801,-22.1175994565215,7.00336027944811));
#31138=CARTESIAN_POINT('Ctrl Pts',(-91.6794634908518,-21.0466401467228,
6.84537711419947));
#31139=CARTESIAN_POINT('Ctrl Pts',(-89.3514812827431,-22.6544790310505,
6.68739394895084));
#31140=CARTESIAN_POINT('Ctrl Pts',(-89.4257959520587,-25.4827513584077,
6.52941078370221));
#31141=CARTESIAN_POINT('Ctrl Pts',(-91.8350015553469,-26.9661175948547,
6.37142761845357));
#31142=CARTESIAN_POINT('Ctrl Pts',(-94.393866379986,-25.7591139324989,6.21344445320494));
#31143=CARTESIAN_POINT('Ctrl Pts',(-94.7814126900398,-22.9565338911938,
6.0554612879563));
#31144=CARTESIAN_POINT('Ctrl Pts',(-92.6461227547216,-21.1004132262322,
5.89747812270767));
#31145=CARTESIAN_POINT('Ctrl Pts',(-89.9247774272819,-21.8743167342334,
5.73949495745903));
#31146=CARTESIAN_POINT('Ctrl Pts',(-89.0857298051077,-24.5762875183812,
5.5815117922104));
#31147=CARTESIAN_POINT('Ctrl Pts',(-90.8900247199854,-26.7555458534626,
5.42352862696176));
#31148=CARTESIAN_POINT('Ctrl Pts',(-93.7011050996681,-26.4354300467115,
5.26554546171314));
#31149=CARTESIAN_POINT('Ctrl Pts',(-94.9692250916023,-23.9062960612504,
5.10756229646449));
#31150=CARTESIAN_POINT('Ctrl Pts',(-93.5441565794039,-21.4621547463393,
4.94957913121586));
#31151=CARTESIAN_POINT('Ctrl Pts',(-90.718485344379,-21.3199256990289,4.79159596596723));
#31152=CARTESIAN_POINT('Ctrl Pts',(-89.0551916427067,-23.6086155184995,
4.63361280071859));
#31153=CARTESIAN_POINT('Ctrl Pts',(-90.0629396340034,-26.252304423281,4.47562963546996));
#31154=CARTESIAN_POINT('Ctrl Pts',(-92.8276674927058,-26.8530763364952,
4.31764647022132));
#31155=CARTESIAN_POINT('Ctrl Pts',(-94.841672686634,-24.8660106383991,4.15966330497269));
#31156=CARTESIAN_POINT('Ctrl Pts',(-94.278183759004,-22.0934437171531,4.00168013972405));
#31157=CARTESIAN_POINT('Ctrl Pts',(-91.648304407565,-21.0501884505964,3.84369697447542));
#31158=CARTESIAN_POINT('Ctrl Pts',(-89.3374249525755,-22.6825128788256,
3.68571380922679));
#31159=CARTESIAN_POINT('Ctrl Pts',(-89.4415919654453,-25.5098432251578,
3.52773064397815));
#31160=CARTESIAN_POINT('Ctrl Pts',(-91.8663223478376,-26.9676939654775,
3.36974747872951));
#31161=CARTESIAN_POINT('Ctrl Pts',(-94.4123030087544,-25.7337455298681,
3.21176431348088));
#31162=CARTESIAN_POINT('Ctrl Pts',(-94.770242329426,-22.9272296101091,3.05378114823225));
#31163=CARTESIAN_POINT('Ctrl Pts',(-92.6154776588472,-21.0937553212802,
2.89579798298361));
#31164=CARTESIAN_POINT('Ctrl Pts',(-89.9024530173452,-21.8963395134606,
2.73781481773498));
#31165=CARTESIAN_POINT('Ctrl Pts',(-89.0919765672402,-24.6070250438712,
2.57983165248634));
#31166=CARTESIAN_POINT('Ctrl Pts',(-90.9191735961077,-26.7670987899064,
2.42184848723771));
#31167=CARTESIAN_POINT('Ctrl Pts',(-93.7267232559334,-26.4173590075846,
2.26386532198908));
#31168=CARTESIAN_POINT('Ctrl Pts',(-94.9680633400506,-23.8749113786469,
2.10588215674044));
#31169=CARTESIAN_POINT('Ctrl Pts',(-93.5172944958673,-21.4460882538716,
1.94789899149181));
#31170=CARTESIAN_POINT('Ctrl Pts',(-90.6902350061731,-21.3334135553823,
1.78991582624317));
#31171=CARTESIAN_POINT('Ctrl Pts',(-89.051284788295,-23.6401114777322,1.63193266099454));
#31172=CARTESIAN_POINT('Ctrl Pts',(-90.0866999338637,-26.2718357348248,
1.4739494957459));
#31173=CARTESIAN_POINT('Ctrl Pts',(-92.8579873933955,-26.8458066914632,
1.31596633049727));
#31174=CARTESIAN_POINT('Ctrl Pts',(-94.8501264485991,-24.8326008181969,
1.15798316524863));
#31175=CARTESIAN_POINT('Ctrl Pts',(-94.4547800806522,-22.9971388327508,
1.05266105508288));
#31176=CARTESIAN_POINT('Ctrl Pts',(-93.913465996665,-22.364012796625,0.999999999999999));
#31177=CARTESIAN_POINT('Ctrl Pts',(-94.5149492652116,-23.9982505980887,
9.11258330249199));
#31178=CARTESIAN_POINT('Ctrl Pts',(-94.5168562980303,-23.7052247424895,
9.09410267755478));
#31179=CARTESIAN_POINT('Ctrl Pts',(-94.4695028989504,-23.4127947803891,
9.07562205261757));
#31180=CARTESIAN_POINT('Ctrl Pts',(-94.3701622929854,-23.139245572567,9.05714142768036));
#31181=CARTESIAN_POINT('Ctrl Pts',(-94.0870884715935,-22.3597594918776,
9.00448037259748));
#31182=CARTESIAN_POINT('Ctrl Pts',(-93.3818884673079,-21.7335815269963,
8.9518193175146));
#31183=CARTESIAN_POINT('Ctrl Pts',(-92.5743964557222,-21.5446793350319,
8.89915826243172));
#31184=CARTESIAN_POINT('Ctrl Pts',(-91.7669044441366,-21.3557771430674,
8.84649720734885));
#31185=CARTESIAN_POINT('Ctrl Pts',(-90.8571204252509,-21.6041507240199,
8.79383615226597));
#31186=CARTESIAN_POINT('Ctrl Pts',(-90.2576401533552,-22.1771656354568,
8.74117509718309));
#31187=CARTESIAN_POINT('Ctrl Pts',(-89.6581598814595,-22.7501805468937,
8.68851404210021));
#31188=CARTESIAN_POINT('Ctrl Pts',(-89.3689833565538,-23.6478367888151,
8.63585298701733));
#31189=CARTESIAN_POINT('Ctrl Pts',(-89.5212604093406,-24.4630284032571,
8.58319193193445));
#31190=CARTESIAN_POINT('Ctrl Pts',(-89.6735374621274,-25.2782200176991,
8.53053087685158));
#31191=CARTESIAN_POINT('Ctrl Pts',(-90.2672680926067,-26.0109470046617,
8.4778698217687));
#31192=CARTESIAN_POINT('Ctrl Pts',(-91.0331836911001,-26.3289069005266,
8.42520876668582));
#31193=CARTESIAN_POINT('Ctrl Pts',(-91.7990992895934,-26.6468667963914,
8.37254771160294));
#31194=CARTESIAN_POINT('Ctrl Pts',(-92.7371998561007,-26.5500596011586,
8.31988665652006));
#31195=CARTESIAN_POINT('Ctrl Pts',(-93.422041575098,-26.0823881830604,8.26722560143718));
#31196=CARTESIAN_POINT('Ctrl Pts',(-94.0924009622684,-25.6246066015112,
8.21567816845545));
#31197=CARTESIAN_POINT('Ctrl Pts',(-94.5200995637937,-24.811480262719,8.16413073547371));
#31198=CARTESIAN_POINT('Ctrl Pts',(-94.5215633824187,-23.9996804087645,
8.11258330249198));
#31199=CARTESIAN_POINT('Ctrl Pts',(-92.7937992825329,-26.9692229537457,
10.));
#31200=CARTESIAN_POINT('Ctrl Pts',(-92.886852386908,-26.9351837124997,10.));
#31201=CARTESIAN_POINT('Ctrl Pts',(-92.9778402151635,-26.8963761434536,
10.));
#31202=CARTESIAN_POINT('Ctrl Pts',(-93.0665542695815,-26.8531284786668,
10.));
#31203=CARTESIAN_POINT('Ctrl Pts',(-93.1572340298667,-26.8089225419468,
10.));
#31204=CARTESIAN_POINT('Ctrl Pts',(-93.2455388043682,-26.7600769477925,
10.));
#31205=CARTESIAN_POINT('Ctrl Pts',(-93.3312170072855,-26.7068966945046,
10.));
#31206=CARTESIAN_POINT('Ctrl Pts',(-93.4136695050849,-26.65571862858,10.));
#31207=CARTESIAN_POINT('Ctrl Pts',(-93.4936897697168,-26.6005252759063,
10.));
#31208=CARTESIAN_POINT('Ctrl Pts',(-93.5710205780919,-26.5415583960894,
10.));
#31209=CARTESIAN_POINT('Ctrl Pts',(-93.63868503542,-26.4899623762497,10.));
#31210=CARTESIAN_POINT('Ctrl Pts',(-93.7042900873145,-26.4354765516642,
10.));
#31211=CARTESIAN_POINT('Ctrl Pts',(-93.7676387673489,-26.378250171364,10.));
#31212=CARTESIAN_POINT('Ctrl Pts',(-93.781737609333,-26.3655139045193,10.));
#31213=CARTESIAN_POINT('Ctrl Pts',(-93.795727291904,-26.3526391912679,10.));
#31214=CARTESIAN_POINT('Ctrl Pts',(-93.8095861705268,-26.3396461050457,
10.));
#31215=CARTESIAN_POINT('Ctrl Pts',(-93.882016875094,-26.271740294252,10.));
#31216=CARTESIAN_POINT('Ctrl Pts',(-93.9509819060163,-26.2005127260756,
10.));
#31217=CARTESIAN_POINT('Ctrl Pts',(-94.0162413172811,-26.1262540066759,
10.));
#31218=CARTESIAN_POINT('Ctrl Pts',(-94.0811410662549,-26.0524045471918,
10.));
#31219=CARTESIAN_POINT('Ctrl Pts',(-94.1423764147232,-25.9755564586413,
10.));
#31220=CARTESIAN_POINT('Ctrl Pts',(-94.1996677535172,-25.895968801161,10.));
#31221=CARTESIAN_POINT('Ctrl Pts',(-94.2548605589228,-25.8192963724053,
10.));
#31222=CARTESIAN_POINT('Ctrl Pts',(-94.3063931619475,-25.7400806580935,
10.));
#31223=CARTESIAN_POINT('Ctrl Pts',(-94.3539706372945,-25.6585396692548,
10.));
#31224=CARTESIAN_POINT('Ctrl Pts',(-94.3739594034168,-25.6242817826521,
10.));
#31225=CARTESIAN_POINT('Ctrl Pts',(-94.3932494780977,-25.589613354766,10.));
#31226=CARTESIAN_POINT('Ctrl Pts',(-94.4118163867649,-25.554550253182,10.));
#31227=CARTESIAN_POINT('Ctrl Pts',(-94.424852971342,-25.5299310180939,10.));
#31228=CARTESIAN_POINT('Ctrl Pts',(-94.4375330011157,-25.5051172053715,
10.));
#31229=CARTESIAN_POINT('Ctrl Pts',(-94.4498475176035,-25.4801143018019,
10.));
#31230=CARTESIAN_POINT('Ctrl Pts',(-94.4575999796004,-25.4643740118823,
10.));
#31231=CARTESIAN_POINT('Ctrl Pts',(-94.4652084584732,-25.4485566580947,
10.));
#31232=CARTESIAN_POINT('Ctrl Pts',(-94.4726610535095,-25.4326847360384,
10.));
#31233=CARTESIAN_POINT('Ctrl Pts',(-94.5147816016199,-25.3429798676917,
10.));
#31234=CARTESIAN_POINT('Ctrl Pts',(-94.551999940776,-25.2513903180325,10.));
#31235=CARTESIAN_POINT('Ctrl Pts',(-94.5840244250316,-25.1581885555992,
10.));
#31236=CARTESIAN_POINT('Ctrl Pts',(-94.6138868935619,-25.0712789686901,
10.));
#31237=CARTESIAN_POINT('Ctrl Pts',(-94.6392329460682,-24.9829667140799,
10.));
#31238=CARTESIAN_POINT('Ctrl Pts',(-94.6597755596864,-24.8934640331103,
10.));
#31239=CARTESIAN_POINT('Ctrl Pts',(-94.6612628263414,-24.8869841199203,
10.));
#31240=CARTESIAN_POINT('Ctrl Pts',(-94.6627248923899,-24.8804979657906,
10.));
#31241=CARTESIAN_POINT('Ctrl Pts',(-94.6641616381052,-24.874005650947,10.));
#31242=CARTESIAN_POINT('Ctrl Pts',(-94.6847472407902,-24.7809841702089,
10.));
#31243=CARTESIAN_POINT('Ctrl Pts',(-94.7001390631694,-24.6866969715819,
10.));
#31244=CARTESIAN_POINT('Ctrl Pts',(-94.7104141120184,-24.5915520773872,
10.));
#31245=CARTESIAN_POINT('Ctrl Pts',(-94.7162317525601,-24.5376818912762,
10.));
#31246=CARTESIAN_POINT('Ctrl Pts',(-94.7204081622463,-24.483536940679,10.));
#31247=CARTESIAN_POINT('Ctrl Pts',(-94.7229504259482,-24.4291939795176,
10.));
#31248=CARTESIAN_POINT('Ctrl Pts',(-94.7235977676587,-24.4153565222132,
10.));
#31249=CARTESIAN_POINT('Ctrl Pts',(-94.7241390041218,-24.4015076323046,
10.));
#31250=CARTESIAN_POINT('Ctrl Pts',(-94.7245740715257,-24.3876608123636,
10.));
#31251=CARTESIAN_POINT('Ctrl Pts',(-94.7275028913787,-24.2944457363059,
10.));
#31252=CARTESIAN_POINT('Ctrl Pts',(-94.7256323237335,-24.20117339609,10.));
#31253=CARTESIAN_POINT('Ctrl Pts',(-94.7190972361895,-24.1082190601576,
10.));
#31254=CARTESIAN_POINT('Ctrl Pts',(-94.7125517108725,-24.0151162585377,
10.));
#31255=CARTESIAN_POINT('Ctrl Pts',(-94.7013263747111,-23.922331498206,10.));
#31256=CARTESIAN_POINT('Ctrl Pts',(-94.6855058357614,-23.8302540027448,
10.));
#31257=CARTESIAN_POINT('Ctrl Pts',(-94.669912459968,-23.7394986249788,10.));
#31258=CARTESIAN_POINT('Ctrl Pts',(-94.6498544351971,-23.6494295034801,
10.));
#31259=CARTESIAN_POINT('Ctrl Pts',(-94.6253697912028,-23.5604445846,10.));
#31260=CARTESIAN_POINT('Ctrl Pts',(-94.6161277167171,-23.5268559709129,
10.));
#31261=CARTESIAN_POINT('Ctrl Pts',(-94.6062545340008,-23.4934221578844,
10.));
#31262=CARTESIAN_POINT('Ctrl Pts',(-94.5957508646961,-23.4601658754547,
10.));
#31263=CARTESIAN_POINT('Ctrl Pts',(-94.5880548970241,-23.4357992215696,
10.));
#31264=CARTESIAN_POINT('Ctrl Pts',(-94.5800204433778,-23.4115278887989,
10.));
#31265=CARTESIAN_POINT('Ctrl Pts',(-94.5716475012962,-23.3873611140396,
10.));
#31266=CARTESIAN_POINT('Ctrl Pts',(-94.5664800360046,-23.3724462885743,
10.));
#31267=CARTESIAN_POINT('Ctrl Pts',(-94.5611866347534,-23.3575799758845,
10.));
#31268=CARTESIAN_POINT('Ctrl Pts',(-94.5557684843318,-23.3427662650201,
10.));
#31269=CARTESIAN_POINT('Ctrl Pts',(-94.5240624591822,-23.2560791388461,
10.));
#31270=CARTESIAN_POINT('Ctrl Pts',(-94.4880796644939,-23.1711661844698,
10.));
#31271=CARTESIAN_POINT('Ctrl Pts',(-94.447880401404,-23.0884282232178,10.));
#31272=CARTESIAN_POINT('Ctrl Pts',(-94.4177309540866,-23.0263747522788,
10.));
#31273=CARTESIAN_POINT('Ctrl Pts',(-94.3852087541631,-22.9655451998349,
10.));
#31274=CARTESIAN_POINT('Ctrl Pts',(-94.3503241512496,-22.9061236582037,
10.));
#31275=CARTESIAN_POINT('Ctrl Pts',(-94.334545249284,-22.8792462795972,10.));
#31276=CARTESIAN_POINT('Ctrl Pts',(-94.3182828567332,-22.8526571658029,
10.));
#31277=CARTESIAN_POINT('Ctrl Pts',(-94.3015371510007,-22.8263744217796,
10.));
#31278=CARTESIAN_POINT('Ctrl Pts',(-94.2924151854529,-22.8120573013602,
10.));
#31279=CARTESIAN_POINT('Ctrl Pts',(-94.2831549823775,-22.7978392515682,
10.));
#31280=CARTESIAN_POINT('Ctrl Pts',(-94.2737572212008,-22.7837232845595,
10.));
#31281=CARTESIAN_POINT('Ctrl Pts',(-94.2261821463953,-22.7122628405486,
10.));
#31282=CARTESIAN_POINT('Ctrl Pts',(-94.175081861178,-22.6434116537846,10.));
#31283=CARTESIAN_POINT('Ctrl Pts',(-94.1204874224216,-22.5775232108296,
10.));
#31284=CARTESIAN_POINT('Ctrl Pts',(-94.0743569854685,-22.5218497258939,
10.));
#31285=CARTESIAN_POINT('Ctrl Pts',(-94.0257311604217,-22.4682919003745,
10.));
#31286=CARTESIAN_POINT('Ctrl Pts',(-93.9746123907307,-22.41708711057,10.));
#31287=CARTESIAN_POINT('Ctrl Pts',(-93.9557806038367,-22.3982236344852,
10.));
#31288=CARTESIAN_POINT('Ctrl Pts',(-93.9366103467742,-22.3796797449892,
10.));
#31289=CARTESIAN_POINT('Ctrl Pts',(-93.9171117712832,-22.3614597429256,
10.));
#31290=CARTESIAN_POINT('Origin',(-92.,-24.,5.));
#31291=CARTESIAN_POINT('Origin',(-30.,-108.,40.));
#31292=CARTESIAN_POINT('',(-30.,-95.3939201416946,10.));
#31293=CARTESIAN_POINT('',(-30.,-95.3939201416946,40.));
#31294=CARTESIAN_POINT('',(-30.,-95.3939201416946,0.));
#31295=CARTESIAN_POINT('',(-30.,-88.,10.));
#31296=CARTESIAN_POINT('',(-30.,-88.,10.));
#31297=CARTESIAN_POINT('',(-30.,-88.,40.));
#31298=CARTESIAN_POINT('',(-30.,-88.,40.));
#31299=CARTESIAN_POINT('',(-30.,-54.,40.));
#31300=CARTESIAN_POINT('Origin',(-30.,-88.,40.));
#31301=CARTESIAN_POINT('',(-12.,-88.,40.));
#31302=CARTESIAN_POINT('',(-12.,-88.,28.));
#31303=CARTESIAN_POINT('',(-12.,-88.,40.));
#31304=CARTESIAN_POINT('',(-15.,-88.,40.));
#31305=CARTESIAN_POINT('',(30.,-88.,10.));
#31306=CARTESIAN_POINT('',(30.,-88.,10.));
#31307=CARTESIAN_POINT('',(30.,-88.,40.));
#31308=CARTESIAN_POINT('',(30.,-88.,40.));
#31309=CARTESIAN_POINT('',(12.,-88.,40.));
#31310=CARTESIAN_POINT('',(-15.,-88.,40.));
#31311=CARTESIAN_POINT('',(12.,-88.,28.));
#31312=CARTESIAN_POINT('',(12.,-88.,40.));
#31313=CARTESIAN_POINT('',(18.,-88.,28.));
#31314=CARTESIAN_POINT('',(-15.,-88.,28.));
#31315=CARTESIAN_POINT('',(18.,-88.,12.));
#31316=CARTESIAN_POINT('',(18.,-88.,34.));
#31317=CARTESIAN_POINT('',(-18.,-88.,12.));
#31318=CARTESIAN_POINT('',(-15.,-88.,12.));
#31319=CARTESIAN_POINT('',(-18.,-88.,28.));
#31320=CARTESIAN_POINT('',(-18.,-88.,34.));
#31321=CARTESIAN_POINT('',(-15.,-88.,28.));
#31322=CARTESIAN_POINT('Origin',(30.,-88.,40.));
#31323=CARTESIAN_POINT('',(30.,-95.3939201416946,40.));
#31324=CARTESIAN_POINT('',(30.,-95.3939201416946,10.));
#31325=CARTESIAN_POINT('',(30.,-95.3939201416946,0.));
#31326=CARTESIAN_POINT('',(30.,-44.,40.));
#31327=CARTESIAN_POINT('',(30.,-108.,10.));
#31328=CARTESIAN_POINT('Origin',(0.,-98.,10.));
#31329=CARTESIAN_POINT('Origin',(0.,0.,10.));
#31330=CARTESIAN_POINT('Origin',(30.,88.,40.));
#31331=CARTESIAN_POINT('',(12.,88.,40.));
#31332=CARTESIAN_POINT('',(12.,88.,28.));
#31333=CARTESIAN_POINT('',(12.,88.,40.));
#31334=CARTESIAN_POINT('',(30.,88.,40.));
#31335=CARTESIAN_POINT('',(15.,88.,40.));
#31336=CARTESIAN_POINT('',(30.,88.,10.));
#31337=CARTESIAN_POINT('',(30.,88.,40.));
#31338=CARTESIAN_POINT('',(-30.,88.,10.));
#31339=CARTESIAN_POINT('',(-30.,88.,10.));
#31340=CARTESIAN_POINT('',(-30.,88.,40.));
#31341=CARTESIAN_POINT('',(-30.,88.,40.));
#31342=CARTESIAN_POINT('',(-12.,88.,40.));
#31343=CARTESIAN_POINT('',(15.,88.,40.));
#31344=CARTESIAN_POINT('',(-12.,88.,28.));
#31345=CARTESIAN_POINT('',(-12.,88.,40.));
#31346=CARTESIAN_POINT('',(-18.,88.,28.));
#31347=CARTESIAN_POINT('',(15.,88.,28.));
#31348=CARTESIAN_POINT('',(-18.,88.,12.));
#31349=CARTESIAN_POINT('',(-18.,88.,34.));
#31350=CARTESIAN_POINT('',(18.,88.,12.));
#31351=CARTESIAN_POINT('',(15.,88.,12.));
#31352=CARTESIAN_POINT('',(18.,88.,28.));
#31353=CARTESIAN_POINT('',(18.,88.,34.));
#31354=CARTESIAN_POINT('',(15.,88.,28.));
#31355=CARTESIAN_POINT('Origin',(30.,108.,40.));
#31356=CARTESIAN_POINT('',(30.,95.3939201416946,10.));
#31357=CARTESIAN_POINT('',(30.,95.3939201416946,40.));
#31358=CARTESIAN_POINT('',(30.,95.3939201416946,0.));
#31359=CARTESIAN_POINT('',(30.,88.,10.));
#31360=CARTESIAN_POINT('',(30.,54.,40.));
#31361=CARTESIAN_POINT('Origin',(-30.,88.,40.));
#31362=CARTESIAN_POINT('',(-30.,95.3939201416946,40.));
#31363=CARTESIAN_POINT('',(-30.,95.3939201416946,10.));
#31364=CARTESIAN_POINT('',(-30.,95.3939201416946,0.));
#31365=CARTESIAN_POINT('',(-30.,44.,40.));
#31366=CARTESIAN_POINT('',(-30.,108.,10.));
#31367=CARTESIAN_POINT('Origin',(0.,98.,10.));
#31368=CARTESIAN_POINT('Origin',(0.,0.,10.));
#31369=CARTESIAN_POINT('Origin',(0.,-54.,12.));
#31370=CARTESIAN_POINT('',(18.,-18.,12.));
#31371=CARTESIAN_POINT('',(18.,-90.,12.));
#31372=CARTESIAN_POINT('',(8.71779788708135,-18.,12.));
#31373=CARTESIAN_POINT('',(18.,-18.,12.));
#31374=CARTESIAN_POINT('',(-8.71779788708135,-18.,12.));
#31375=CARTESIAN_POINT('Origin',(0.,0.,12.));
#31376=CARTESIAN_POINT('',(-18.,-18.,12.));
#31377=CARTESIAN_POINT('',(18.,-18.,12.));
#31378=CARTESIAN_POINT('',(-18.,-18.,12.));
#31379=CARTESIAN_POINT('Origin',(18.,-18.,28.));
#31380=CARTESIAN_POINT('',(18.,-18.,28.));
#31381=CARTESIAN_POINT('',(18.,-90.,28.));
#31382=CARTESIAN_POINT('',(18.,-18.,28.));
#31383=CARTESIAN_POINT('Origin',(0.,0.,40.));
#31384=CARTESIAN_POINT('',(95.3939201416946,-30.,40.));
#31385=CARTESIAN_POINT('Origin',(0.,0.,40.));
#31386=CARTESIAN_POINT('',(88.,-30.,40.));
#31387=CARTESIAN_POINT('',(54.,-30.,40.));
#31388=CARTESIAN_POINT('',(88.,-12.,40.));
#31389=CARTESIAN_POINT('',(88.,-15.,40.));
#31390=CARTESIAN_POINT('',(18.,-12.,40.));
#31391=CARTESIAN_POINT('',(45.,-12.,40.));
#31392=CARTESIAN_POINT('',(18.,-8.71779788708135,40.));
#31393=CARTESIAN_POINT('',(18.,-6.,40.));
#31394=CARTESIAN_POINT('',(8.71779788708135,-18.,40.));
#31395=CARTESIAN_POINT('Origin',(0.,0.,40.));
#31396=CARTESIAN_POINT('',(12.,-18.,40.));
#31397=CARTESIAN_POINT('',(-6.,-18.,40.));
#31398=CARTESIAN_POINT('',(12.,-9.,40.));
#31399=CARTESIAN_POINT('Origin',(0.,0.,40.));
#31400=CARTESIAN_POINT('',(-12.,-18.,40.));
#31401=CARTESIAN_POINT('',(-12.,-45.,40.));
#31402=CARTESIAN_POINT('',(-8.71779788708135,-18.,40.));
#31403=CARTESIAN_POINT('',(-6.,-18.,40.));
#31404=CARTESIAN_POINT('',(-18.,-8.71779788708135,40.));
#31405=CARTESIAN_POINT('Origin',(0.,0.,40.));
#31406=CARTESIAN_POINT('',(-18.,-12.,40.));
#31407=CARTESIAN_POINT('',(-18.,6.,40.));
#31408=CARTESIAN_POINT('',(-88.,-12.,40.));
#31409=CARTESIAN_POINT('',(-9.,-12.,40.));
#31410=CARTESIAN_POINT('',(-88.,-30.,40.));
#31411=CARTESIAN_POINT('',(-88.,15.,40.));
#31412=CARTESIAN_POINT('',(-95.3939201416946,-30.,40.));
#31413=CARTESIAN_POINT('',(-44.,-30.,40.));
#31414=CARTESIAN_POINT('Origin',(0.,0.,40.));
#31415=CARTESIAN_POINT('Origin',(0.,-54.,28.));
#31416=CARTESIAN_POINT('',(12.,-18.,28.));
#31417=CARTESIAN_POINT('',(12.,-90.,28.));
#31418=CARTESIAN_POINT('',(18.,-18.,28.));
#31419=CARTESIAN_POINT('Origin',(12.,-18.,40.));
#31420=CARTESIAN_POINT('',(12.,-18.,40.));
#31421=CARTESIAN_POINT('Origin',(0.,54.,12.));
#31422=CARTESIAN_POINT('',(-18.,18.,12.));
#31423=CARTESIAN_POINT('',(-18.,90.,12.));
#31424=CARTESIAN_POINT('',(-8.71779788708135,18.,12.));
#31425=CARTESIAN_POINT('',(-18.,18.,12.));
#31426=CARTESIAN_POINT('',(8.71779788708135,18.,12.));
#31427=CARTESIAN_POINT('Origin',(0.,0.,12.));
#31428=CARTESIAN_POINT('',(18.,18.,12.));
#31429=CARTESIAN_POINT('',(-18.,18.,12.));
#31430=CARTESIAN_POINT('',(18.,18.,12.));
#31431=CARTESIAN_POINT('Origin',(-18.,18.,28.));
#31432=CARTESIAN_POINT('',(-18.,18.,28.));
#31433=CARTESIAN_POINT('',(-18.,90.,28.));
#31434=CARTESIAN_POINT('',(-18.,18.,28.));
#31435=CARTESIAN_POINT('Origin',(0.,54.,28.));
#31436=CARTESIAN_POINT('',(-12.,18.,28.));
#31437=CARTESIAN_POINT('',(-12.,90.,28.));
#31438=CARTESIAN_POINT('',(-18.,18.,28.));
#31439=CARTESIAN_POINT('Origin',(-12.,18.,40.));
#31440=CARTESIAN_POINT('',(-12.,18.,40.));
#31441=CARTESIAN_POINT('',(-12.,9.,40.));
#31442=CARTESIAN_POINT('',(-12.,18.,40.));
#31443=CARTESIAN_POINT('Origin',(0.,0.,40.));
#31444=CARTESIAN_POINT('',(-95.3939201416946,30.,40.));
#31445=CARTESIAN_POINT('Origin',(0.,0.,40.));
#31446=CARTESIAN_POINT('',(-88.,30.,40.));
#31447=CARTESIAN_POINT('',(-54.,30.,40.));
#31448=CARTESIAN_POINT('',(-88.,12.,40.));
#31449=CARTESIAN_POINT('',(-88.,15.,40.));
#31450=CARTESIAN_POINT('',(-18.,12.,40.));
#31451=CARTESIAN_POINT('',(-45.,12.,40.));
#31452=CARTESIAN_POINT('',(-18.,8.71779788708135,40.));
#31453=CARTESIAN_POINT('',(-18.,6.,40.));
#31454=CARTESIAN_POINT('',(-8.71779788708135,18.,40.));
#31455=CARTESIAN_POINT('Origin',(0.,0.,40.));
#31456=CARTESIAN_POINT('',(6.,18.,40.));
#31457=CARTESIAN_POINT('Origin',(-18.,-90.,28.));
#31458=CARTESIAN_POINT('',(-18.,-18.,28.));
#31459=CARTESIAN_POINT('',(-18.,-18.,28.));
#31460=CARTESIAN_POINT('',(-18.,-18.,28.));
#31461=CARTESIAN_POINT('Origin',(0.,-54.,28.));
#31462=CARTESIAN_POINT('',(-12.,-18.,28.));
#31463=CARTESIAN_POINT('',(18.,-18.,28.));
#31464=CARTESIAN_POINT('',(-12.,-18.,28.));
#31465=CARTESIAN_POINT('Origin',(0.,54.,28.));
#31466=CARTESIAN_POINT('',(18.,18.,28.));
#31467=CARTESIAN_POINT('',(18.,18.,28.));
#31468=CARTESIAN_POINT('',(12.,18.,28.));
#31469=CARTESIAN_POINT('',(-18.,18.,28.));
#31470=CARTESIAN_POINT('',(12.,18.,28.));
#31471=CARTESIAN_POINT('Origin',(18.,90.,28.));
#31472=CARTESIAN_POINT('',(18.,18.,28.));
#31473=CARTESIAN_POINT('Origin',(0.,0.,0.));
#31474=CARTESIAN_POINT('',(-8.71779788708135,-18.,0.));
#31475=CARTESIAN_POINT('',(8.71779788708135,-18.,0.));
#31476=CARTESIAN_POINT('',(18.,-8.71779788708135,12.));
#31477=CARTESIAN_POINT('',(18.,-8.71779788708135,0.));
#31478=CARTESIAN_POINT('',(18.,8.71779788708135,12.));
#31479=CARTESIAN_POINT('Origin',(0.,0.,12.));
#31480=CARTESIAN_POINT('',(18.,8.71779788708135,40.));
#31481=CARTESIAN_POINT('',(18.,8.71779788708135,0.));
#31482=CARTESIAN_POINT('',(8.71779788708135,18.,40.));
#31483=CARTESIAN_POINT('Origin',(0.,0.,40.));
#31484=CARTESIAN_POINT('',(8.71779788708135,18.,0.));
#31485=CARTESIAN_POINT('',(-8.71779788708135,18.,0.));
#31486=CARTESIAN_POINT('',(-18.,8.71779788708135,12.));
#31487=CARTESIAN_POINT('',(-18.,8.71779788708135,0.));
#31488=CARTESIAN_POINT('',(-20.,-2.44929359829471E-15,12.));
#31489=CARTESIAN_POINT('Origin',(0.,0.,12.));
#31490=CARTESIAN_POINT('',(-20.,2.44929359829471E-15,4.));
#31491=CARTESIAN_POINT('',(-20.,-2.44929359829471E-15,0.));
#31492=CARTESIAN_POINT('Origin',(0.,0.,4.));
#31493=CARTESIAN_POINT('',(-18.,-8.71779788708135,12.));
#31494=CARTESIAN_POINT('Origin',(0.,0.,12.));
#31495=CARTESIAN_POINT('',(-18.,-8.71779788708135,0.));
#31496=CARTESIAN_POINT('Origin',(-12.,-18.,40.));
#31497=CARTESIAN_POINT('',(-12.,-18.,40.));
#31498=CARTESIAN_POINT('',(-18.,-18.,28.));
#31499=CARTESIAN_POINT('Origin',(-12.,-18.,40.));
#31500=CARTESIAN_POINT('',(18.,-18.,28.));
#31501=CARTESIAN_POINT('Origin',(-12.,-90.,40.));
#31502=CARTESIAN_POINT('Origin',(12.,18.,40.));
#31503=CARTESIAN_POINT('',(-18.,18.,28.));
#31504=CARTESIAN_POINT('Origin',(12.,18.,40.));
#31505=CARTESIAN_POINT('',(12.,18.,40.));
#31506=CARTESIAN_POINT('',(6.,18.,40.));
#31507=CARTESIAN_POINT('',(12.,18.,40.));
#31508=CARTESIAN_POINT('',(18.,18.,28.));
#31509=CARTESIAN_POINT('Origin',(12.,90.,40.));
#31510=CARTESIAN_POINT('',(12.,45.,40.));
#31511=CARTESIAN_POINT('Origin',(-88.,-30.,40.));
#31512=CARTESIAN_POINT('',(-95.3939201416946,-30.,10.));
#31513=CARTESIAN_POINT('',(-95.3939201416946,-30.,0.));
#31514=CARTESIAN_POINT('',(-88.,-30.,10.));
#31515=CARTESIAN_POINT('',(-88.,-30.,40.));
#31516=CARTESIAN_POINT('',(-108.,-30.,10.));
#31517=CARTESIAN_POINT('Origin',(-98.,0.,10.));
#31518=CARTESIAN_POINT('',(-100.,-1.22464679914735E-14,10.));
#31519=CARTESIAN_POINT('Origin',(0.,0.,10.));
#31520=CARTESIAN_POINT('',(-88.,30.,10.));
#31521=CARTESIAN_POINT('',(-88.,-30.,10.));
#31522=CARTESIAN_POINT('',(-95.3939201416946,30.,10.));
#31523=CARTESIAN_POINT('',(-88.,30.,10.));
#31524=CARTESIAN_POINT('Origin',(0.,0.,10.));
#31525=CARTESIAN_POINT('Origin',(-88.,30.,40.));
#31526=CARTESIAN_POINT('',(-88.,-12.,28.));
#31527=CARTESIAN_POINT('',(-88.,-12.,40.));
#31528=CARTESIAN_POINT('',(-88.,-18.,28.));
#31529=CARTESIAN_POINT('',(-88.,15.,28.));
#31530=CARTESIAN_POINT('',(-88.,-18.,12.));
#31531=CARTESIAN_POINT('',(-88.,-18.,34.));
#31532=CARTESIAN_POINT('',(-88.,18.,12.));
#31533=CARTESIAN_POINT('',(-88.,15.,12.));
#31534=CARTESIAN_POINT('',(-88.,18.,28.));
#31535=CARTESIAN_POINT('',(-88.,18.,34.));
#31536=CARTESIAN_POINT('',(-88.,12.,28.));
#31537=CARTESIAN_POINT('',(-88.,15.,28.));
#31538=CARTESIAN_POINT('',(-88.,12.,40.));
#31539=CARTESIAN_POINT('',(-88.,30.,40.));
#31540=CARTESIAN_POINT('Origin',(-108.,30.,40.));
#31541=CARTESIAN_POINT('',(-95.3939201416946,30.,0.));
#31542=CARTESIAN_POINT('Origin',(108.,-30.,40.));
#31543=CARTESIAN_POINT('',(95.3939201416946,-30.,10.));
#31544=CARTESIAN_POINT('',(95.3939201416946,-30.,0.));
#31545=CARTESIAN_POINT('',(88.,-30.,10.));
#31546=CARTESIAN_POINT('',(88.,-30.,10.));
#31547=CARTESIAN_POINT('',(88.,-30.,40.));
#31548=CARTESIAN_POINT('Origin',(88.,-30.,40.));
#31549=CARTESIAN_POINT('',(88.,-12.,28.));
#31550=CARTESIAN_POINT('',(88.,-12.,40.));
#31551=CARTESIAN_POINT('',(88.,30.,10.));
#31552=CARTESIAN_POINT('',(88.,30.,10.));
#31553=CARTESIAN_POINT('',(88.,30.,40.));
#31554=CARTESIAN_POINT('',(88.,30.,40.));
#31555=CARTESIAN_POINT('',(88.,12.,40.));
#31556=CARTESIAN_POINT('',(88.,-15.,40.));
#31557=CARTESIAN_POINT('',(88.,12.,28.));
#31558=CARTESIAN_POINT('',(88.,12.,40.));
#31559=CARTESIAN_POINT('',(88.,18.,28.));
#31560=CARTESIAN_POINT('',(88.,-15.,28.));
#31561=CARTESIAN_POINT('',(88.,18.,12.));
#31562=CARTESIAN_POINT('',(88.,18.,34.));
#31563=CARTESIAN_POINT('',(88.,-18.,12.));
#31564=CARTESIAN_POINT('',(88.,-15.,12.));
#31565=CARTESIAN_POINT('',(88.,-18.,28.));
#31566=CARTESIAN_POINT('',(88.,-18.,34.));
#31567=CARTESIAN_POINT('',(88.,-15.,28.));
#31568=CARTESIAN_POINT('Origin',(88.,30.,40.));
#31569=CARTESIAN_POINT('',(95.3939201416946,30.,40.));
#31570=CARTESIAN_POINT('',(95.3939201416946,30.,10.));
#31571=CARTESIAN_POINT('',(95.3939201416946,30.,0.));
#31572=CARTESIAN_POINT('',(44.,30.,40.));
#31573=CARTESIAN_POINT('',(108.,30.,10.));
#31574=CARTESIAN_POINT('Origin',(98.,0.,10.));
#31575=CARTESIAN_POINT('Origin',(0.,0.,10.));
#31576=CARTESIAN_POINT('Origin',(-18.,-18.,28.));
#31577=CARTESIAN_POINT('',(-90.,-18.,28.));
#31578=CARTESIAN_POINT('',(-90.,-18.,12.));
#31579=CARTESIAN_POINT('Origin',(-54.,0.,28.));
#31580=CARTESIAN_POINT('',(-18.,-12.,28.));
#31581=CARTESIAN_POINT('',(-90.,-12.,28.));
#31582=CARTESIAN_POINT('',(-18.,-18.,28.));
#31583=CARTESIAN_POINT('Origin',(-18.,-12.,40.));
#31584=CARTESIAN_POINT('',(-18.,-12.,40.));
#31585=CARTESIAN_POINT('Origin',(0.,0.,0.));
#31586=CARTESIAN_POINT('',(-100.,-1.22464679914735E-14,0.));
#31587=CARTESIAN_POINT('',(-100.,-1.22464679914735E-14,0.));
#31588=CARTESIAN_POINT('Origin',(0.,0.,0.));
#31589=CARTESIAN_POINT('Origin',(0.,0.,40.));
#31590=CARTESIAN_POINT('Origin',(90.,-12.,40.));
#31591=CARTESIAN_POINT('',(18.,-12.,28.));
#31592=CARTESIAN_POINT('',(18.,-12.,28.));
#31593=CARTESIAN_POINT('',(18.,-12.,40.));
#31594=CARTESIAN_POINT('Origin',(54.,0.,28.));
#31595=CARTESIAN_POINT('',(18.,-18.,28.));
#31596=CARTESIAN_POINT('',(18.,18.,28.));
#31597=CARTESIAN_POINT('Origin',(0.,0.,40.));
#31598=CARTESIAN_POINT('',(18.,12.,40.));
#31599=CARTESIAN_POINT('',(18.,-6.,40.));
#31600=CARTESIAN_POINT('',(9.,12.,40.));
#31601=CARTESIAN_POINT('Origin',(90.,-18.,28.));
#31602=CARTESIAN_POINT('',(18.,-18.,12.));
#31603=CARTESIAN_POINT('Origin',(54.,0.,12.));
#31604=CARTESIAN_POINT('',(90.,18.,12.));
#31605=CARTESIAN_POINT('',(18.,18.,12.));
#31606=CARTESIAN_POINT('',(18.,18.,12.));
#31607=CARTESIAN_POINT('Origin',(18.,18.,28.));
#31608=CARTESIAN_POINT('',(90.,18.,28.));
#31609=CARTESIAN_POINT('Origin',(-54.,0.,12.));
#31610=CARTESIAN_POINT('',(-18.,-18.,12.));
#31611=CARTESIAN_POINT('',(-18.,-18.,12.));
#31612=CARTESIAN_POINT('',(-18.,18.,12.));
#31613=CARTESIAN_POINT('Origin',(-54.,0.,28.));
#31614=CARTESIAN_POINT('',(-18.,18.,28.));
#31615=CARTESIAN_POINT('',(-18.,12.,28.));
#31616=CARTESIAN_POINT('',(-18.,-18.,28.));
#31617=CARTESIAN_POINT('',(-18.,12.,28.));
#31618=CARTESIAN_POINT('Origin',(-90.,18.,28.));
#31619=CARTESIAN_POINT('Origin',(54.,0.,28.));
#31620=CARTESIAN_POINT('',(18.,12.,28.));
#31621=CARTESIAN_POINT('',(90.,12.,28.));
#31622=CARTESIAN_POINT('',(18.,18.,28.));
#31623=CARTESIAN_POINT('Origin',(-18.,12.,40.));
#31624=CARTESIAN_POINT('Origin',(-18.,12.,40.));
#31625=CARTESIAN_POINT('',(-18.,12.,40.));
#31626=CARTESIAN_POINT('Origin',(-90.,12.,40.));
#31627=CARTESIAN_POINT('Origin',(18.,-12.,40.));
#31628=CARTESIAN_POINT('Origin',(18.,12.,40.));
#31629=CARTESIAN_POINT('',(18.,12.,40.));
#31630=CARTESIAN_POINT('Origin',(18.,-12.,40.));
#31631=CARTESIAN_POINT('Origin',(0.,0.,2.));
#31632=CARTESIAN_POINT('',(40.,4.89858719658941E-15,0.));
#31633=CARTESIAN_POINT('Origin',(0.,0.,0.));
#31634=CARTESIAN_POINT('',(40.,4.89858719658941E-15,4.));
#31635=CARTESIAN_POINT('',(40.,4.89858719658941E-15,2.));
#31636=CARTESIAN_POINT('Origin',(0.,0.,4.));
#31637=CARTESIAN_POINT('Origin',(0.,0.,4.));
#31638=CARTESIAN_POINT('Origin',(0.,0.,0.));
#69467=UNCERTAINTY_MEASURE_WITH_UNIT(LENGTH_MEASURE(0.01),#69492,
'DISTANCE_ACCURACY_VALUE',
'Maximum model space distance between geometric entities at asserted c
onnectivities');
#69478=UNCERTAINTY_MEASURE_WITH_UNIT(LENGTH_MEASURE(0.01),#69492,
'DISTANCE_ACCURACY_VALUE',
'Maximum model space distance between geometric entities at asserted c
onnectivities');
#69480=(
GEOMETRIC_REPRESENTATION_CONTEXT(3)
GLOBAL_UNCERTAINTY_ASSIGNED_CONTEXT((#69467))
GLOBAL_UNIT_ASSIGNED_CONTEXT((#69492,#69494,#69495))
REPRESENTATION_CONTEXT('','3D')
);
#69491=(
GEOMETRIC_REPRESENTATION_CONTEXT(3)
GLOBAL_UNCERTAINTY_ASSIGNED_CONTEXT((#69478))
GLOBAL_UNIT_ASSIGNED_CONTEXT((#69492,#69494,#69495))
REPRESENTATION_CONTEXT('','3D')
);
#69492=(
LENGTH_UNIT()
NAMED_UNIT(*)
SI_UNIT(.MILLI.,.METRE.)
);
#69494=(
NAMED_UNIT(*)
PLANE_ANGLE_UNIT()
SI_UNIT($,.RADIAN.)
);
#69495=(
NAMED_UNIT(*)
SI_UNIT($,.STERADIAN.)
SOLID_ANGLE_UNIT()
);
#69497=SHAPE_DEFINITION_REPRESENTATION(#69509,#69571);
#69509=PRODUCT_DEFINITION_SHAPE('',$,#69584);
#69571=SHAPE_REPRESENTATION('',(#14865),#69480);
#69582=PRODUCT_DEFINITION_CONTEXT('part definition',#69620,'design');
#69584=PRODUCT_DEFINITION('Chuck body','Chuck body',#69596,#69582);
#69596=PRODUCT_DEFINITION_FORMATION('',$,#69623);
#69620=APPLICATION_CONTEXT(
'Core Data for Automotive Mechanical Design Process');
#69621=PRODUCT_CONTEXT('part definition',#69620,'mechanical');
#69623=PRODUCT('Chuck body','Chuck body',$,(#69621));
#69635=PRESENTATION_STYLE_ASSIGNMENT((#69645));
#69645=SURFACE_STYLE_USAGE(.BOTH.,#69655);
#69655=SURFACE_SIDE_STYLE('',(#69665));
#69665=SURFACE_STYLE_FILL_AREA(#69675);
#69675=FILL_AREA_STYLE('Dark blue',(#69685));
#69685=FILL_AREA_STYLE_COLOUR('Dark blue',#69695);
#69695=COLOUR_RGB('Dark blue',0.0901960784313725,0.270588235294118,0.513725490196078);
ENDSEC;
END-ISO-10303-21;
